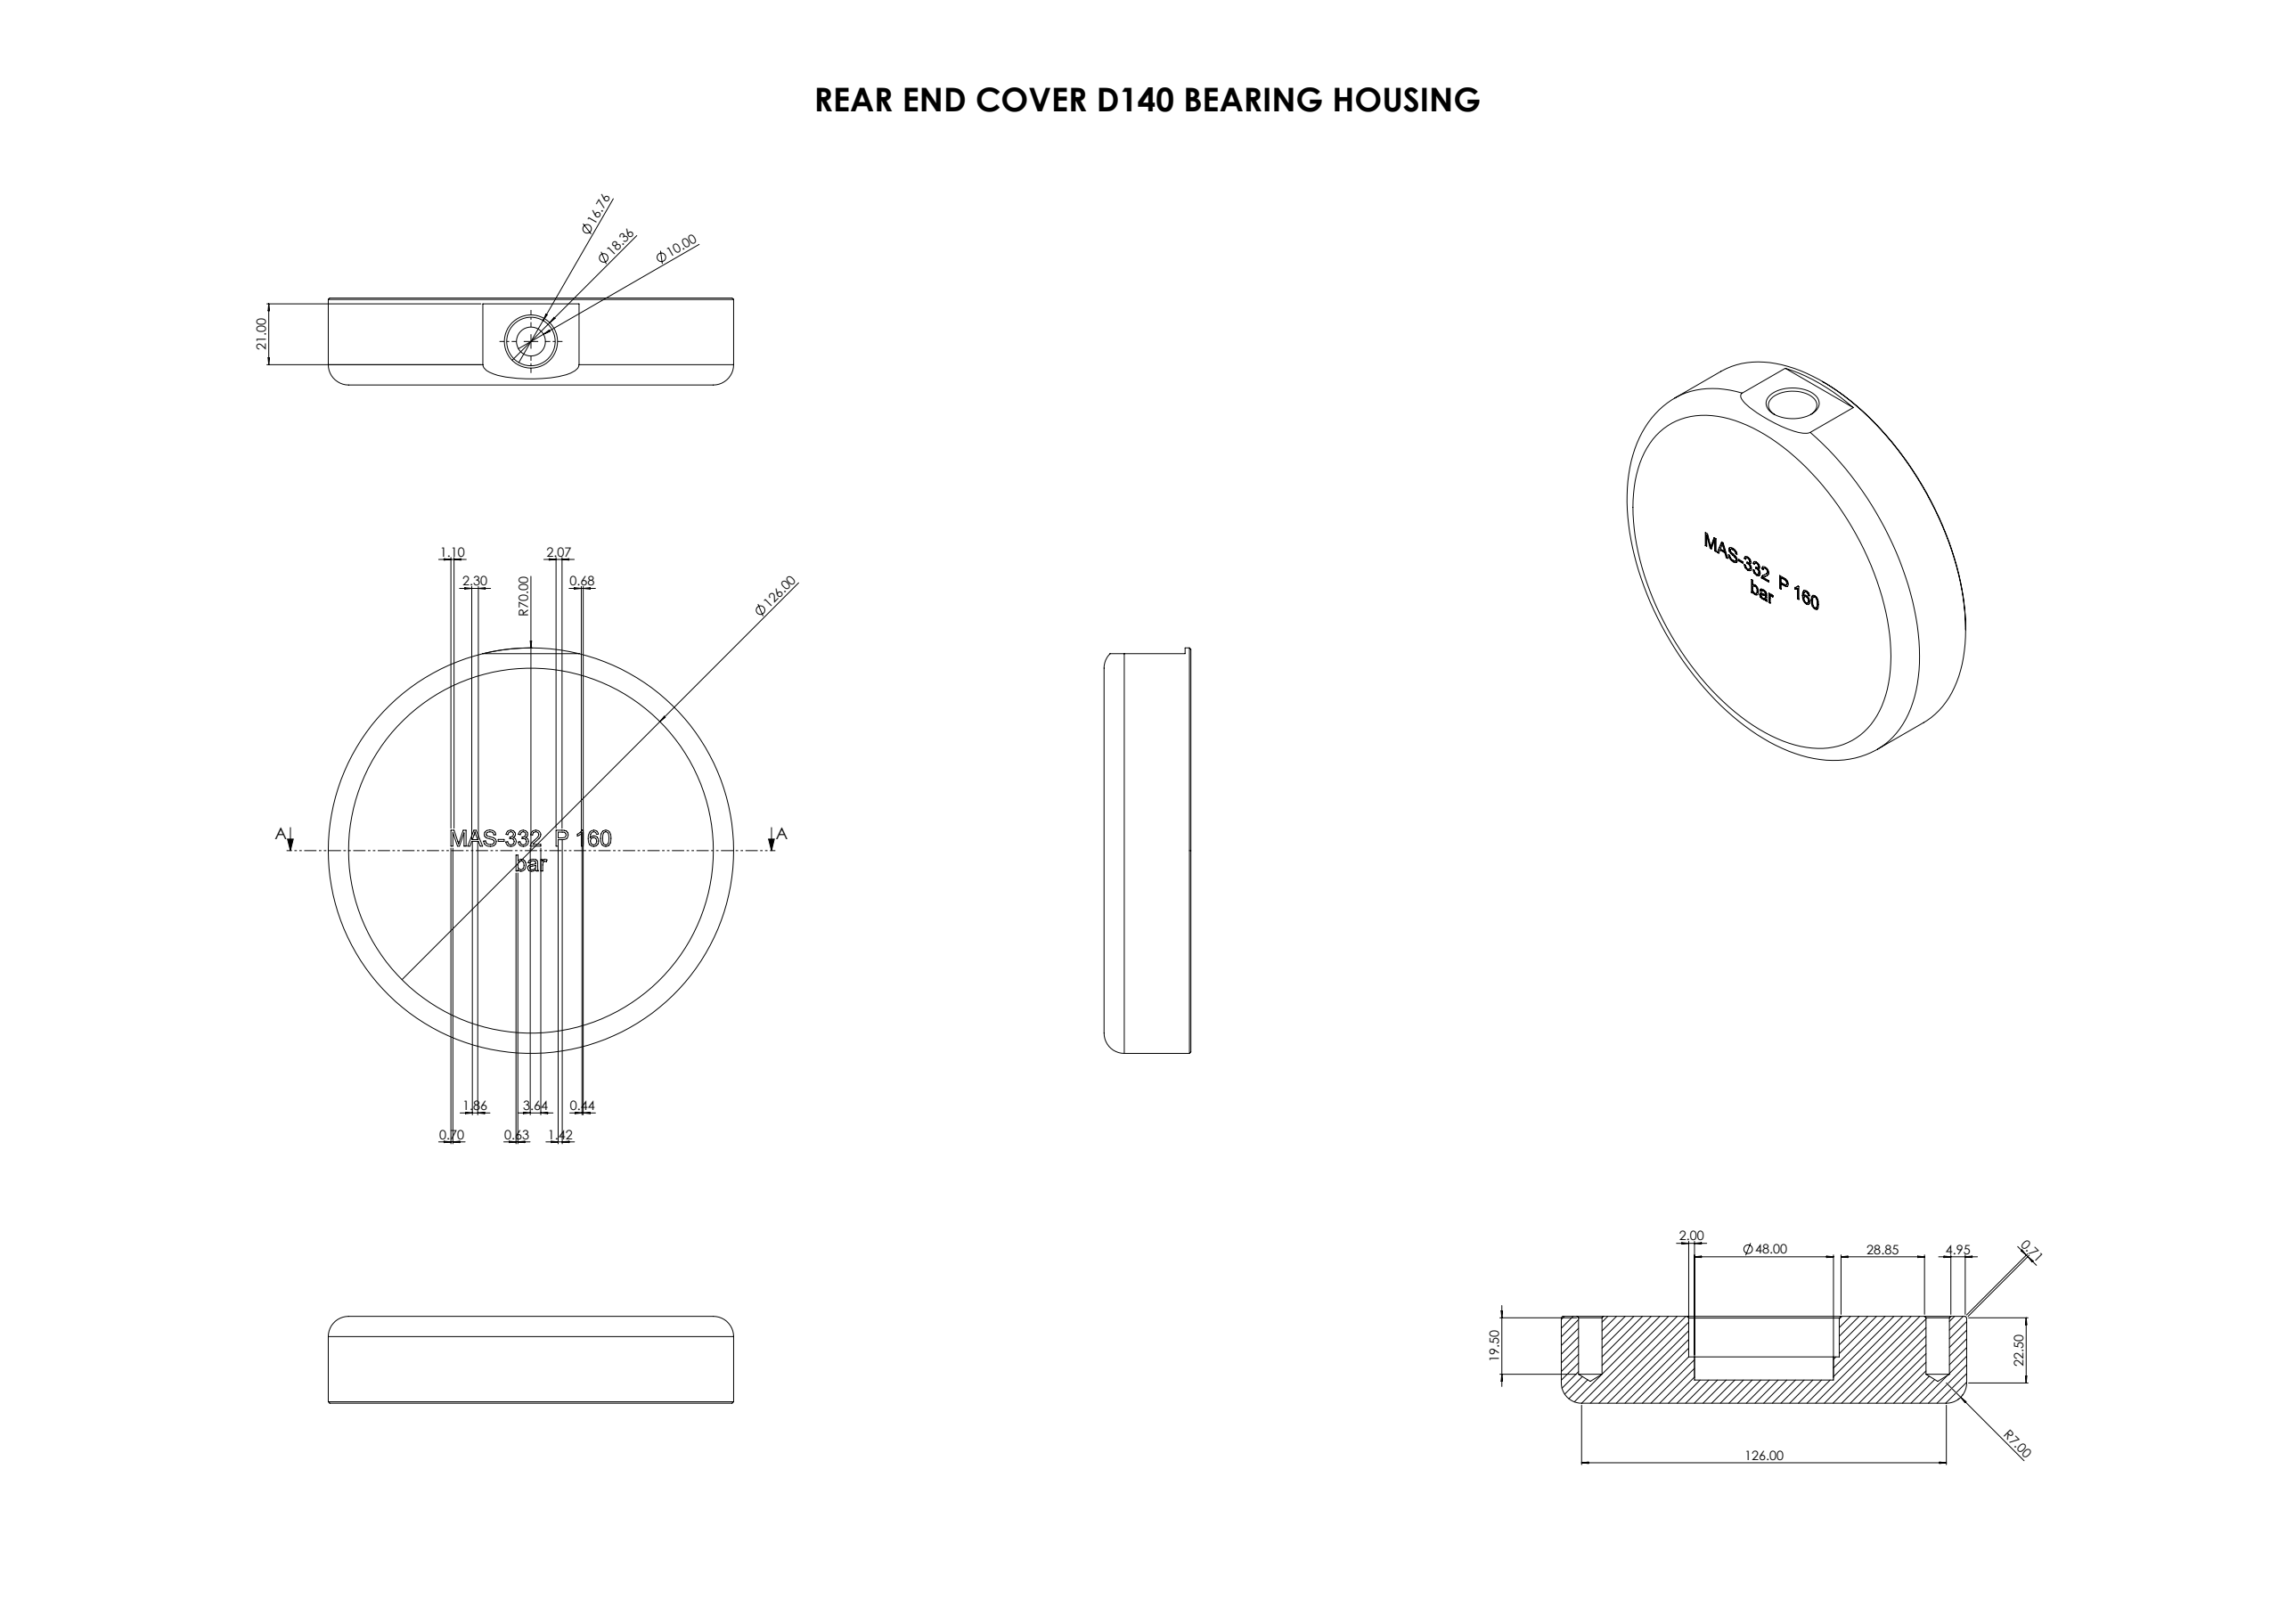
ISO-10303-21;
HEADER;
/* Generated by software containing ST-Developer
 * from STEP Tools, Inc. (www.steptools.com) 
 */

FILE_DESCRIPTION(
/* description */ (''),
/* implementation_level */ '2;1');

FILE_NAME(
/* name */ '03_Rear_End_Cover_D140_Bearing_Housing.step',
/* time_stamp */ '2026-10-23T00:52:27+05:00',
/* author */ (''),
/* organization */ (''),
/* preprocessor_version */ 'ST-DEVELOPER v20.2',
/* originating_system */ 'Autodesk Translation Framework v15.15.0.0',
/* authorisation */ '');

FILE_SCHEMA (('AUTOMOTIVE_DESIGN { 1 0 10303 214 3 1 1 }'));
ENDSEC;

DATA;
#10=MECHANICAL_DESIGN_GEOMETRIC_PRESENTATION_REPRESENTATION('',(#1566,#1567),#59204);
#312=TOROIDAL_SURFACE('',#24105,6.3,0.7);
#332=B_SPLINE_SURFACE_WITH_KNOTS('',2,1,((#43216,#43217),(#43218,#43219),
(#43220,#43221)),.UNSPECIFIED.,.F.,.F.,.F.,(3,3),(2,2),(0.,1.),(0.,0.0300000000000002),
 .UNSPECIFIED.);
#333=B_SPLINE_SURFACE_WITH_KNOTS('',2,1,((#43234,#43235),(#43236,#43237),
(#43238,#43239)),.UNSPECIFIED.,.F.,.F.,.F.,(3,3),(2,2),(0.,1.),(0.,0.0300000000000002),
 .UNSPECIFIED.);
#334=B_SPLINE_SURFACE_WITH_KNOTS('',2,1,((#43249,#43250),(#43251,#43252),
(#43253,#43254)),.UNSPECIFIED.,.F.,.F.,.F.,(3,3),(2,2),(0.,1.),(0.,0.0300000000000002),
 .UNSPECIFIED.);
#335=B_SPLINE_SURFACE_WITH_KNOTS('',2,1,((#43264,#43265),(#43266,#43267),
(#43268,#43269)),.UNSPECIFIED.,.F.,.F.,.F.,(3,3),(2,2),(0.,1.),(0.,0.0300000000000002),
 .UNSPECIFIED.);
#336=B_SPLINE_SURFACE_WITH_KNOTS('',2,1,((#43279,#43280),(#43281,#43282),
(#43283,#43284)),.UNSPECIFIED.,.F.,.F.,.F.,(3,3),(2,2),(0.,1.),(0.,0.0300000000000002),
 .UNSPECIFIED.);
#337=B_SPLINE_SURFACE_WITH_KNOTS('',2,1,((#43294,#43295),(#43296,#43297),
(#43298,#43299)),.UNSPECIFIED.,.F.,.F.,.F.,(3,3),(2,2),(0.,1.),(0.,0.0300000000000002),
 .UNSPECIFIED.);
#338=B_SPLINE_SURFACE_WITH_KNOTS('',2,1,((#43309,#43310),(#43311,#43312),
(#43313,#43314)),.UNSPECIFIED.,.F.,.F.,.F.,(3,3),(2,2),(0.,1.),(0.,0.0300000000000002),
 .UNSPECIFIED.);
#339=B_SPLINE_SURFACE_WITH_KNOTS('',2,1,((#43324,#43325),(#43326,#43327),
(#43328,#43329)),.UNSPECIFIED.,.F.,.F.,.F.,(3,3),(2,2),(0.,1.),(0.,0.0300000000000002),
 .UNSPECIFIED.);
#340=B_SPLINE_SURFACE_WITH_KNOTS('',2,1,((#43339,#43340),(#43341,#43342),
(#43343,#43344)),.UNSPECIFIED.,.F.,.F.,.F.,(3,3),(2,2),(0.,1.),(0.,0.0300000000000002),
 .UNSPECIFIED.);
#341=B_SPLINE_SURFACE_WITH_KNOTS('',2,1,((#43357,#43358),(#43359,#43360),
(#43361,#43362)),.UNSPECIFIED.,.F.,.F.,.F.,(3,3),(2,2),(0.,1.),(0.,0.0300000000000002),
 .UNSPECIFIED.);
#342=B_SPLINE_SURFACE_WITH_KNOTS('',2,1,((#43375,#43376),(#43377,#43378),
(#43379,#43380)),.UNSPECIFIED.,.F.,.F.,.F.,(3,3),(2,2),(0.,1.),(0.,0.0300000000000002),
 .UNSPECIFIED.);
#343=B_SPLINE_SURFACE_WITH_KNOTS('',2,1,((#43396,#43397),(#43398,#43399),
(#43400,#43401)),.UNSPECIFIED.,.F.,.F.,.F.,(3,3),(2,2),(0.,1.),(0.,0.0300000000000002),
 .UNSPECIFIED.);
#344=B_SPLINE_SURFACE_WITH_KNOTS('',2,1,((#43411,#43412),(#43413,#43414),
(#43415,#43416)),.UNSPECIFIED.,.F.,.F.,.F.,(3,3),(2,2),(0.,1.),(0.,0.0300000000000002),
 .UNSPECIFIED.);
#345=B_SPLINE_SURFACE_WITH_KNOTS('',2,1,((#43426,#43427),(#43428,#43429),
(#43430,#43431)),.UNSPECIFIED.,.F.,.F.,.F.,(3,3),(2,2),(0.,1.),(0.,0.0300000000000002),
 .UNSPECIFIED.);
#346=B_SPLINE_SURFACE_WITH_KNOTS('',2,1,((#43441,#43442),(#43443,#43444),
(#43445,#43446)),.UNSPECIFIED.,.F.,.F.,.F.,(3,3),(2,2),(0.,1.),(0.,0.0300000000000002),
 .UNSPECIFIED.);
#347=B_SPLINE_SURFACE_WITH_KNOTS('',2,1,((#43456,#43457),(#43458,#43459),
(#43460,#43461)),.UNSPECIFIED.,.F.,.F.,.F.,(3,3),(2,2),(0.,1.),(0.,0.0300000000000002),
 .UNSPECIFIED.);
#348=B_SPLINE_SURFACE_WITH_KNOTS('',2,1,((#43471,#43472),(#43473,#43474),
(#43475,#43476)),.UNSPECIFIED.,.F.,.F.,.F.,(3,3),(2,2),(0.,1.),(0.,0.0300000000000002),
 .UNSPECIFIED.);
#349=B_SPLINE_SURFACE_WITH_KNOTS('',2,1,((#43486,#43487),(#43488,#43489),
(#43490,#43491)),.UNSPECIFIED.,.F.,.F.,.F.,(3,3),(2,2),(0.,1.),(0.,0.0300000000000002),
 .UNSPECIFIED.);
#350=B_SPLINE_SURFACE_WITH_KNOTS('',2,1,((#43507,#43508),(#43509,#43510),
(#43511,#43512)),.UNSPECIFIED.,.F.,.F.,.F.,(3,3),(2,2),(0.,1.),(0.,0.0300000000000002),
 .UNSPECIFIED.);
#351=B_SPLINE_SURFACE_WITH_KNOTS('',2,1,((#43522,#43523),(#43524,#43525),
(#43526,#43527)),.UNSPECIFIED.,.F.,.F.,.F.,(3,3),(2,2),(0.,1.),(0.,0.0300000000000002),
 .UNSPECIFIED.);
#352=B_SPLINE_SURFACE_WITH_KNOTS('',2,1,((#43537,#43538),(#43539,#43540),
(#43541,#43542)),.UNSPECIFIED.,.F.,.F.,.F.,(3,3),(2,2),(0.,1.),(0.,0.0300000000000002),
 .UNSPECIFIED.);
#353=B_SPLINE_SURFACE_WITH_KNOTS('',2,1,((#43552,#43553),(#43554,#43555),
(#43556,#43557)),.UNSPECIFIED.,.F.,.F.,.F.,(3,3),(2,2),(0.,1.),(0.,0.0300000000000002),
 .UNSPECIFIED.);
#354=B_SPLINE_SURFACE_WITH_KNOTS('',2,1,((#43567,#43568),(#43569,#43570),
(#43571,#43572)),.UNSPECIFIED.,.F.,.F.,.F.,(3,3),(2,2),(0.,1.),(0.,0.0300000000000002),
 .UNSPECIFIED.);
#355=B_SPLINE_SURFACE_WITH_KNOTS('',2,1,((#43582,#43583),(#43584,#43585),
(#43586,#43587)),.UNSPECIFIED.,.F.,.F.,.F.,(3,3),(2,2),(0.,1.),(0.,0.0300000000000002),
 .UNSPECIFIED.);
#356=B_SPLINE_SURFACE_WITH_KNOTS('',2,1,((#43597,#43598),(#43599,#43600),
(#43601,#43602)),.UNSPECIFIED.,.F.,.F.,.F.,(3,3),(2,2),(0.,1.),(0.,0.0300000000000002),
 .UNSPECIFIED.);
#357=B_SPLINE_SURFACE_WITH_KNOTS('',2,1,((#43612,#43613),(#43614,#43615),
(#43616,#43617)),.UNSPECIFIED.,.F.,.F.,.F.,(3,3),(2,2),(0.,1.),(0.,0.0300000000000002),
 .UNSPECIFIED.);
#358=B_SPLINE_SURFACE_WITH_KNOTS('',2,1,((#43627,#43628),(#43629,#43630),
(#43631,#43632)),.UNSPECIFIED.,.F.,.F.,.F.,(3,3),(2,2),(0.,1.),(0.,0.0300000000000002),
 .UNSPECIFIED.);
#359=B_SPLINE_SURFACE_WITH_KNOTS('',2,1,((#43642,#43643),(#43644,#43645),
(#43646,#43647)),.UNSPECIFIED.,.F.,.F.,.F.,(3,3),(2,2),(0.,1.),(0.,0.0300000000000002),
 .UNSPECIFIED.);
#360=B_SPLINE_SURFACE_WITH_KNOTS('',2,1,((#43657,#43658),(#43659,#43660),
(#43661,#43662)),.UNSPECIFIED.,.F.,.F.,.F.,(3,3),(2,2),(0.,1.),(0.,0.0300000000000002),
 .UNSPECIFIED.);
#361=B_SPLINE_SURFACE_WITH_KNOTS('',2,1,((#43672,#43673),(#43674,#43675),
(#43676,#43677)),.UNSPECIFIED.,.F.,.F.,.F.,(3,3),(2,2),(0.,1.),(0.,0.0300000000000002),
 .UNSPECIFIED.);
#362=B_SPLINE_SURFACE_WITH_KNOTS('',2,1,((#43687,#43688),(#43689,#43690),
(#43691,#43692)),.UNSPECIFIED.,.F.,.F.,.F.,(3,3),(2,2),(0.,1.),(0.,0.0300000000000002),
 .UNSPECIFIED.);
#363=B_SPLINE_SURFACE_WITH_KNOTS('',2,1,((#43702,#43703),(#43704,#43705),
(#43706,#43707)),.UNSPECIFIED.,.F.,.F.,.F.,(3,3),(2,2),(0.,1.),(0.,0.0300000000000002),
 .UNSPECIFIED.);
#364=B_SPLINE_SURFACE_WITH_KNOTS('',2,1,((#43717,#43718),(#43719,#43720),
(#43721,#43722)),.UNSPECIFIED.,.F.,.F.,.F.,(3,3),(2,2),(0.,1.),(0.,0.0300000000000002),
 .UNSPECIFIED.);
#365=B_SPLINE_SURFACE_WITH_KNOTS('',2,1,((#43736,#43737),(#43738,#43739),
(#43740,#43741)),.UNSPECIFIED.,.F.,.F.,.F.,(3,3),(2,2),(0.,1.),(0.,0.0300000000000002),
 .UNSPECIFIED.);
#366=B_SPLINE_SURFACE_WITH_KNOTS('',2,1,((#43754,#43755),(#43756,#43757),
(#43758,#43759)),.UNSPECIFIED.,.F.,.F.,.F.,(3,3),(2,2),(0.,1.),(0.,0.0300000000000002),
 .UNSPECIFIED.);
#367=B_SPLINE_SURFACE_WITH_KNOTS('',2,1,((#43769,#43770),(#43771,#43772),
(#43773,#43774)),.UNSPECIFIED.,.F.,.F.,.F.,(3,3),(2,2),(0.,1.),(0.,0.0300000000000002),
 .UNSPECIFIED.);
#368=B_SPLINE_SURFACE_WITH_KNOTS('',2,1,((#43784,#43785),(#43786,#43787),
(#43788,#43789)),.UNSPECIFIED.,.F.,.F.,.F.,(3,3),(2,2),(0.,1.),(0.,0.0300000000000002),
 .UNSPECIFIED.);
#369=B_SPLINE_SURFACE_WITH_KNOTS('',2,1,((#43799,#43800),(#43801,#43802),
(#43803,#43804)),.UNSPECIFIED.,.F.,.F.,.F.,(3,3),(2,2),(0.,1.),(0.,0.0300000000000002),
 .UNSPECIFIED.);
#370=B_SPLINE_SURFACE_WITH_KNOTS('',2,1,((#43814,#43815),(#43816,#43817),
(#43818,#43819)),.UNSPECIFIED.,.F.,.F.,.F.,(3,3),(2,2),(0.,1.),(0.,0.0300000000000002),
 .UNSPECIFIED.);
#371=B_SPLINE_SURFACE_WITH_KNOTS('',2,1,((#43829,#43830),(#43831,#43832),
(#43833,#43834)),.UNSPECIFIED.,.F.,.F.,.F.,(3,3),(2,2),(0.,1.),(0.,0.0300000000000002),
 .UNSPECIFIED.);
#372=B_SPLINE_SURFACE_WITH_KNOTS('',2,1,((#43844,#43845),(#43846,#43847),
(#43848,#43849)),.UNSPECIFIED.,.F.,.F.,.F.,(3,3),(2,2),(0.,1.),(0.,0.0300000000000002),
 .UNSPECIFIED.);
#373=B_SPLINE_SURFACE_WITH_KNOTS('',2,1,((#43856,#43857),(#43858,#43859),
(#43860,#43861)),.UNSPECIFIED.,.F.,.F.,.F.,(3,3),(2,2),(0.,1.),(0.,0.0300000000000002),
 .UNSPECIFIED.);
#374=B_SPLINE_SURFACE_WITH_KNOTS('',2,1,((#43874,#43875),(#43876,#43877),
(#43878,#43879)),.UNSPECIFIED.,.F.,.F.,.F.,(3,3),(2,2),(0.,1.),(0.,0.0300000000000002),
 .UNSPECIFIED.);
#375=B_SPLINE_SURFACE_WITH_KNOTS('',2,1,((#43889,#43890),(#43891,#43892),
(#43893,#43894)),.UNSPECIFIED.,.F.,.F.,.F.,(3,3),(2,2),(0.,1.),(0.,0.0300000000000002),
 .UNSPECIFIED.);
#376=B_SPLINE_SURFACE_WITH_KNOTS('',2,1,((#43904,#43905),(#43906,#43907),
(#43908,#43909)),.UNSPECIFIED.,.F.,.F.,.F.,(3,3),(2,2),(0.,1.),(0.,0.0300000000000002),
 .UNSPECIFIED.);
#377=B_SPLINE_SURFACE_WITH_KNOTS('',2,1,((#43919,#43920),(#43921,#43922),
(#43923,#43924)),.UNSPECIFIED.,.F.,.F.,.F.,(3,3),(2,2),(0.,1.),(0.,0.0300000000000002),
 .UNSPECIFIED.);
#378=B_SPLINE_SURFACE_WITH_KNOTS('',2,1,((#43934,#43935),(#43936,#43937),
(#43938,#43939)),.UNSPECIFIED.,.F.,.F.,.F.,(3,3),(2,2),(0.,1.),(0.,0.0300000000000002),
 .UNSPECIFIED.);
#379=B_SPLINE_SURFACE_WITH_KNOTS('',2,1,((#43949,#43950),(#43951,#43952),
(#43953,#43954)),.UNSPECIFIED.,.F.,.F.,.F.,(3,3),(2,2),(0.,1.),(0.,0.0300000000000002),
 .UNSPECIFIED.);
#380=B_SPLINE_SURFACE_WITH_KNOTS('',2,1,((#43964,#43965),(#43966,#43967),
(#43968,#43969)),.UNSPECIFIED.,.F.,.F.,.F.,(3,3),(2,2),(0.,1.),(0.,0.0300000000000002),
 .UNSPECIFIED.);
#381=B_SPLINE_SURFACE_WITH_KNOTS('',2,1,((#43979,#43980),(#43981,#43982),
(#43983,#43984)),.UNSPECIFIED.,.F.,.F.,.F.,(3,3),(2,2),(0.,1.),(0.,0.0300000000000002),
 .UNSPECIFIED.);
#382=B_SPLINE_SURFACE_WITH_KNOTS('',2,1,((#43994,#43995),(#43996,#43997),
(#43998,#43999)),.UNSPECIFIED.,.F.,.F.,.F.,(3,3),(2,2),(0.,1.),(0.,0.0300000000000002),
 .UNSPECIFIED.);
#383=B_SPLINE_SURFACE_WITH_KNOTS('',2,1,((#44009,#44010),(#44011,#44012),
(#44013,#44014)),.UNSPECIFIED.,.F.,.F.,.F.,(3,3),(2,2),(0.,1.),(0.,0.0300000000000002),
 .UNSPECIFIED.);
#384=B_SPLINE_SURFACE_WITH_KNOTS('',2,1,((#44024,#44025),(#44026,#44027),
(#44028,#44029)),.UNSPECIFIED.,.F.,.F.,.F.,(3,3),(2,2),(0.,1.),(0.,0.0300000000000002),
 .UNSPECIFIED.);
#385=B_SPLINE_SURFACE_WITH_KNOTS('',2,1,((#44037,#44038),(#44039,#44040),
(#44041,#44042)),.UNSPECIFIED.,.F.,.F.,.F.,(3,3),(2,2),(0.,1.),(0.,0.0300000000000002),
 .UNSPECIFIED.);
#386=B_SPLINE_SURFACE_WITH_KNOTS('',2,1,((#44055,#44056),(#44057,#44058),
(#44059,#44060)),.UNSPECIFIED.,.F.,.F.,.F.,(3,3),(2,2),(0.,1.),(0.,0.0300000000000002),
 .UNSPECIFIED.);
#387=B_SPLINE_SURFACE_WITH_KNOTS('',2,1,((#44076,#44077),(#44078,#44079),
(#44080,#44081)),.UNSPECIFIED.,.F.,.F.,.F.,(3,3),(2,2),(0.,1.),(0.,0.0300000000000002),
 .UNSPECIFIED.);
#388=B_SPLINE_SURFACE_WITH_KNOTS('',2,1,((#44091,#44092),(#44093,#44094),
(#44095,#44096)),.UNSPECIFIED.,.F.,.F.,.F.,(3,3),(2,2),(0.,1.),(0.,0.0300000000000002),
 .UNSPECIFIED.);
#389=B_SPLINE_SURFACE_WITH_KNOTS('',2,1,((#44179,#44180),(#44181,#44182),
(#44183,#44184)),.UNSPECIFIED.,.F.,.F.,.F.,(3,3),(2,2),(0.,1.),(0.,0.0300000000000002),
 .UNSPECIFIED.);
#390=B_SPLINE_SURFACE_WITH_KNOTS('',2,1,((#44194,#44195),(#44196,#44197),
(#44198,#44199)),.UNSPECIFIED.,.F.,.F.,.F.,(3,3),(2,2),(0.,1.),(0.,0.0300000000000002),
 .UNSPECIFIED.);
#391=B_SPLINE_SURFACE_WITH_KNOTS('',2,1,((#44237,#44238),(#44239,#44240),
(#44241,#44242)),.UNSPECIFIED.,.F.,.F.,.F.,(3,3),(2,2),(0.,1.),(0.,0.0300000000000002),
 .UNSPECIFIED.);
#392=B_SPLINE_SURFACE_WITH_KNOTS('',2,1,((#44255,#44256),(#44257,#44258),
(#44259,#44260)),.UNSPECIFIED.,.F.,.F.,.F.,(3,3),(2,2),(0.,1.),(0.,0.0300000000000002),
 .UNSPECIFIED.);
#393=B_SPLINE_SURFACE_WITH_KNOTS('',2,1,((#44270,#44271),(#44272,#44273),
(#44274,#44275)),.UNSPECIFIED.,.F.,.F.,.F.,(3,3),(2,2),(0.,1.),(0.,0.0300000000000002),
 .UNSPECIFIED.);
#394=B_SPLINE_SURFACE_WITH_KNOTS('',2,1,((#44285,#44286),(#44287,#44288),
(#44289,#44290)),.UNSPECIFIED.,.F.,.F.,.F.,(3,3),(2,2),(0.,1.),(0.,0.0300000000000002),
 .UNSPECIFIED.);
#395=B_SPLINE_SURFACE_WITH_KNOTS('',2,1,((#44300,#44301),(#44302,#44303),
(#44304,#44305)),.UNSPECIFIED.,.F.,.F.,.F.,(3,3),(2,2),(0.,1.),(0.,0.0300000000000002),
 .UNSPECIFIED.);
#396=B_SPLINE_SURFACE_WITH_KNOTS('',2,1,((#44315,#44316),(#44317,#44318),
(#44319,#44320)),.UNSPECIFIED.,.F.,.F.,.F.,(3,3),(2,2),(0.,1.),(0.,0.0300000000000002),
 .UNSPECIFIED.);
#397=B_SPLINE_SURFACE_WITH_KNOTS('',2,1,((#44330,#44331),(#44332,#44333),
(#44334,#44335)),.UNSPECIFIED.,.F.,.F.,.F.,(3,3),(2,2),(0.,1.),(0.,0.0300000000000002),
 .UNSPECIFIED.);
#398=B_SPLINE_SURFACE_WITH_KNOTS('',2,1,((#44345,#44346),(#44347,#44348),
(#44349,#44350)),.UNSPECIFIED.,.F.,.F.,.F.,(3,3),(2,2),(0.,1.),(0.,0.0300000000000002),
 .UNSPECIFIED.);
#399=B_SPLINE_SURFACE_WITH_KNOTS('',2,1,((#44360,#44361),(#44362,#44363),
(#44364,#44365)),.UNSPECIFIED.,.F.,.F.,.F.,(3,3),(2,2),(0.,1.),(0.,0.0300000000000002),
 .UNSPECIFIED.);
#400=B_SPLINE_SURFACE_WITH_KNOTS('',2,1,((#44375,#44376),(#44377,#44378),
(#44379,#44380)),.UNSPECIFIED.,.F.,.F.,.F.,(3,3),(2,2),(0.,1.),(0.,0.0300000000000002),
 .UNSPECIFIED.);
#401=B_SPLINE_SURFACE_WITH_KNOTS('',2,1,((#44390,#44391),(#44392,#44393),
(#44394,#44395)),.UNSPECIFIED.,.F.,.F.,.F.,(3,3),(2,2),(0.,1.),(0.,0.0300000000000002),
 .UNSPECIFIED.);
#402=B_SPLINE_SURFACE_WITH_KNOTS('',2,1,((#44411,#44412),(#44413,#44414),
(#44415,#44416)),.UNSPECIFIED.,.F.,.F.,.F.,(3,3),(2,2),(0.,1.),(0.,0.0300000000000002),
 .UNSPECIFIED.);
#403=B_SPLINE_SURFACE_WITH_KNOTS('',2,1,((#44426,#44427),(#44428,#44429),
(#44430,#44431)),.UNSPECIFIED.,.F.,.F.,.F.,(3,3),(2,2),(0.,1.),(0.,0.0300000000000002),
 .UNSPECIFIED.);
#404=B_SPLINE_SURFACE_WITH_KNOTS('',2,1,((#44441,#44442),(#44443,#44444),
(#44445,#44446)),.UNSPECIFIED.,.F.,.F.,.F.,(3,3),(2,2),(0.,1.),(0.,0.0300000000000002),
 .UNSPECIFIED.);
#405=B_SPLINE_SURFACE_WITH_KNOTS('',2,1,((#44456,#44457),(#44458,#44459),
(#44460,#44461)),.UNSPECIFIED.,.F.,.F.,.F.,(3,3),(2,2),(0.,1.),(0.,0.0300000000000002),
 .UNSPECIFIED.);
#406=B_SPLINE_SURFACE_WITH_KNOTS('',2,1,((#44471,#44472),(#44473,#44474),
(#44475,#44476)),.UNSPECIFIED.,.F.,.F.,.F.,(3,3),(2,2),(0.,1.),(0.,0.0300000000000002),
 .UNSPECIFIED.);
#407=B_SPLINE_SURFACE_WITH_KNOTS('',2,1,((#44486,#44487),(#44488,#44489),
(#44490,#44491)),.UNSPECIFIED.,.F.,.F.,.F.,(3,3),(2,2),(0.,1.),(0.,0.0300000000000002),
 .UNSPECIFIED.);
#408=B_SPLINE_SURFACE_WITH_KNOTS('',2,1,((#44501,#44502),(#44503,#44504),
(#44505,#44506)),.UNSPECIFIED.,.F.,.F.,.F.,(3,3),(2,2),(0.,1.),(0.,0.0300000000000002),
 .UNSPECIFIED.);
#409=B_SPLINE_SURFACE_WITH_KNOTS('',2,1,((#44522,#44523),(#44524,#44525),
(#44526,#44527)),.UNSPECIFIED.,.F.,.F.,.F.,(3,3),(2,2),(0.,1.),(0.,0.0300000000000002),
 .UNSPECIFIED.);
#410=B_SPLINE_SURFACE_WITH_KNOTS('',2,1,((#44537,#44538),(#44539,#44540),
(#44541,#44542)),.UNSPECIFIED.,.F.,.F.,.F.,(3,3),(2,2),(0.,1.),(0.,0.0300000000000002),
 .UNSPECIFIED.);
#411=B_SPLINE_SURFACE_WITH_KNOTS('',2,1,((#44552,#44553),(#44554,#44555),
(#44556,#44557)),.UNSPECIFIED.,.F.,.F.,.F.,(3,3),(2,2),(0.,1.),(0.,0.0300000000000002),
 .UNSPECIFIED.);
#412=B_SPLINE_SURFACE_WITH_KNOTS('',2,1,((#44567,#44568),(#44569,#44570),
(#44571,#44572)),.UNSPECIFIED.,.F.,.F.,.F.,(3,3),(2,2),(0.,1.),(0.,0.0300000000000002),
 .UNSPECIFIED.);
#413=B_SPLINE_SURFACE_WITH_KNOTS('',2,1,((#44582,#44583),(#44584,#44585),
(#44586,#44587)),.UNSPECIFIED.,.F.,.F.,.F.,(3,3),(2,2),(0.,1.),(0.,0.0300000000000002),
 .UNSPECIFIED.);
#414=B_SPLINE_SURFACE_WITH_KNOTS('',2,1,((#44597,#44598),(#44599,#44600),
(#44601,#44602)),.UNSPECIFIED.,.F.,.F.,.F.,(3,3),(2,2),(0.,1.),(0.,0.0300000000000002),
 .UNSPECIFIED.);
#415=B_SPLINE_SURFACE_WITH_KNOTS('',2,1,((#44612,#44613),(#44614,#44615),
(#44616,#44617)),.UNSPECIFIED.,.F.,.F.,.F.,(3,3),(2,2),(0.,1.),(0.,0.0300000000000002),
 .UNSPECIFIED.);
#416=B_SPLINE_SURFACE_WITH_KNOTS('',2,1,((#44633,#44634),(#44635,#44636),
(#44637,#44638)),.UNSPECIFIED.,.F.,.F.,.F.,(3,3),(2,2),(0.,1.),(0.,0.0300000000000002),
 .UNSPECIFIED.);
#417=B_SPLINE_SURFACE_WITH_KNOTS('',2,1,((#44648,#44649),(#44650,#44651),
(#44652,#44653)),.UNSPECIFIED.,.F.,.F.,.F.,(3,3),(2,2),(0.,1.),(0.,0.0300000000000002),
 .UNSPECIFIED.);
#418=B_SPLINE_SURFACE_WITH_KNOTS('',2,1,((#44686,#44687),(#44688,#44689),
(#44690,#44691)),.UNSPECIFIED.,.F.,.F.,.F.,(3,3),(2,2),(0.,1.),(0.,0.0300000000000002),
 .UNSPECIFIED.);
#419=B_SPLINE_SURFACE_WITH_KNOTS('',2,1,((#44704,#44705),(#44706,#44707),
(#44708,#44709)),.UNSPECIFIED.,.F.,.F.,.F.,(3,3),(2,2),(0.,1.),(0.,0.0300000000000002),
 .UNSPECIFIED.);
#420=B_SPLINE_SURFACE_WITH_KNOTS('',2,1,((#44783,#44784),(#44785,#44786),
(#44787,#44788)),.UNSPECIFIED.,.F.,.F.,.F.,(3,3),(2,2),(0.,1.),(0.,0.0300000000000002),
 .UNSPECIFIED.);
#421=B_SPLINE_SURFACE_WITH_KNOTS('',2,1,((#44801,#44802),(#44803,#44804),
(#44805,#44806)),.UNSPECIFIED.,.F.,.F.,.F.,(3,3),(2,2),(0.,1.),(0.,0.0300000000000002),
 .UNSPECIFIED.);
#422=B_SPLINE_SURFACE_WITH_KNOTS('',2,1,((#44816,#44817),(#44818,#44819),
(#44820,#44821)),.UNSPECIFIED.,.F.,.F.,.F.,(3,3),(2,2),(0.,1.),(0.,0.0300000000000002),
 .UNSPECIFIED.);
#423=B_SPLINE_SURFACE_WITH_KNOTS('',2,1,((#44831,#44832),(#44833,#44834),
(#44835,#44836)),.UNSPECIFIED.,.F.,.F.,.F.,(3,3),(2,2),(0.,1.),(0.,0.0300000000000002),
 .UNSPECIFIED.);
#424=B_SPLINE_SURFACE_WITH_KNOTS('',2,1,((#44846,#44847),(#44848,#44849),
(#44850,#44851)),.UNSPECIFIED.,.F.,.F.,.F.,(3,3),(2,2),(0.,1.),(0.,0.0300000000000002),
 .UNSPECIFIED.);
#425=B_SPLINE_SURFACE_WITH_KNOTS('',2,1,((#44861,#44862),(#44863,#44864),
(#44865,#44866)),.UNSPECIFIED.,.F.,.F.,.F.,(3,3),(2,2),(0.,1.),(0.,0.0300000000000002),
 .UNSPECIFIED.);
#426=B_SPLINE_SURFACE_WITH_KNOTS('',2,1,((#44876,#44877),(#44878,#44879),
(#44880,#44881)),.UNSPECIFIED.,.F.,.F.,.F.,(3,3),(2,2),(0.,1.),(0.,0.0300000000000002),
 .UNSPECIFIED.);
#427=B_SPLINE_SURFACE_WITH_KNOTS('',2,1,((#44891,#44892),(#44893,#44894),
(#44895,#44896)),.UNSPECIFIED.,.F.,.F.,.F.,(3,3),(2,2),(0.,1.),(0.,0.0300000000000002),
 .UNSPECIFIED.);
#428=B_SPLINE_SURFACE_WITH_KNOTS('',2,1,((#44906,#44907),(#44908,#44909),
(#44910,#44911)),.UNSPECIFIED.,.F.,.F.,.F.,(3,3),(2,2),(0.,1.),(0.,0.0300000000000002),
 .UNSPECIFIED.);
#429=B_SPLINE_SURFACE_WITH_KNOTS('',2,1,((#44921,#44922),(#44923,#44924),
(#44925,#44926)),.UNSPECIFIED.,.F.,.F.,.F.,(3,3),(2,2),(0.,1.),(0.,0.0300000000000002),
 .UNSPECIFIED.);
#430=B_SPLINE_SURFACE_WITH_KNOTS('',2,1,((#44936,#44937),(#44938,#44939),
(#44940,#44941)),.UNSPECIFIED.,.F.,.F.,.F.,(3,3),(2,2),(0.,1.),(0.,0.0300000000000002),
 .UNSPECIFIED.);
#431=B_SPLINE_SURFACE_WITH_KNOTS('',2,1,((#44951,#44952),(#44953,#44954),
(#44955,#44956)),.UNSPECIFIED.,.F.,.F.,.F.,(3,3),(2,2),(0.,1.),(0.,0.0300000000000002),
 .UNSPECIFIED.);
#432=B_SPLINE_SURFACE_WITH_KNOTS('',2,1,((#44966,#44967),(#44968,#44969),
(#44970,#44971)),.UNSPECIFIED.,.F.,.F.,.F.,(3,3),(2,2),(0.,1.),(0.,0.0300000000000002),
 .UNSPECIFIED.);
#433=B_SPLINE_SURFACE_WITH_KNOTS('',2,1,((#44987,#44988),(#44989,#44990),
(#44991,#44992)),.UNSPECIFIED.,.F.,.F.,.F.,(3,3),(2,2),(0.,1.),(0.,0.0300000000000002),
 .UNSPECIFIED.);
#434=B_SPLINE_SURFACE_WITH_KNOTS('',2,1,((#45002,#45003),(#45004,#45005),
(#45006,#45007)),.UNSPECIFIED.,.F.,.F.,.F.,(3,3),(2,2),(0.,1.),(0.,0.0300000000000002),
 .UNSPECIFIED.);
#435=B_SPLINE_SURFACE_WITH_KNOTS('',2,1,((#45017,#45018),(#45019,#45020),
(#45021,#45022)),.UNSPECIFIED.,.F.,.F.,.F.,(3,3),(2,2),(0.,1.),(0.,0.0300000000000002),
 .UNSPECIFIED.);
#436=B_SPLINE_SURFACE_WITH_KNOTS('',2,1,((#45032,#45033),(#45034,#45035),
(#45036,#45037)),.UNSPECIFIED.,.F.,.F.,.F.,(3,3),(2,2),(0.,1.),(0.,0.0300000000000002),
 .UNSPECIFIED.);
#437=B_SPLINE_SURFACE_WITH_KNOTS('',2,1,((#45047,#45048),(#45049,#45050),
(#45051,#45052)),.UNSPECIFIED.,.F.,.F.,.F.,(3,3),(2,2),(0.,1.),(0.,0.0300000000000002),
 .UNSPECIFIED.);
#438=B_SPLINE_SURFACE_WITH_KNOTS('',2,1,((#45062,#45063),(#45064,#45065),
(#45066,#45067)),.UNSPECIFIED.,.F.,.F.,.F.,(3,3),(2,2),(0.,1.),(0.,0.0300000000000002),
 .UNSPECIFIED.);
#439=B_SPLINE_SURFACE_WITH_KNOTS('',2,1,((#45077,#45078),(#45079,#45080),
(#45081,#45082)),.UNSPECIFIED.,.F.,.F.,.F.,(3,3),(2,2),(0.,1.),(0.,0.0300000000000002),
 .UNSPECIFIED.);
#440=B_SPLINE_SURFACE_WITH_KNOTS('',2,1,((#45092,#45093),(#45094,#45095),
(#45096,#45097)),.UNSPECIFIED.,.F.,.F.,.F.,(3,3),(2,2),(0.,1.),(0.,0.0300000000000002),
 .UNSPECIFIED.);
#441=B_SPLINE_SURFACE_WITH_KNOTS('',2,1,((#45107,#45108),(#45109,#45110),
(#45111,#45112)),.UNSPECIFIED.,.F.,.F.,.F.,(3,3),(2,2),(0.,1.),(0.,0.0300000000000002),
 .UNSPECIFIED.);
#442=B_SPLINE_SURFACE_WITH_KNOTS('',2,1,((#45122,#45123),(#45124,#45125),
(#45126,#45127)),.UNSPECIFIED.,.F.,.F.,.F.,(3,3),(2,2),(0.,1.),(0.,0.0300000000000002),
 .UNSPECIFIED.);
#443=B_SPLINE_SURFACE_WITH_KNOTS('',2,1,((#45137,#45138),(#45139,#45140),
(#45141,#45142)),.UNSPECIFIED.,.F.,.F.,.F.,(3,3),(2,2),(0.,1.),(0.,0.0300000000000002),
 .UNSPECIFIED.);
#444=B_SPLINE_SURFACE_WITH_KNOTS('',2,1,((#45152,#45153),(#45154,#45155),
(#45156,#45157)),.UNSPECIFIED.,.F.,.F.,.F.,(3,3),(2,2),(0.,1.),(0.,0.0300000000000002),
 .UNSPECIFIED.);
#445=B_SPLINE_SURFACE_WITH_KNOTS('',2,1,((#45167,#45168),(#45169,#45170),
(#45171,#45172)),.UNSPECIFIED.,.F.,.F.,.F.,(3,3),(2,2),(0.,1.),(0.,0.0300000000000002),
 .UNSPECIFIED.);
#446=B_SPLINE_SURFACE_WITH_KNOTS('',2,1,((#45182,#45183),(#45184,#45185),
(#45186,#45187)),.UNSPECIFIED.,.F.,.F.,.F.,(3,3),(2,2),(0.,1.),(0.,0.0300000000000002),
 .UNSPECIFIED.);
#447=B_SPLINE_SURFACE_WITH_KNOTS('',2,1,((#45197,#45198),(#45199,#45200),
(#45201,#45202)),.UNSPECIFIED.,.F.,.F.,.F.,(3,3),(2,2),(0.,1.),(0.,0.0300000000000002),
 .UNSPECIFIED.);
#448=B_SPLINE_SURFACE_WITH_KNOTS('',2,1,((#45212,#45213),(#45214,#45215),
(#45216,#45217)),.UNSPECIFIED.,.F.,.F.,.F.,(3,3),(2,2),(0.,1.),(0.,0.0300000000000002),
 .UNSPECIFIED.);
#449=B_SPLINE_SURFACE_WITH_KNOTS('',2,1,((#45227,#45228),(#45229,#45230),
(#45231,#45232)),.UNSPECIFIED.,.F.,.F.,.F.,(3,3),(2,2),(0.,1.),(0.,0.0300000000000002),
 .UNSPECIFIED.);
#450=B_SPLINE_SURFACE_WITH_KNOTS('',2,1,((#45242,#45243),(#45244,#45245),
(#45246,#45247)),.UNSPECIFIED.,.F.,.F.,.F.,(3,3),(2,2),(0.,1.),(0.,0.0300000000000002),
 .UNSPECIFIED.);
#451=B_SPLINE_SURFACE_WITH_KNOTS('',2,1,((#45263,#45264),(#45265,#45266),
(#45267,#45268)),.UNSPECIFIED.,.F.,.F.,.F.,(3,3),(2,2),(0.,1.),(0.,0.0300000000000002),
 .UNSPECIFIED.);
#452=B_SPLINE_SURFACE_WITH_KNOTS('',2,1,((#45278,#45279),(#45280,#45281),
(#45282,#45283)),.UNSPECIFIED.,.F.,.F.,.F.,(3,3),(2,2),(0.,1.),(0.,0.0300000000000002),
 .UNSPECIFIED.);
#453=B_SPLINE_SURFACE_WITH_KNOTS('',2,1,((#45291,#45292),(#45293,#45294),
(#45295,#45296)),.UNSPECIFIED.,.F.,.F.,.F.,(3,3),(2,2),(0.,1.),(0.,0.0300000000000002),
 .UNSPECIFIED.);
#454=B_SPLINE_SURFACE_WITH_KNOTS('',2,1,((#45309,#45310),(#45311,#45312),
(#45313,#45314)),.UNSPECIFIED.,.F.,.F.,.F.,(3,3),(2,2),(0.,1.),(0.,0.0300000000000002),
 .UNSPECIFIED.);
#455=B_SPLINE_SURFACE_WITH_KNOTS('',2,1,((#45324,#45325),(#45326,#45327),
(#45328,#45329)),.UNSPECIFIED.,.F.,.F.,.F.,(3,3),(2,2),(0.,1.),(0.,0.0300000000000002),
 .UNSPECIFIED.);
#456=B_SPLINE_SURFACE_WITH_KNOTS('',2,1,((#45339,#45340),(#45341,#45342),
(#45343,#45344)),.UNSPECIFIED.,.F.,.F.,.F.,(3,3),(2,2),(0.,1.),(0.,0.0300000000000002),
 .UNSPECIFIED.);
#457=B_SPLINE_SURFACE_WITH_KNOTS('',2,1,((#45354,#45355),(#45356,#45357),
(#45358,#45359)),.UNSPECIFIED.,.F.,.F.,.F.,(3,3),(2,2),(0.,1.),(0.,0.0300000000000002),
 .UNSPECIFIED.);
#458=B_SPLINE_SURFACE_WITH_KNOTS('',2,1,((#45369,#45370),(#45371,#45372),
(#45373,#45374)),.UNSPECIFIED.,.F.,.F.,.F.,(3,3),(2,2),(0.,1.),(0.,0.0300000000000002),
 .UNSPECIFIED.);
#459=B_SPLINE_SURFACE_WITH_KNOTS('',2,1,((#45384,#45385),(#45386,#45387),
(#45388,#45389)),.UNSPECIFIED.,.F.,.F.,.F.,(3,3),(2,2),(0.,1.),(0.,0.0300000000000002),
 .UNSPECIFIED.);
#460=B_SPLINE_SURFACE_WITH_KNOTS('',2,1,((#45399,#45400),(#45401,#45402),
(#45403,#45404)),.UNSPECIFIED.,.F.,.F.,.F.,(3,3),(2,2),(0.,1.),(0.,0.0300000000000002),
 .UNSPECIFIED.);
#461=B_SPLINE_SURFACE_WITH_KNOTS('',2,1,((#45414,#45415),(#45416,#45417),
(#45418,#45419)),.UNSPECIFIED.,.F.,.F.,.F.,(3,3),(2,2),(0.,1.),(0.,0.0300000000000002),
 .UNSPECIFIED.);
#462=B_SPLINE_SURFACE_WITH_KNOTS('',2,1,((#45429,#45430),(#45431,#45432),
(#45433,#45434)),.UNSPECIFIED.,.F.,.F.,.F.,(3,3),(2,2),(0.,1.),(0.,0.0300000000000002),
 .UNSPECIFIED.);
#463=B_SPLINE_SURFACE_WITH_KNOTS('',2,1,((#45444,#45445),(#45446,#45447),
(#45448,#45449)),.UNSPECIFIED.,.F.,.F.,.F.,(3,3),(2,2),(0.,1.),(0.,0.0300000000000002),
 .UNSPECIFIED.);
#464=B_SPLINE_SURFACE_WITH_KNOTS('',2,1,((#45465,#45466),(#45467,#45468),
(#45469,#45470)),.UNSPECIFIED.,.F.,.F.,.F.,(3,3),(2,2),(0.,1.),(0.,0.0300000000000002),
 .UNSPECIFIED.);
#465=B_SPLINE_SURFACE_WITH_KNOTS('',2,1,((#45480,#45481),(#45482,#45483),
(#45484,#45485)),.UNSPECIFIED.,.F.,.F.,.F.,(3,3),(2,2),(0.,1.),(0.,0.0300000000000002),
 .UNSPECIFIED.);
#466=B_SPLINE_SURFACE_WITH_KNOTS('',2,1,((#45495,#45496),(#45497,#45498),
(#45499,#45500)),.UNSPECIFIED.,.F.,.F.,.F.,(3,3),(2,2),(0.,1.),(0.,0.0300000000000002),
 .UNSPECIFIED.);
#467=B_SPLINE_SURFACE_WITH_KNOTS('',2,1,((#45510,#45511),(#45512,#45513),
(#45514,#45515)),.UNSPECIFIED.,.F.,.F.,.F.,(3,3),(2,2),(0.,1.),(0.,0.0300000000000002),
 .UNSPECIFIED.);
#468=B_SPLINE_SURFACE_WITH_KNOTS('',2,1,((#45525,#45526),(#45527,#45528),
(#45529,#45530)),.UNSPECIFIED.,.F.,.F.,.F.,(3,3),(2,2),(0.,1.),(0.,0.0300000000000002),
 .UNSPECIFIED.);
#469=B_SPLINE_SURFACE_WITH_KNOTS('',2,1,((#45540,#45541),(#45542,#45543),
(#45544,#45545)),.UNSPECIFIED.,.F.,.F.,.F.,(3,3),(2,2),(0.,1.),(0.,0.0300000000000002),
 .UNSPECIFIED.);
#470=B_SPLINE_SURFACE_WITH_KNOTS('',2,1,((#45555,#45556),(#45557,#45558),
(#45559,#45560)),.UNSPECIFIED.,.F.,.F.,.F.,(3,3),(2,2),(0.,1.),(0.,0.0300000000000002),
 .UNSPECIFIED.);
#471=B_SPLINE_SURFACE_WITH_KNOTS('',2,1,((#45576,#45577),(#45578,#45579),
(#45580,#45581)),.UNSPECIFIED.,.F.,.F.,.F.,(3,3),(2,2),(0.,1.),(0.,0.0300000000000002),
 .UNSPECIFIED.);
#472=B_SPLINE_SURFACE_WITH_KNOTS('',2,1,((#45591,#45592),(#45593,#45594),
(#45595,#45596)),.UNSPECIFIED.,.F.,.F.,.F.,(3,3),(2,2),(0.,1.),(0.,0.0300000000000002),
 .UNSPECIFIED.);
#473=B_SPLINE_SURFACE_WITH_KNOTS('',2,1,((#45606,#45607),(#45608,#45609),
(#45610,#45611)),.UNSPECIFIED.,.F.,.F.,.F.,(3,3),(2,2),(0.,1.),(0.,0.0300000000000002),
 .UNSPECIFIED.);
#474=B_SPLINE_SURFACE_WITH_KNOTS('',2,1,((#45621,#45622),(#45623,#45624),
(#45625,#45626)),.UNSPECIFIED.,.F.,.F.,.F.,(3,3),(2,2),(0.,1.),(0.,0.0300000000000002),
 .UNSPECIFIED.);
#475=B_SPLINE_SURFACE_WITH_KNOTS('',2,1,((#45636,#45637),(#45638,#45639),
(#45640,#45641)),.UNSPECIFIED.,.F.,.F.,.F.,(3,3),(2,2),(0.,1.),(0.,0.0300000000000002),
 .UNSPECIFIED.);
#476=B_SPLINE_SURFACE_WITH_KNOTS('',2,1,((#45651,#45652),(#45653,#45654),
(#45655,#45656)),.UNSPECIFIED.,.F.,.F.,.F.,(3,3),(2,2),(0.,1.),(0.,0.0300000000000002),
 .UNSPECIFIED.);
#477=B_SPLINE_SURFACE_WITH_KNOTS('',2,1,((#45666,#45667),(#45668,#45669),
(#45670,#45671)),.UNSPECIFIED.,.F.,.F.,.F.,(3,3),(2,2),(0.,1.),(0.,0.0300000000000002),
 .UNSPECIFIED.);
#478=B_SPLINE_SURFACE_WITH_KNOTS('',2,1,((#45687,#45688),(#45689,#45690),
(#45691,#45692)),.UNSPECIFIED.,.F.,.F.,.F.,(3,3),(2,2),(0.,1.),(0.,0.0300000000000002),
 .UNSPECIFIED.);
#479=B_SPLINE_SURFACE_WITH_KNOTS('',2,1,((#45702,#45703),(#45704,#45705),
(#45706,#45707)),.UNSPECIFIED.,.F.,.F.,.F.,(3,3),(2,2),(0.,1.),(0.,0.0300000000000002),
 .UNSPECIFIED.);
#480=B_SPLINE_SURFACE_WITH_KNOTS('',2,1,((#45715,#45716),(#45717,#45718),
(#45719,#45720)),.UNSPECIFIED.,.F.,.F.,.F.,(3,3),(2,2),(0.,1.),(0.,0.0300000000000002),
 .UNSPECIFIED.);
#481=B_SPLINE_SURFACE_WITH_KNOTS('',2,1,((#45733,#45734),(#45735,#45736),
(#45737,#45738)),.UNSPECIFIED.,.F.,.F.,.F.,(3,3),(2,2),(0.,1.),(0.,0.0300000000000002),
 .UNSPECIFIED.);
#482=B_SPLINE_SURFACE_WITH_KNOTS('',2,1,((#45748,#45749),(#45750,#45751),
(#45752,#45753)),.UNSPECIFIED.,.F.,.F.,.F.,(3,3),(2,2),(0.,1.),(0.,0.0300000000000002),
 .UNSPECIFIED.);
#483=B_SPLINE_SURFACE_WITH_KNOTS('',2,1,((#45763,#45764),(#45765,#45766),
(#45767,#45768)),.UNSPECIFIED.,.F.,.F.,.F.,(3,3),(2,2),(0.,1.),(0.,0.0300000000000002),
 .UNSPECIFIED.);
#484=B_SPLINE_SURFACE_WITH_KNOTS('',2,1,((#45778,#45779),(#45780,#45781),
(#45782,#45783)),.UNSPECIFIED.,.F.,.F.,.F.,(3,3),(2,2),(0.,1.),(0.,0.0300000000000002),
 .UNSPECIFIED.);
#485=B_SPLINE_SURFACE_WITH_KNOTS('',2,1,((#45793,#45794),(#45795,#45796),
(#45797,#45798)),.UNSPECIFIED.,.F.,.F.,.F.,(3,3),(2,2),(0.,1.),(0.,0.0300000000000002),
 .UNSPECIFIED.);
#486=B_SPLINE_SURFACE_WITH_KNOTS('',2,1,((#45808,#45809),(#45810,#45811),
(#45812,#45813)),.UNSPECIFIED.,.F.,.F.,.F.,(3,3),(2,2),(0.,1.),(0.,0.0300000000000002),
 .UNSPECIFIED.);
#487=B_SPLINE_SURFACE_WITH_KNOTS('',2,1,((#45823,#45824),(#45825,#45826),
(#45827,#45828)),.UNSPECIFIED.,.F.,.F.,.F.,(3,3),(2,2),(0.,1.),(0.,0.0300000000000002),
 .UNSPECIFIED.);
#488=B_SPLINE_SURFACE_WITH_KNOTS('',2,1,((#45844,#45845),(#45846,#45847),
(#45848,#45849)),.UNSPECIFIED.,.F.,.F.,.F.,(3,3),(2,2),(0.,1.),(0.,0.0300000000000002),
 .UNSPECIFIED.);
#489=B_SPLINE_SURFACE_WITH_KNOTS('',2,1,((#45859,#45860),(#45861,#45862),
(#45863,#45864)),.UNSPECIFIED.,.F.,.F.,.F.,(3,3),(2,2),(0.,1.),(0.,0.0300000000000002),
 .UNSPECIFIED.);
#490=B_SPLINE_SURFACE_WITH_KNOTS('',2,1,((#45874,#45875),(#45876,#45877),
(#45878,#45879)),.UNSPECIFIED.,.F.,.F.,.F.,(3,3),(2,2),(0.,1.),(0.,0.0300000000000002),
 .UNSPECIFIED.);
#491=B_SPLINE_SURFACE_WITH_KNOTS('',2,1,((#45889,#45890),(#45891,#45892),
(#45893,#45894)),.UNSPECIFIED.,.F.,.F.,.F.,(3,3),(2,2),(0.,1.),(0.,0.0300000000000002),
 .UNSPECIFIED.);
#492=B_SPLINE_SURFACE_WITH_KNOTS('',2,1,((#45904,#45905),(#45906,#45907),
(#45908,#45909)),.UNSPECIFIED.,.F.,.F.,.F.,(3,3),(2,2),(0.,1.),(0.,0.0300000000000002),
 .UNSPECIFIED.);
#493=B_SPLINE_SURFACE_WITH_KNOTS('',2,1,((#45919,#45920),(#45921,#45922),
(#45923,#45924)),.UNSPECIFIED.,.F.,.F.,.F.,(3,3),(2,2),(0.,1.),(0.,0.0300000000000002),
 .UNSPECIFIED.);
#494=B_SPLINE_SURFACE_WITH_KNOTS('',2,1,((#45934,#45935),(#45936,#45937),
(#45938,#45939)),.UNSPECIFIED.,.F.,.F.,.F.,(3,3),(2,2),(0.,1.),(0.,0.0300000000000002),
 .UNSPECIFIED.);
#495=B_SPLINE_SURFACE_WITH_KNOTS('',2,1,((#45949,#45950),(#45951,#45952),
(#45953,#45954)),.UNSPECIFIED.,.F.,.F.,.F.,(3,3),(2,2),(0.,1.),(0.,0.0300000000000002),
 .UNSPECIFIED.);
#496=B_SPLINE_SURFACE_WITH_KNOTS('',2,1,((#45964,#45965),(#45966,#45967),
(#45968,#45969)),.UNSPECIFIED.,.F.,.F.,.F.,(3,3),(2,2),(0.,1.),(0.,0.0300000000000002),
 .UNSPECIFIED.);
#497=B_SPLINE_SURFACE_WITH_KNOTS('',2,1,((#45997,#45998),(#45999,#46000),
(#46001,#46002)),.UNSPECIFIED.,.F.,.F.,.F.,(3,3),(2,2),(0.,1.),(0.,0.0300000000000002),
 .UNSPECIFIED.);
#498=B_SPLINE_SURFACE_WITH_KNOTS('',2,1,((#46019,#46020),(#46021,#46022),
(#46023,#46024)),.UNSPECIFIED.,.F.,.F.,.F.,(3,3),(2,2),(0.,1.),(0.,0.0300000000000002),
 .UNSPECIFIED.);
#499=B_SPLINE_SURFACE_WITH_KNOTS('',2,1,((#46034,#46035),(#46036,#46037),
(#46038,#46039)),.UNSPECIFIED.,.F.,.F.,.F.,(3,3),(2,2),(0.,1.),(0.,0.0300000000000002),
 .UNSPECIFIED.);
#500=B_SPLINE_SURFACE_WITH_KNOTS('',2,1,((#46049,#46050),(#46051,#46052),
(#46053,#46054)),.UNSPECIFIED.,.F.,.F.,.F.,(3,3),(2,2),(0.,1.),(0.,0.0300000000000002),
 .UNSPECIFIED.);
#501=B_SPLINE_SURFACE_WITH_KNOTS('',2,1,((#46064,#46065),(#46066,#46067),
(#46068,#46069)),.UNSPECIFIED.,.F.,.F.,.F.,(3,3),(2,2),(0.,1.),(0.,0.0300000000000002),
 .UNSPECIFIED.);
#502=B_SPLINE_SURFACE_WITH_KNOTS('',2,1,((#46079,#46080),(#46081,#46082),
(#46083,#46084)),.UNSPECIFIED.,.F.,.F.,.F.,(3,3),(2,2),(0.,1.),(0.,0.0300000000000002),
 .UNSPECIFIED.);
#503=B_SPLINE_SURFACE_WITH_KNOTS('',2,1,((#46112,#46113),(#46114,#46115),
(#46116,#46117)),.UNSPECIFIED.,.F.,.F.,.F.,(3,3),(2,2),(0.,1.),(0.,0.0300000000000002),
 .UNSPECIFIED.);
#504=B_SPLINE_SURFACE_WITH_KNOTS('',2,1,((#46127,#46128),(#46129,#46130),
(#46131,#46132)),.UNSPECIFIED.,.F.,.F.,.F.,(3,3),(2,2),(0.,1.),(0.,0.0300000000000002),
 .UNSPECIFIED.);
#505=B_SPLINE_SURFACE_WITH_KNOTS('',2,1,((#46142,#46143),(#46144,#46145),
(#46146,#46147)),.UNSPECIFIED.,.F.,.F.,.F.,(3,3),(2,2),(0.,1.),(0.,0.0300000000000002),
 .UNSPECIFIED.);
#506=B_SPLINE_SURFACE_WITH_KNOTS('',2,1,((#46157,#46158),(#46159,#46160),
(#46161,#46162)),.UNSPECIFIED.,.F.,.F.,.F.,(3,3),(2,2),(0.,1.),(0.,0.0300000000000002),
 .UNSPECIFIED.);
#507=B_SPLINE_SURFACE_WITH_KNOTS('',2,1,((#46172,#46173),(#46174,#46175),
(#46176,#46177)),.UNSPECIFIED.,.F.,.F.,.F.,(3,3),(2,2),(0.,1.),(0.,0.0300000000000002),
 .UNSPECIFIED.);
#508=B_SPLINE_SURFACE_WITH_KNOTS('',2,1,((#46187,#46188),(#46189,#46190),
(#46191,#46192)),.UNSPECIFIED.,.F.,.F.,.F.,(3,3),(2,2),(0.,1.),(0.,0.0300000000000002),
 .UNSPECIFIED.);
#509=B_SPLINE_SURFACE_WITH_KNOTS('',2,1,((#46224,#46225),(#46226,#46227),
(#46228,#46229)),.UNSPECIFIED.,.F.,.F.,.F.,(3,3),(2,2),(0.,1.),(0.,0.0300000000000002),
 .UNSPECIFIED.);
#510=B_SPLINE_SURFACE_WITH_KNOTS('',2,1,((#46242,#46243),(#46244,#46245),
(#46246,#46247)),.UNSPECIFIED.,.F.,.F.,.F.,(3,3),(2,2),(0.,1.),(0.,0.0300000000000002),
 .UNSPECIFIED.);
#511=B_SPLINE_SURFACE_WITH_KNOTS('',2,1,((#46257,#46258),(#46259,#46260),
(#46261,#46262)),.UNSPECIFIED.,.F.,.F.,.F.,(3,3),(2,2),(0.,1.),(0.,0.0300000000000002),
 .UNSPECIFIED.);
#512=B_SPLINE_SURFACE_WITH_KNOTS('',2,1,((#46272,#46273),(#46274,#46275),
(#46276,#46277)),.UNSPECIFIED.,.F.,.F.,.F.,(3,3),(2,2),(0.,1.),(0.,0.0300000000000002),
 .UNSPECIFIED.);
#513=B_SPLINE_SURFACE_WITH_KNOTS('',2,1,((#46287,#46288),(#46289,#46290),
(#46291,#46292)),.UNSPECIFIED.,.F.,.F.,.F.,(3,3),(2,2),(0.,1.),(0.,0.0300000000000002),
 .UNSPECIFIED.);
#514=B_SPLINE_SURFACE_WITH_KNOTS('',2,1,((#46302,#46303),(#46304,#46305),
(#46306,#46307)),.UNSPECIFIED.,.F.,.F.,.F.,(3,3),(2,2),(0.,1.),(0.,0.0300000000000002),
 .UNSPECIFIED.);
#515=B_SPLINE_SURFACE_WITH_KNOTS('',2,1,((#46317,#46318),(#46319,#46320),
(#46321,#46322)),.UNSPECIFIED.,.F.,.F.,.F.,(3,3),(2,2),(0.,1.),(0.,0.0300000000000002),
 .UNSPECIFIED.);
#516=B_SPLINE_SURFACE_WITH_KNOTS('',2,1,((#46332,#46333),(#46334,#46335),
(#46336,#46337)),.UNSPECIFIED.,.F.,.F.,.F.,(3,3),(2,2),(0.,1.),(0.,0.0300000000000002),
 .UNSPECIFIED.);
#517=B_SPLINE_SURFACE_WITH_KNOTS('',2,1,((#46347,#46348),(#46349,#46350),
(#46351,#46352)),.UNSPECIFIED.,.F.,.F.,.F.,(3,3),(2,2),(0.,1.),(0.,0.0300000000000002),
 .UNSPECIFIED.);
#518=B_SPLINE_SURFACE_WITH_KNOTS('',2,1,((#46359,#46360),(#46361,#46362),
(#46363,#46364)),.UNSPECIFIED.,.F.,.F.,.F.,(3,3),(2,2),(0.,1.),(0.,0.0300000000000002),
 .UNSPECIFIED.);
#519=B_SPLINE_SURFACE_WITH_KNOTS('',2,1,((#46377,#46378),(#46379,#46380),
(#46381,#46382)),.UNSPECIFIED.,.F.,.F.,.F.,(3,3),(2,2),(0.,1.),(0.,0.0300000000000002),
 .UNSPECIFIED.);
#520=B_SPLINE_SURFACE_WITH_KNOTS('',2,1,((#46392,#46393),(#46394,#46395),
(#46396,#46397)),.UNSPECIFIED.,.F.,.F.,.F.,(3,3),(2,2),(0.,1.),(0.,0.0300000000000002),
 .UNSPECIFIED.);
#521=B_SPLINE_SURFACE_WITH_KNOTS('',2,1,((#46407,#46408),(#46409,#46410),
(#46411,#46412)),.UNSPECIFIED.,.F.,.F.,.F.,(3,3),(2,2),(0.,1.),(0.,0.0300000000000002),
 .UNSPECIFIED.);
#522=B_SPLINE_SURFACE_WITH_KNOTS('',2,1,((#46422,#46423),(#46424,#46425),
(#46426,#46427)),.UNSPECIFIED.,.F.,.F.,.F.,(3,3),(2,2),(0.,1.),(0.,0.0300000000000002),
 .UNSPECIFIED.);
#523=B_SPLINE_SURFACE_WITH_KNOTS('',2,1,((#46437,#46438),(#46439,#46440),
(#46441,#46442)),.UNSPECIFIED.,.F.,.F.,.F.,(3,3),(2,2),(0.,1.),(0.,0.0300000000000002),
 .UNSPECIFIED.);
#524=B_SPLINE_SURFACE_WITH_KNOTS('',2,1,((#46452,#46453),(#46454,#46455),
(#46456,#46457)),.UNSPECIFIED.,.F.,.F.,.F.,(3,3),(2,2),(0.,1.),(0.,0.0300000000000002),
 .UNSPECIFIED.);
#525=B_SPLINE_SURFACE_WITH_KNOTS('',2,1,((#46467,#46468),(#46469,#46470),
(#46471,#46472)),.UNSPECIFIED.,.F.,.F.,.F.,(3,3),(2,2),(0.,1.),(0.,0.0300000000000002),
 .UNSPECIFIED.);
#526=B_SPLINE_SURFACE_WITH_KNOTS('',2,1,((#46482,#46483),(#46484,#46485),
(#46486,#46487)),.UNSPECIFIED.,.F.,.F.,.F.,(3,3),(2,2),(0.,1.),(0.,0.0300000000000002),
 .UNSPECIFIED.);
#527=B_SPLINE_SURFACE_WITH_KNOTS('',2,1,((#46497,#46498),(#46499,#46500),
(#46501,#46502)),.UNSPECIFIED.,.F.,.F.,.F.,(3,3),(2,2),(0.,1.),(0.,0.0300000000000002),
 .UNSPECIFIED.);
#528=B_SPLINE_SURFACE_WITH_KNOTS('',2,1,((#46512,#46513),(#46514,#46515),
(#46516,#46517)),.UNSPECIFIED.,.F.,.F.,.F.,(3,3),(2,2),(0.,1.),(0.,0.0300000000000002),
 .UNSPECIFIED.);
#529=B_SPLINE_SURFACE_WITH_KNOTS('',2,1,((#46527,#46528),(#46529,#46530),
(#46531,#46532)),.UNSPECIFIED.,.F.,.F.,.F.,(3,3),(2,2),(0.,1.),(0.,0.0300000000000002),
 .UNSPECIFIED.);
#530=B_SPLINE_SURFACE_WITH_KNOTS('',2,1,((#46542,#46543),(#46544,#46545),
(#46546,#46547)),.UNSPECIFIED.,.F.,.F.,.F.,(3,3),(2,2),(0.,1.),(0.,0.0300000000000002),
 .UNSPECIFIED.);
#531=B_SPLINE_SURFACE_WITH_KNOTS('',2,1,((#46557,#46558),(#46559,#46560),
(#46561,#46562)),.UNSPECIFIED.,.F.,.F.,.F.,(3,3),(2,2),(0.,1.),(0.,0.0300000000000002),
 .UNSPECIFIED.);
#532=B_SPLINE_SURFACE_WITH_KNOTS('',2,1,((#46572,#46573),(#46574,#46575),
(#46576,#46577)),.UNSPECIFIED.,.F.,.F.,.F.,(3,3),(2,2),(0.,1.),(0.,0.0300000000000002),
 .UNSPECIFIED.);
#533=B_SPLINE_SURFACE_WITH_KNOTS('',2,1,((#46587,#46588),(#46589,#46590),
(#46591,#46592)),.UNSPECIFIED.,.F.,.F.,.F.,(3,3),(2,2),(0.,1.),(0.,0.0300000000000002),
 .UNSPECIFIED.);
#534=B_SPLINE_SURFACE_WITH_KNOTS('',2,1,((#46608,#46609),(#46610,#46611),
(#46612,#46613)),.UNSPECIFIED.,.F.,.F.,.F.,(3,3),(2,2),(0.,1.),(0.,0.0300000000000002),
 .UNSPECIFIED.);
#535=B_SPLINE_SURFACE_WITH_KNOTS('',2,1,((#46623,#46624),(#46625,#46626),
(#46627,#46628)),.UNSPECIFIED.,.F.,.F.,.F.,(3,3),(2,2),(0.,1.),(0.,0.0300000000000002),
 .UNSPECIFIED.);
#536=B_SPLINE_SURFACE_WITH_KNOTS('',2,1,((#46636,#46637),(#46638,#46639),
(#46640,#46641)),.UNSPECIFIED.,.F.,.F.,.F.,(3,3),(2,2),(0.,1.),(0.,0.0300000000000002),
 .UNSPECIFIED.);
#537=B_SPLINE_SURFACE_WITH_KNOTS('',2,1,((#46654,#46655),(#46656,#46657),
(#46658,#46659)),.UNSPECIFIED.,.F.,.F.,.F.,(3,3),(2,2),(0.,1.),(0.,0.0300000000000002),
 .UNSPECIFIED.);
#538=B_SPLINE_SURFACE_WITH_KNOTS('',2,1,((#46669,#46670),(#46671,#46672),
(#46673,#46674)),.UNSPECIFIED.,.F.,.F.,.F.,(3,3),(2,2),(0.,1.),(0.,0.0300000000000002),
 .UNSPECIFIED.);
#539=B_SPLINE_SURFACE_WITH_KNOTS('',2,1,((#46684,#46685),(#46686,#46687),
(#46688,#46689)),.UNSPECIFIED.,.F.,.F.,.F.,(3,3),(2,2),(0.,1.),(0.,0.0300000000000002),
 .UNSPECIFIED.);
#540=B_SPLINE_SURFACE_WITH_KNOTS('',2,1,((#46699,#46700),(#46701,#46702),
(#46703,#46704)),.UNSPECIFIED.,.F.,.F.,.F.,(3,3),(2,2),(0.,1.),(0.,0.0300000000000002),
 .UNSPECIFIED.);
#541=B_SPLINE_SURFACE_WITH_KNOTS('',2,1,((#46714,#46715),(#46716,#46717),
(#46718,#46719)),.UNSPECIFIED.,.F.,.F.,.F.,(3,3),(2,2),(0.,1.),(0.,0.0300000000000002),
 .UNSPECIFIED.);
#542=B_SPLINE_SURFACE_WITH_KNOTS('',2,1,((#46729,#46730),(#46731,#46732),
(#46733,#46734)),.UNSPECIFIED.,.F.,.F.,.F.,(3,3),(2,2),(0.,1.),(0.,0.0300000000000002),
 .UNSPECIFIED.);
#543=B_SPLINE_SURFACE_WITH_KNOTS('',2,1,((#46744,#46745),(#46746,#46747),
(#46748,#46749)),.UNSPECIFIED.,.F.,.F.,.F.,(3,3),(2,2),(0.,1.),(0.,0.0300000000000002),
 .UNSPECIFIED.);
#544=B_SPLINE_SURFACE_WITH_KNOTS('',2,1,((#46756,#46757),(#46758,#46759),
(#46760,#46761)),.UNSPECIFIED.,.F.,.F.,.F.,(3,3),(2,2),(0.,1.),(0.,0.0300000000000002),
 .UNSPECIFIED.);
#545=B_SPLINE_SURFACE_WITH_KNOTS('',2,1,((#46774,#46775),(#46776,#46777),
(#46778,#46779)),.UNSPECIFIED.,.F.,.F.,.F.,(3,3),(2,2),(0.,1.),(0.,0.0300000000000002),
 .UNSPECIFIED.);
#546=B_SPLINE_SURFACE_WITH_KNOTS('',2,1,((#46789,#46790),(#46791,#46792),
(#46793,#46794)),.UNSPECIFIED.,.F.,.F.,.F.,(3,3),(2,2),(0.,1.),(0.,0.0300000000000002),
 .UNSPECIFIED.);
#547=B_SPLINE_SURFACE_WITH_KNOTS('',2,1,((#46804,#46805),(#46806,#46807),
(#46808,#46809)),.UNSPECIFIED.,.F.,.F.,.F.,(3,3),(2,2),(0.,1.),(0.,0.0300000000000002),
 .UNSPECIFIED.);
#548=B_SPLINE_SURFACE_WITH_KNOTS('',2,1,((#46819,#46820),(#46821,#46822),
(#46823,#46824)),.UNSPECIFIED.,.F.,.F.,.F.,(3,3),(2,2),(0.,1.),(0.,0.0300000000000002),
 .UNSPECIFIED.);
#549=B_SPLINE_SURFACE_WITH_KNOTS('',2,1,((#46834,#46835),(#46836,#46837),
(#46838,#46839)),.UNSPECIFIED.,.F.,.F.,.F.,(3,3),(2,2),(0.,1.),(0.,0.0300000000000002),
 .UNSPECIFIED.);
#550=B_SPLINE_SURFACE_WITH_KNOTS('',2,1,((#46849,#46850),(#46851,#46852),
(#46853,#46854)),.UNSPECIFIED.,.F.,.F.,.F.,(3,3),(2,2),(0.,1.),(0.,0.0300000000000002),
 .UNSPECIFIED.);
#551=B_SPLINE_SURFACE_WITH_KNOTS('',2,1,((#46894,#46895),(#46896,#46897),
(#46898,#46899)),.UNSPECIFIED.,.F.,.F.,.F.,(3,3),(2,2),(0.,1.),(0.,0.0300000000000002),
 .UNSPECIFIED.);
#552=B_SPLINE_SURFACE_WITH_KNOTS('',2,1,((#46907,#46908),(#46909,#46910),
(#46911,#46912)),.UNSPECIFIED.,.F.,.F.,.F.,(3,3),(2,2),(0.,1.),(0.,0.0300000000000002),
 .UNSPECIFIED.);
#553=B_SPLINE_SURFACE_WITH_KNOTS('',2,1,((#46925,#46926),(#46927,#46928),
(#46929,#46930)),.UNSPECIFIED.,.F.,.F.,.F.,(3,3),(2,2),(0.,1.),(0.,0.0300000000000002),
 .UNSPECIFIED.);
#554=B_SPLINE_SURFACE_WITH_KNOTS('',2,1,((#46940,#46941),(#46942,#46943),
(#46944,#46945)),.UNSPECIFIED.,.F.,.F.,.F.,(3,3),(2,2),(0.,1.),(0.,0.0300000000000002),
 .UNSPECIFIED.);
#555=B_SPLINE_SURFACE_WITH_KNOTS('',2,1,((#46955,#46956),(#46957,#46958),
(#46959,#46960)),.UNSPECIFIED.,.F.,.F.,.F.,(3,3),(2,2),(0.,1.),(0.,0.0300000000000002),
 .UNSPECIFIED.);
#556=B_SPLINE_SURFACE_WITH_KNOTS('',2,1,((#46976,#46977),(#46978,#46979),
(#46980,#46981)),.UNSPECIFIED.,.F.,.F.,.F.,(3,3),(2,2),(0.,1.),(0.,0.0300000000000002),
 .UNSPECIFIED.);
#557=B_SPLINE_SURFACE_WITH_KNOTS('',2,1,((#46991,#46992),(#46993,#46994),
(#46995,#46996)),.UNSPECIFIED.,.F.,.F.,.F.,(3,3),(2,2),(0.,1.),(0.,0.0300000000000002),
 .UNSPECIFIED.);
#558=B_SPLINE_SURFACE_WITH_KNOTS('',2,1,((#47006,#47007),(#47008,#47009),
(#47010,#47011)),.UNSPECIFIED.,.F.,.F.,.F.,(3,3),(2,2),(0.,1.),(0.,0.0300000000000002),
 .UNSPECIFIED.);
#716=B_SPLINE_CURVE_WITH_KNOTS('',2,(#43224,#43225,#43226),
 .UNSPECIFIED.,.F.,.F.,(3,3),(0.,1.),.UNSPECIFIED.);
#717=B_SPLINE_CURVE_WITH_KNOTS('',2,(#43230,#43231,#43232),
 .UNSPECIFIED.,.F.,.F.,(3,3),(0.,1.),.UNSPECIFIED.);
#718=B_SPLINE_CURVE_WITH_KNOTS('',2,(#43241,#43242,#43243),
 .UNSPECIFIED.,.F.,.F.,(3,3),(0.,1.),.UNSPECIFIED.);
#719=B_SPLINE_CURVE_WITH_KNOTS('',2,(#43246,#43247,#43248),
 .UNSPECIFIED.,.F.,.F.,(3,3),(0.,1.),.UNSPECIFIED.);
#720=B_SPLINE_CURVE_WITH_KNOTS('',2,(#43256,#43257,#43258),
 .UNSPECIFIED.,.F.,.F.,(3,3),(0.,1.),.UNSPECIFIED.);
#721=B_SPLINE_CURVE_WITH_KNOTS('',2,(#43261,#43262,#43263),
 .UNSPECIFIED.,.F.,.F.,(3,3),(0.,1.),.UNSPECIFIED.);
#722=B_SPLINE_CURVE_WITH_KNOTS('',2,(#43271,#43272,#43273),
 .UNSPECIFIED.,.F.,.F.,(3,3),(0.,1.),.UNSPECIFIED.);
#723=B_SPLINE_CURVE_WITH_KNOTS('',2,(#43276,#43277,#43278),
 .UNSPECIFIED.,.F.,.F.,(3,3),(0.,1.),.UNSPECIFIED.);
#724=B_SPLINE_CURVE_WITH_KNOTS('',2,(#43286,#43287,#43288),
 .UNSPECIFIED.,.F.,.F.,(3,3),(0.,1.),.UNSPECIFIED.);
#725=B_SPLINE_CURVE_WITH_KNOTS('',2,(#43291,#43292,#43293),
 .UNSPECIFIED.,.F.,.F.,(3,3),(0.,1.),.UNSPECIFIED.);
#726=B_SPLINE_CURVE_WITH_KNOTS('',2,(#43301,#43302,#43303),
 .UNSPECIFIED.,.F.,.F.,(3,3),(0.,1.),.UNSPECIFIED.);
#727=B_SPLINE_CURVE_WITH_KNOTS('',2,(#43306,#43307,#43308),
 .UNSPECIFIED.,.F.,.F.,(3,3),(0.,1.),.UNSPECIFIED.);
#728=B_SPLINE_CURVE_WITH_KNOTS('',2,(#43316,#43317,#43318),
 .UNSPECIFIED.,.F.,.F.,(3,3),(0.,1.),.UNSPECIFIED.);
#729=B_SPLINE_CURVE_WITH_KNOTS('',2,(#43321,#43322,#43323),
 .UNSPECIFIED.,.F.,.F.,(3,3),(0.,1.),.UNSPECIFIED.);
#730=B_SPLINE_CURVE_WITH_KNOTS('',2,(#43331,#43332,#43333),
 .UNSPECIFIED.,.F.,.F.,(3,3),(0.,1.),.UNSPECIFIED.);
#731=B_SPLINE_CURVE_WITH_KNOTS('',2,(#43336,#43337,#43338),
 .UNSPECIFIED.,.F.,.F.,(3,3),(0.,1.),.UNSPECIFIED.);
#732=B_SPLINE_CURVE_WITH_KNOTS('',2,(#43346,#43347,#43348),
 .UNSPECIFIED.,.F.,.F.,(3,3),(0.,1.),.UNSPECIFIED.);
#733=B_SPLINE_CURVE_WITH_KNOTS('',2,(#43351,#43352,#43353),
 .UNSPECIFIED.,.F.,.F.,(3,3),(0.,1.),.UNSPECIFIED.);
#734=B_SPLINE_CURVE_WITH_KNOTS('',2,(#43365,#43366,#43367),
 .UNSPECIFIED.,.F.,.F.,(3,3),(0.,1.),.UNSPECIFIED.);
#735=B_SPLINE_CURVE_WITH_KNOTS('',2,(#43371,#43372,#43373),
 .UNSPECIFIED.,.F.,.F.,(3,3),(0.,1.),.UNSPECIFIED.);
#736=B_SPLINE_CURVE_WITH_KNOTS('',2,(#43382,#43383,#43384),
 .UNSPECIFIED.,.F.,.F.,(3,3),(0.,1.),.UNSPECIFIED.);
#737=B_SPLINE_CURVE_WITH_KNOTS('',2,(#43387,#43388,#43389),
 .UNSPECIFIED.,.F.,.F.,(3,3),(0.,1.),.UNSPECIFIED.);
#738=B_SPLINE_CURVE_WITH_KNOTS('',2,(#43403,#43404,#43405),
 .UNSPECIFIED.,.F.,.F.,(3,3),(0.,1.),.UNSPECIFIED.);
#739=B_SPLINE_CURVE_WITH_KNOTS('',2,(#43408,#43409,#43410),
 .UNSPECIFIED.,.F.,.F.,(3,3),(0.,1.),.UNSPECIFIED.);
#740=B_SPLINE_CURVE_WITH_KNOTS('',2,(#43418,#43419,#43420),
 .UNSPECIFIED.,.F.,.F.,(3,3),(0.,1.),.UNSPECIFIED.);
#741=B_SPLINE_CURVE_WITH_KNOTS('',2,(#43423,#43424,#43425),
 .UNSPECIFIED.,.F.,.F.,(3,3),(0.,1.),.UNSPECIFIED.);
#742=B_SPLINE_CURVE_WITH_KNOTS('',2,(#43433,#43434,#43435),
 .UNSPECIFIED.,.F.,.F.,(3,3),(0.,1.),.UNSPECIFIED.);
#743=B_SPLINE_CURVE_WITH_KNOTS('',2,(#43438,#43439,#43440),
 .UNSPECIFIED.,.F.,.F.,(3,3),(0.,1.),.UNSPECIFIED.);
#744=B_SPLINE_CURVE_WITH_KNOTS('',2,(#43448,#43449,#43450),
 .UNSPECIFIED.,.F.,.F.,(3,3),(0.,1.),.UNSPECIFIED.);
#745=B_SPLINE_CURVE_WITH_KNOTS('',2,(#43453,#43454,#43455),
 .UNSPECIFIED.,.F.,.F.,(3,3),(0.,1.),.UNSPECIFIED.);
#746=B_SPLINE_CURVE_WITH_KNOTS('',2,(#43463,#43464,#43465),
 .UNSPECIFIED.,.F.,.F.,(3,3),(0.,1.),.UNSPECIFIED.);
#747=B_SPLINE_CURVE_WITH_KNOTS('',2,(#43468,#43469,#43470),
 .UNSPECIFIED.,.F.,.F.,(3,3),(0.,1.),.UNSPECIFIED.);
#748=B_SPLINE_CURVE_WITH_KNOTS('',2,(#43478,#43479,#43480),
 .UNSPECIFIED.,.F.,.F.,(3,3),(0.,1.),.UNSPECIFIED.);
#749=B_SPLINE_CURVE_WITH_KNOTS('',2,(#43483,#43484,#43485),
 .UNSPECIFIED.,.F.,.F.,(3,3),(0.,1.),.UNSPECIFIED.);
#750=B_SPLINE_CURVE_WITH_KNOTS('',2,(#43493,#43494,#43495),
 .UNSPECIFIED.,.F.,.F.,(3,3),(0.,1.),.UNSPECIFIED.);
#751=B_SPLINE_CURVE_WITH_KNOTS('',2,(#43498,#43499,#43500),
 .UNSPECIFIED.,.F.,.F.,(3,3),(0.,1.),.UNSPECIFIED.);
#752=B_SPLINE_CURVE_WITH_KNOTS('',2,(#43514,#43515,#43516),
 .UNSPECIFIED.,.F.,.F.,(3,3),(0.,1.),.UNSPECIFIED.);
#753=B_SPLINE_CURVE_WITH_KNOTS('',2,(#43519,#43520,#43521),
 .UNSPECIFIED.,.F.,.F.,(3,3),(0.,1.),.UNSPECIFIED.);
#754=B_SPLINE_CURVE_WITH_KNOTS('',2,(#43529,#43530,#43531),
 .UNSPECIFIED.,.F.,.F.,(3,3),(0.,1.),.UNSPECIFIED.);
#755=B_SPLINE_CURVE_WITH_KNOTS('',2,(#43534,#43535,#43536),
 .UNSPECIFIED.,.F.,.F.,(3,3),(0.,1.),.UNSPECIFIED.);
#756=B_SPLINE_CURVE_WITH_KNOTS('',2,(#43544,#43545,#43546),
 .UNSPECIFIED.,.F.,.F.,(3,3),(0.,1.),.UNSPECIFIED.);
#757=B_SPLINE_CURVE_WITH_KNOTS('',2,(#43549,#43550,#43551),
 .UNSPECIFIED.,.F.,.F.,(3,3),(0.,1.),.UNSPECIFIED.);
#758=B_SPLINE_CURVE_WITH_KNOTS('',2,(#43559,#43560,#43561),
 .UNSPECIFIED.,.F.,.F.,(3,3),(0.,1.),.UNSPECIFIED.);
#759=B_SPLINE_CURVE_WITH_KNOTS('',2,(#43564,#43565,#43566),
 .UNSPECIFIED.,.F.,.F.,(3,3),(0.,1.),.UNSPECIFIED.);
#760=B_SPLINE_CURVE_WITH_KNOTS('',2,(#43574,#43575,#43576),
 .UNSPECIFIED.,.F.,.F.,(3,3),(0.,1.),.UNSPECIFIED.);
#761=B_SPLINE_CURVE_WITH_KNOTS('',2,(#43579,#43580,#43581),
 .UNSPECIFIED.,.F.,.F.,(3,3),(0.,1.),.UNSPECIFIED.);
#762=B_SPLINE_CURVE_WITH_KNOTS('',2,(#43589,#43590,#43591),
 .UNSPECIFIED.,.F.,.F.,(3,3),(0.,1.),.UNSPECIFIED.);
#763=B_SPLINE_CURVE_WITH_KNOTS('',2,(#43594,#43595,#43596),
 .UNSPECIFIED.,.F.,.F.,(3,3),(0.,1.),.UNSPECIFIED.);
#764=B_SPLINE_CURVE_WITH_KNOTS('',2,(#43604,#43605,#43606),
 .UNSPECIFIED.,.F.,.F.,(3,3),(0.,1.),.UNSPECIFIED.);
#765=B_SPLINE_CURVE_WITH_KNOTS('',2,(#43609,#43610,#43611),
 .UNSPECIFIED.,.F.,.F.,(3,3),(0.,1.),.UNSPECIFIED.);
#766=B_SPLINE_CURVE_WITH_KNOTS('',2,(#43619,#43620,#43621),
 .UNSPECIFIED.,.F.,.F.,(3,3),(0.,1.),.UNSPECIFIED.);
#767=B_SPLINE_CURVE_WITH_KNOTS('',2,(#43624,#43625,#43626),
 .UNSPECIFIED.,.F.,.F.,(3,3),(0.,1.),.UNSPECIFIED.);
#768=B_SPLINE_CURVE_WITH_KNOTS('',2,(#43634,#43635,#43636),
 .UNSPECIFIED.,.F.,.F.,(3,3),(0.,1.),.UNSPECIFIED.);
#769=B_SPLINE_CURVE_WITH_KNOTS('',2,(#43639,#43640,#43641),
 .UNSPECIFIED.,.F.,.F.,(3,3),(0.,1.),.UNSPECIFIED.);
#770=B_SPLINE_CURVE_WITH_KNOTS('',2,(#43649,#43650,#43651),
 .UNSPECIFIED.,.F.,.F.,(3,3),(0.,1.),.UNSPECIFIED.);
#771=B_SPLINE_CURVE_WITH_KNOTS('',2,(#43654,#43655,#43656),
 .UNSPECIFIED.,.F.,.F.,(3,3),(0.,1.),.UNSPECIFIED.);
#772=B_SPLINE_CURVE_WITH_KNOTS('',2,(#43664,#43665,#43666),
 .UNSPECIFIED.,.F.,.F.,(3,3),(0.,1.),.UNSPECIFIED.);
#773=B_SPLINE_CURVE_WITH_KNOTS('',2,(#43669,#43670,#43671),
 .UNSPECIFIED.,.F.,.F.,(3,3),(0.,1.),.UNSPECIFIED.);
#774=B_SPLINE_CURVE_WITH_KNOTS('',2,(#43679,#43680,#43681),
 .UNSPECIFIED.,.F.,.F.,(3,3),(0.,1.),.UNSPECIFIED.);
#775=B_SPLINE_CURVE_WITH_KNOTS('',2,(#43684,#43685,#43686),
 .UNSPECIFIED.,.F.,.F.,(3,3),(0.,1.),.UNSPECIFIED.);
#776=B_SPLINE_CURVE_WITH_KNOTS('',2,(#43694,#43695,#43696),
 .UNSPECIFIED.,.F.,.F.,(3,3),(0.,1.),.UNSPECIFIED.);
#777=B_SPLINE_CURVE_WITH_KNOTS('',2,(#43699,#43700,#43701),
 .UNSPECIFIED.,.F.,.F.,(3,3),(0.,1.),.UNSPECIFIED.);
#778=B_SPLINE_CURVE_WITH_KNOTS('',2,(#43709,#43710,#43711),
 .UNSPECIFIED.,.F.,.F.,(3,3),(0.,1.),.UNSPECIFIED.);
#779=B_SPLINE_CURVE_WITH_KNOTS('',2,(#43714,#43715,#43716),
 .UNSPECIFIED.,.F.,.F.,(3,3),(0.,1.),.UNSPECIFIED.);
#780=B_SPLINE_CURVE_WITH_KNOTS('',2,(#43724,#43725,#43726),
 .UNSPECIFIED.,.F.,.F.,(3,3),(0.,1.),.UNSPECIFIED.);
#781=B_SPLINE_CURVE_WITH_KNOTS('',2,(#43729,#43730,#43731),
 .UNSPECIFIED.,.F.,.F.,(3,3),(0.,1.),.UNSPECIFIED.);
#782=B_SPLINE_CURVE_WITH_KNOTS('',2,(#43744,#43745,#43746),
 .UNSPECIFIED.,.F.,.F.,(3,3),(0.,1.),.UNSPECIFIED.);
#783=B_SPLINE_CURVE_WITH_KNOTS('',2,(#43750,#43751,#43752),
 .UNSPECIFIED.,.F.,.F.,(3,3),(0.,1.),.UNSPECIFIED.);
#784=B_SPLINE_CURVE_WITH_KNOTS('',2,(#43761,#43762,#43763),
 .UNSPECIFIED.,.F.,.F.,(3,3),(0.,1.),.UNSPECIFIED.);
#785=B_SPLINE_CURVE_WITH_KNOTS('',2,(#43766,#43767,#43768),
 .UNSPECIFIED.,.F.,.F.,(3,3),(0.,1.),.UNSPECIFIED.);
#786=B_SPLINE_CURVE_WITH_KNOTS('',2,(#43776,#43777,#43778),
 .UNSPECIFIED.,.F.,.F.,(3,3),(0.,1.),.UNSPECIFIED.);
#787=B_SPLINE_CURVE_WITH_KNOTS('',2,(#43781,#43782,#43783),
 .UNSPECIFIED.,.F.,.F.,(3,3),(0.,1.),.UNSPECIFIED.);
#788=B_SPLINE_CURVE_WITH_KNOTS('',2,(#43791,#43792,#43793),
 .UNSPECIFIED.,.F.,.F.,(3,3),(0.,1.),.UNSPECIFIED.);
#789=B_SPLINE_CURVE_WITH_KNOTS('',2,(#43796,#43797,#43798),
 .UNSPECIFIED.,.F.,.F.,(3,3),(0.,1.),.UNSPECIFIED.);
#790=B_SPLINE_CURVE_WITH_KNOTS('',2,(#43806,#43807,#43808),
 .UNSPECIFIED.,.F.,.F.,(3,3),(0.,1.),.UNSPECIFIED.);
#791=B_SPLINE_CURVE_WITH_KNOTS('',2,(#43811,#43812,#43813),
 .UNSPECIFIED.,.F.,.F.,(3,3),(0.,1.),.UNSPECIFIED.);
#792=B_SPLINE_CURVE_WITH_KNOTS('',2,(#43821,#43822,#43823),
 .UNSPECIFIED.,.F.,.F.,(3,3),(0.,1.),.UNSPECIFIED.);
#793=B_SPLINE_CURVE_WITH_KNOTS('',2,(#43826,#43827,#43828),
 .UNSPECIFIED.,.F.,.F.,(3,3),(0.,1.),.UNSPECIFIED.);
#794=B_SPLINE_CURVE_WITH_KNOTS('',2,(#43836,#43837,#43838),
 .UNSPECIFIED.,.F.,.F.,(3,3),(0.,1.),.UNSPECIFIED.);
#795=B_SPLINE_CURVE_WITH_KNOTS('',2,(#43841,#43842,#43843),
 .UNSPECIFIED.,.F.,.F.,(3,3),(0.,1.),.UNSPECIFIED.);
#796=B_SPLINE_CURVE_WITH_KNOTS('',2,(#43850,#43851,#43852),
 .UNSPECIFIED.,.F.,.F.,(3,3),(0.,1.),.UNSPECIFIED.);
#797=B_SPLINE_CURVE_WITH_KNOTS('',2,(#43853,#43854,#43855),
 .UNSPECIFIED.,.F.,.F.,(3,3),(0.,1.),.UNSPECIFIED.);
#798=B_SPLINE_CURVE_WITH_KNOTS('',2,(#43864,#43865,#43866),
 .UNSPECIFIED.,.F.,.F.,(3,3),(0.,1.),.UNSPECIFIED.);
#799=B_SPLINE_CURVE_WITH_KNOTS('',2,(#43870,#43871,#43872),
 .UNSPECIFIED.,.F.,.F.,(3,3),(0.,1.),.UNSPECIFIED.);
#800=B_SPLINE_CURVE_WITH_KNOTS('',2,(#43881,#43882,#43883),
 .UNSPECIFIED.,.F.,.F.,(3,3),(0.,1.),.UNSPECIFIED.);
#801=B_SPLINE_CURVE_WITH_KNOTS('',2,(#43886,#43887,#43888),
 .UNSPECIFIED.,.F.,.F.,(3,3),(0.,1.),.UNSPECIFIED.);
#802=B_SPLINE_CURVE_WITH_KNOTS('',2,(#43896,#43897,#43898),
 .UNSPECIFIED.,.F.,.F.,(3,3),(0.,1.),.UNSPECIFIED.);
#803=B_SPLINE_CURVE_WITH_KNOTS('',2,(#43901,#43902,#43903),
 .UNSPECIFIED.,.F.,.F.,(3,3),(0.,1.),.UNSPECIFIED.);
#804=B_SPLINE_CURVE_WITH_KNOTS('',2,(#43911,#43912,#43913),
 .UNSPECIFIED.,.F.,.F.,(3,3),(0.,1.),.UNSPECIFIED.);
#805=B_SPLINE_CURVE_WITH_KNOTS('',2,(#43916,#43917,#43918),
 .UNSPECIFIED.,.F.,.F.,(3,3),(0.,1.),.UNSPECIFIED.);
#806=B_SPLINE_CURVE_WITH_KNOTS('',2,(#43926,#43927,#43928),
 .UNSPECIFIED.,.F.,.F.,(3,3),(0.,1.),.UNSPECIFIED.);
#807=B_SPLINE_CURVE_WITH_KNOTS('',2,(#43931,#43932,#43933),
 .UNSPECIFIED.,.F.,.F.,(3,3),(0.,1.),.UNSPECIFIED.);
#808=B_SPLINE_CURVE_WITH_KNOTS('',2,(#43941,#43942,#43943),
 .UNSPECIFIED.,.F.,.F.,(3,3),(0.,1.),.UNSPECIFIED.);
#809=B_SPLINE_CURVE_WITH_KNOTS('',2,(#43946,#43947,#43948),
 .UNSPECIFIED.,.F.,.F.,(3,3),(0.,1.),.UNSPECIFIED.);
#810=B_SPLINE_CURVE_WITH_KNOTS('',2,(#43956,#43957,#43958),
 .UNSPECIFIED.,.F.,.F.,(3,3),(0.,1.),.UNSPECIFIED.);
#811=B_SPLINE_CURVE_WITH_KNOTS('',2,(#43961,#43962,#43963),
 .UNSPECIFIED.,.F.,.F.,(3,3),(0.,1.),.UNSPECIFIED.);
#812=B_SPLINE_CURVE_WITH_KNOTS('',2,(#43971,#43972,#43973),
 .UNSPECIFIED.,.F.,.F.,(3,3),(0.,1.),.UNSPECIFIED.);
#813=B_SPLINE_CURVE_WITH_KNOTS('',2,(#43976,#43977,#43978),
 .UNSPECIFIED.,.F.,.F.,(3,3),(0.,1.),.UNSPECIFIED.);
#814=B_SPLINE_CURVE_WITH_KNOTS('',2,(#43986,#43987,#43988),
 .UNSPECIFIED.,.F.,.F.,(3,3),(0.,1.),.UNSPECIFIED.);
#815=B_SPLINE_CURVE_WITH_KNOTS('',2,(#43991,#43992,#43993),
 .UNSPECIFIED.,.F.,.F.,(3,3),(0.,1.),.UNSPECIFIED.);
#816=B_SPLINE_CURVE_WITH_KNOTS('',2,(#44001,#44002,#44003),
 .UNSPECIFIED.,.F.,.F.,(3,3),(0.,1.),.UNSPECIFIED.);
#817=B_SPLINE_CURVE_WITH_KNOTS('',2,(#44006,#44007,#44008),
 .UNSPECIFIED.,.F.,.F.,(3,3),(0.,1.),.UNSPECIFIED.);
#818=B_SPLINE_CURVE_WITH_KNOTS('',2,(#44016,#44017,#44018),
 .UNSPECIFIED.,.F.,.F.,(3,3),(0.,1.),.UNSPECIFIED.);
#819=B_SPLINE_CURVE_WITH_KNOTS('',2,(#44021,#44022,#44023),
 .UNSPECIFIED.,.F.,.F.,(3,3),(0.,1.),.UNSPECIFIED.);
#820=B_SPLINE_CURVE_WITH_KNOTS('',2,(#44030,#44031,#44032),
 .UNSPECIFIED.,.F.,.F.,(3,3),(0.,1.),.UNSPECIFIED.);
#821=B_SPLINE_CURVE_WITH_KNOTS('',2,(#44033,#44034,#44035),
 .UNSPECIFIED.,.F.,.F.,(3,3),(0.,1.),.UNSPECIFIED.);
#822=B_SPLINE_CURVE_WITH_KNOTS('',2,(#44045,#44046,#44047),
 .UNSPECIFIED.,.F.,.F.,(3,3),(0.,1.),.UNSPECIFIED.);
#823=B_SPLINE_CURVE_WITH_KNOTS('',2,(#44051,#44052,#44053),
 .UNSPECIFIED.,.F.,.F.,(3,3),(0.,1.),.UNSPECIFIED.);
#824=B_SPLINE_CURVE_WITH_KNOTS('',2,(#44062,#44063,#44064),
 .UNSPECIFIED.,.F.,.F.,(3,3),(0.,1.),.UNSPECIFIED.);
#825=B_SPLINE_CURVE_WITH_KNOTS('',2,(#44067,#44068,#44069),
 .UNSPECIFIED.,.F.,.F.,(3,3),(0.,1.),.UNSPECIFIED.);
#826=B_SPLINE_CURVE_WITH_KNOTS('',2,(#44083,#44084,#44085),
 .UNSPECIFIED.,.F.,.F.,(3,3),(0.,1.),.UNSPECIFIED.);
#827=B_SPLINE_CURVE_WITH_KNOTS('',2,(#44088,#44089,#44090),
 .UNSPECIFIED.,.F.,.F.,(3,3),(0.,1.),.UNSPECIFIED.);
#828=B_SPLINE_CURVE_WITH_KNOTS('',2,(#44098,#44099,#44100),
 .UNSPECIFIED.,.F.,.F.,(3,3),(0.,1.),.UNSPECIFIED.);
#829=B_SPLINE_CURVE_WITH_KNOTS('',2,(#44103,#44104,#44105),
 .UNSPECIFIED.,.F.,.F.,(3,3),(0.,1.),.UNSPECIFIED.);
#830=B_SPLINE_CURVE_WITH_KNOTS('',2,(#44186,#44187,#44188),
 .UNSPECIFIED.,.F.,.F.,(3,3),(0.,1.),.UNSPECIFIED.);
#831=B_SPLINE_CURVE_WITH_KNOTS('',2,(#44191,#44192,#44193),
 .UNSPECIFIED.,.F.,.F.,(3,3),(0.,1.),.UNSPECIFIED.);
#832=B_SPLINE_CURVE_WITH_KNOTS('',2,(#44201,#44202,#44203),
 .UNSPECIFIED.,.F.,.F.,(3,3),(0.,1.),.UNSPECIFIED.);
#833=B_SPLINE_CURVE_WITH_KNOTS('',2,(#44206,#44207,#44208),
 .UNSPECIFIED.,.F.,.F.,(3,3),(0.,1.),.UNSPECIFIED.);
#834=B_SPLINE_CURVE_WITH_KNOTS('',2,(#44245,#44246,#44247),
 .UNSPECIFIED.,.F.,.F.,(3,3),(0.,1.),.UNSPECIFIED.);
#835=B_SPLINE_CURVE_WITH_KNOTS('',2,(#44251,#44252,#44253),
 .UNSPECIFIED.,.F.,.F.,(3,3),(0.,1.),.UNSPECIFIED.);
#836=B_SPLINE_CURVE_WITH_KNOTS('',2,(#44262,#44263,#44264),
 .UNSPECIFIED.,.F.,.F.,(3,3),(0.,1.),.UNSPECIFIED.);
#837=B_SPLINE_CURVE_WITH_KNOTS('',2,(#44267,#44268,#44269),
 .UNSPECIFIED.,.F.,.F.,(3,3),(0.,1.),.UNSPECIFIED.);
#838=B_SPLINE_CURVE_WITH_KNOTS('',2,(#44277,#44278,#44279),
 .UNSPECIFIED.,.F.,.F.,(3,3),(0.,1.),.UNSPECIFIED.);
#839=B_SPLINE_CURVE_WITH_KNOTS('',2,(#44282,#44283,#44284),
 .UNSPECIFIED.,.F.,.F.,(3,3),(0.,1.),.UNSPECIFIED.);
#840=B_SPLINE_CURVE_WITH_KNOTS('',2,(#44292,#44293,#44294),
 .UNSPECIFIED.,.F.,.F.,(3,3),(0.,1.),.UNSPECIFIED.);
#841=B_SPLINE_CURVE_WITH_KNOTS('',2,(#44297,#44298,#44299),
 .UNSPECIFIED.,.F.,.F.,(3,3),(0.,1.),.UNSPECIFIED.);
#842=B_SPLINE_CURVE_WITH_KNOTS('',2,(#44307,#44308,#44309),
 .UNSPECIFIED.,.F.,.F.,(3,3),(0.,1.),.UNSPECIFIED.);
#843=B_SPLINE_CURVE_WITH_KNOTS('',2,(#44312,#44313,#44314),
 .UNSPECIFIED.,.F.,.F.,(3,3),(0.,1.),.UNSPECIFIED.);
#844=B_SPLINE_CURVE_WITH_KNOTS('',2,(#44322,#44323,#44324),
 .UNSPECIFIED.,.F.,.F.,(3,3),(0.,1.),.UNSPECIFIED.);
#845=B_SPLINE_CURVE_WITH_KNOTS('',2,(#44327,#44328,#44329),
 .UNSPECIFIED.,.F.,.F.,(3,3),(0.,1.),.UNSPECIFIED.);
#846=B_SPLINE_CURVE_WITH_KNOTS('',2,(#44337,#44338,#44339),
 .UNSPECIFIED.,.F.,.F.,(3,3),(0.,1.),.UNSPECIFIED.);
#847=B_SPLINE_CURVE_WITH_KNOTS('',2,(#44342,#44343,#44344),
 .UNSPECIFIED.,.F.,.F.,(3,3),(0.,1.),.UNSPECIFIED.);
#848=B_SPLINE_CURVE_WITH_KNOTS('',2,(#44352,#44353,#44354),
 .UNSPECIFIED.,.F.,.F.,(3,3),(0.,1.),.UNSPECIFIED.);
#849=B_SPLINE_CURVE_WITH_KNOTS('',2,(#44357,#44358,#44359),
 .UNSPECIFIED.,.F.,.F.,(3,3),(0.,1.),.UNSPECIFIED.);
#850=B_SPLINE_CURVE_WITH_KNOTS('',2,(#44367,#44368,#44369),
 .UNSPECIFIED.,.F.,.F.,(3,3),(0.,1.),.UNSPECIFIED.);
#851=B_SPLINE_CURVE_WITH_KNOTS('',2,(#44372,#44373,#44374),
 .UNSPECIFIED.,.F.,.F.,(3,3),(0.,1.),.UNSPECIFIED.);
#852=B_SPLINE_CURVE_WITH_KNOTS('',2,(#44382,#44383,#44384),
 .UNSPECIFIED.,.F.,.F.,(3,3),(0.,1.),.UNSPECIFIED.);
#853=B_SPLINE_CURVE_WITH_KNOTS('',2,(#44387,#44388,#44389),
 .UNSPECIFIED.,.F.,.F.,(3,3),(0.,1.),.UNSPECIFIED.);
#854=B_SPLINE_CURVE_WITH_KNOTS('',2,(#44397,#44398,#44399),
 .UNSPECIFIED.,.F.,.F.,(3,3),(0.,1.),.UNSPECIFIED.);
#855=B_SPLINE_CURVE_WITH_KNOTS('',2,(#44402,#44403,#44404),
 .UNSPECIFIED.,.F.,.F.,(3,3),(0.,1.),.UNSPECIFIED.);
#856=B_SPLINE_CURVE_WITH_KNOTS('',2,(#44418,#44419,#44420),
 .UNSPECIFIED.,.F.,.F.,(3,3),(0.,1.),.UNSPECIFIED.);
#857=B_SPLINE_CURVE_WITH_KNOTS('',2,(#44423,#44424,#44425),
 .UNSPECIFIED.,.F.,.F.,(3,3),(0.,1.),.UNSPECIFIED.);
#858=B_SPLINE_CURVE_WITH_KNOTS('',2,(#44433,#44434,#44435),
 .UNSPECIFIED.,.F.,.F.,(3,3),(0.,1.),.UNSPECIFIED.);
#859=B_SPLINE_CURVE_WITH_KNOTS('',2,(#44438,#44439,#44440),
 .UNSPECIFIED.,.F.,.F.,(3,3),(0.,1.),.UNSPECIFIED.);
#860=B_SPLINE_CURVE_WITH_KNOTS('',2,(#44448,#44449,#44450),
 .UNSPECIFIED.,.F.,.F.,(3,3),(0.,1.),.UNSPECIFIED.);
#861=B_SPLINE_CURVE_WITH_KNOTS('',2,(#44453,#44454,#44455),
 .UNSPECIFIED.,.F.,.F.,(3,3),(0.,1.),.UNSPECIFIED.);
#862=B_SPLINE_CURVE_WITH_KNOTS('',2,(#44463,#44464,#44465),
 .UNSPECIFIED.,.F.,.F.,(3,3),(0.,1.),.UNSPECIFIED.);
#863=B_SPLINE_CURVE_WITH_KNOTS('',2,(#44468,#44469,#44470),
 .UNSPECIFIED.,.F.,.F.,(3,3),(0.,1.),.UNSPECIFIED.);
#864=B_SPLINE_CURVE_WITH_KNOTS('',2,(#44478,#44479,#44480),
 .UNSPECIFIED.,.F.,.F.,(3,3),(0.,1.),.UNSPECIFIED.);
#865=B_SPLINE_CURVE_WITH_KNOTS('',2,(#44483,#44484,#44485),
 .UNSPECIFIED.,.F.,.F.,(3,3),(0.,1.),.UNSPECIFIED.);
#866=B_SPLINE_CURVE_WITH_KNOTS('',2,(#44493,#44494,#44495),
 .UNSPECIFIED.,.F.,.F.,(3,3),(0.,1.),.UNSPECIFIED.);
#867=B_SPLINE_CURVE_WITH_KNOTS('',2,(#44498,#44499,#44500),
 .UNSPECIFIED.,.F.,.F.,(3,3),(0.,1.),.UNSPECIFIED.);
#868=B_SPLINE_CURVE_WITH_KNOTS('',2,(#44508,#44509,#44510),
 .UNSPECIFIED.,.F.,.F.,(3,3),(0.,1.),.UNSPECIFIED.);
#869=B_SPLINE_CURVE_WITH_KNOTS('',2,(#44513,#44514,#44515),
 .UNSPECIFIED.,.F.,.F.,(3,3),(0.,1.),.UNSPECIFIED.);
#870=B_SPLINE_CURVE_WITH_KNOTS('',2,(#44529,#44530,#44531),
 .UNSPECIFIED.,.F.,.F.,(3,3),(0.,1.),.UNSPECIFIED.);
#871=B_SPLINE_CURVE_WITH_KNOTS('',2,(#44534,#44535,#44536),
 .UNSPECIFIED.,.F.,.F.,(3,3),(0.,1.),.UNSPECIFIED.);
#872=B_SPLINE_CURVE_WITH_KNOTS('',2,(#44544,#44545,#44546),
 .UNSPECIFIED.,.F.,.F.,(3,3),(0.,1.),.UNSPECIFIED.);
#873=B_SPLINE_CURVE_WITH_KNOTS('',2,(#44549,#44550,#44551),
 .UNSPECIFIED.,.F.,.F.,(3,3),(0.,1.),.UNSPECIFIED.);
#874=B_SPLINE_CURVE_WITH_KNOTS('',2,(#44559,#44560,#44561),
 .UNSPECIFIED.,.F.,.F.,(3,3),(0.,1.),.UNSPECIFIED.);
#875=B_SPLINE_CURVE_WITH_KNOTS('',2,(#44564,#44565,#44566),
 .UNSPECIFIED.,.F.,.F.,(3,3),(0.,1.),.UNSPECIFIED.);
#876=B_SPLINE_CURVE_WITH_KNOTS('',2,(#44574,#44575,#44576),
 .UNSPECIFIED.,.F.,.F.,(3,3),(0.,1.),.UNSPECIFIED.);
#877=B_SPLINE_CURVE_WITH_KNOTS('',2,(#44579,#44580,#44581),
 .UNSPECIFIED.,.F.,.F.,(3,3),(0.,1.),.UNSPECIFIED.);
#878=B_SPLINE_CURVE_WITH_KNOTS('',2,(#44589,#44590,#44591),
 .UNSPECIFIED.,.F.,.F.,(3,3),(0.,1.),.UNSPECIFIED.);
#879=B_SPLINE_CURVE_WITH_KNOTS('',2,(#44594,#44595,#44596),
 .UNSPECIFIED.,.F.,.F.,(3,3),(0.,1.),.UNSPECIFIED.);
#880=B_SPLINE_CURVE_WITH_KNOTS('',2,(#44604,#44605,#44606),
 .UNSPECIFIED.,.F.,.F.,(3,3),(0.,1.),.UNSPECIFIED.);
#881=B_SPLINE_CURVE_WITH_KNOTS('',2,(#44609,#44610,#44611),
 .UNSPECIFIED.,.F.,.F.,(3,3),(0.,1.),.UNSPECIFIED.);
#882=B_SPLINE_CURVE_WITH_KNOTS('',2,(#44619,#44620,#44621),
 .UNSPECIFIED.,.F.,.F.,(3,3),(0.,1.),.UNSPECIFIED.);
#883=B_SPLINE_CURVE_WITH_KNOTS('',2,(#44624,#44625,#44626),
 .UNSPECIFIED.,.F.,.F.,(3,3),(0.,1.),.UNSPECIFIED.);
#884=B_SPLINE_CURVE_WITH_KNOTS('',2,(#44640,#44641,#44642),
 .UNSPECIFIED.,.F.,.F.,(3,3),(0.,1.),.UNSPECIFIED.);
#885=B_SPLINE_CURVE_WITH_KNOTS('',2,(#44645,#44646,#44647),
 .UNSPECIFIED.,.F.,.F.,(3,3),(0.,1.),.UNSPECIFIED.);
#886=B_SPLINE_CURVE_WITH_KNOTS('',2,(#44654,#44655,#44656),
 .UNSPECIFIED.,.F.,.F.,(3,3),(0.,1.),.UNSPECIFIED.);
#887=B_SPLINE_CURVE_WITH_KNOTS('',2,(#44657,#44658,#44659),
 .UNSPECIFIED.,.F.,.F.,(3,3),(0.,1.),.UNSPECIFIED.);
#888=B_SPLINE_CURVE_WITH_KNOTS('',2,(#44694,#44695,#44696),
 .UNSPECIFIED.,.F.,.F.,(3,3),(0.,1.),.UNSPECIFIED.);
#889=B_SPLINE_CURVE_WITH_KNOTS('',2,(#44700,#44701,#44702),
 .UNSPECIFIED.,.F.,.F.,(3,3),(0.,1.),.UNSPECIFIED.);
#890=B_SPLINE_CURVE_WITH_KNOTS('',2,(#44711,#44712,#44713),
 .UNSPECIFIED.,.F.,.F.,(3,3),(0.,1.),.UNSPECIFIED.);
#891=B_SPLINE_CURVE_WITH_KNOTS('',2,(#44716,#44717,#44718),
 .UNSPECIFIED.,.F.,.F.,(3,3),(0.,1.),.UNSPECIFIED.);
#892=B_SPLINE_CURVE_WITH_KNOTS('',2,(#44791,#44792,#44793),
 .UNSPECIFIED.,.F.,.F.,(3,3),(0.,1.),.UNSPECIFIED.);
#893=B_SPLINE_CURVE_WITH_KNOTS('',2,(#44797,#44798,#44799),
 .UNSPECIFIED.,.F.,.F.,(3,3),(0.,1.),.UNSPECIFIED.);
#894=B_SPLINE_CURVE_WITH_KNOTS('',2,(#44808,#44809,#44810),
 .UNSPECIFIED.,.F.,.F.,(3,3),(0.,1.),.UNSPECIFIED.);
#895=B_SPLINE_CURVE_WITH_KNOTS('',2,(#44813,#44814,#44815),
 .UNSPECIFIED.,.F.,.F.,(3,3),(0.,1.),.UNSPECIFIED.);
#896=B_SPLINE_CURVE_WITH_KNOTS('',2,(#44823,#44824,#44825),
 .UNSPECIFIED.,.F.,.F.,(3,3),(0.,1.),.UNSPECIFIED.);
#897=B_SPLINE_CURVE_WITH_KNOTS('',2,(#44828,#44829,#44830),
 .UNSPECIFIED.,.F.,.F.,(3,3),(0.,1.),.UNSPECIFIED.);
#898=B_SPLINE_CURVE_WITH_KNOTS('',2,(#44838,#44839,#44840),
 .UNSPECIFIED.,.F.,.F.,(3,3),(0.,1.),.UNSPECIFIED.);
#899=B_SPLINE_CURVE_WITH_KNOTS('',2,(#44843,#44844,#44845),
 .UNSPECIFIED.,.F.,.F.,(3,3),(0.,1.),.UNSPECIFIED.);
#900=B_SPLINE_CURVE_WITH_KNOTS('',2,(#44853,#44854,#44855),
 .UNSPECIFIED.,.F.,.F.,(3,3),(0.,1.),.UNSPECIFIED.);
#901=B_SPLINE_CURVE_WITH_KNOTS('',2,(#44858,#44859,#44860),
 .UNSPECIFIED.,.F.,.F.,(3,3),(0.,1.),.UNSPECIFIED.);
#902=B_SPLINE_CURVE_WITH_KNOTS('',2,(#44868,#44869,#44870),
 .UNSPECIFIED.,.F.,.F.,(3,3),(0.,1.),.UNSPECIFIED.);
#903=B_SPLINE_CURVE_WITH_KNOTS('',2,(#44873,#44874,#44875),
 .UNSPECIFIED.,.F.,.F.,(3,3),(0.,1.),.UNSPECIFIED.);
#904=B_SPLINE_CURVE_WITH_KNOTS('',2,(#44883,#44884,#44885),
 .UNSPECIFIED.,.F.,.F.,(3,3),(0.,1.),.UNSPECIFIED.);
#905=B_SPLINE_CURVE_WITH_KNOTS('',2,(#44888,#44889,#44890),
 .UNSPECIFIED.,.F.,.F.,(3,3),(0.,1.),.UNSPECIFIED.);
#906=B_SPLINE_CURVE_WITH_KNOTS('',2,(#44898,#44899,#44900),
 .UNSPECIFIED.,.F.,.F.,(3,3),(0.,1.),.UNSPECIFIED.);
#907=B_SPLINE_CURVE_WITH_KNOTS('',2,(#44903,#44904,#44905),
 .UNSPECIFIED.,.F.,.F.,(3,3),(0.,1.),.UNSPECIFIED.);
#908=B_SPLINE_CURVE_WITH_KNOTS('',2,(#44913,#44914,#44915),
 .UNSPECIFIED.,.F.,.F.,(3,3),(0.,1.),.UNSPECIFIED.);
#909=B_SPLINE_CURVE_WITH_KNOTS('',2,(#44918,#44919,#44920),
 .UNSPECIFIED.,.F.,.F.,(3,3),(0.,1.),.UNSPECIFIED.);
#910=B_SPLINE_CURVE_WITH_KNOTS('',2,(#44928,#44929,#44930),
 .UNSPECIFIED.,.F.,.F.,(3,3),(0.,1.),.UNSPECIFIED.);
#911=B_SPLINE_CURVE_WITH_KNOTS('',2,(#44933,#44934,#44935),
 .UNSPECIFIED.,.F.,.F.,(3,3),(0.,1.),.UNSPECIFIED.);
#912=B_SPLINE_CURVE_WITH_KNOTS('',2,(#44943,#44944,#44945),
 .UNSPECIFIED.,.F.,.F.,(3,3),(0.,1.),.UNSPECIFIED.);
#913=B_SPLINE_CURVE_WITH_KNOTS('',2,(#44948,#44949,#44950),
 .UNSPECIFIED.,.F.,.F.,(3,3),(0.,1.),.UNSPECIFIED.);
#914=B_SPLINE_CURVE_WITH_KNOTS('',2,(#44958,#44959,#44960),
 .UNSPECIFIED.,.F.,.F.,(3,3),(0.,1.),.UNSPECIFIED.);
#915=B_SPLINE_CURVE_WITH_KNOTS('',2,(#44963,#44964,#44965),
 .UNSPECIFIED.,.F.,.F.,(3,3),(0.,1.),.UNSPECIFIED.);
#916=B_SPLINE_CURVE_WITH_KNOTS('',2,(#44973,#44974,#44975),
 .UNSPECIFIED.,.F.,.F.,(3,3),(0.,1.),.UNSPECIFIED.);
#917=B_SPLINE_CURVE_WITH_KNOTS('',2,(#44978,#44979,#44980),
 .UNSPECIFIED.,.F.,.F.,(3,3),(0.,1.),.UNSPECIFIED.);
#918=B_SPLINE_CURVE_WITH_KNOTS('',2,(#44994,#44995,#44996),
 .UNSPECIFIED.,.F.,.F.,(3,3),(0.,1.),.UNSPECIFIED.);
#919=B_SPLINE_CURVE_WITH_KNOTS('',2,(#44999,#45000,#45001),
 .UNSPECIFIED.,.F.,.F.,(3,3),(0.,1.),.UNSPECIFIED.);
#920=B_SPLINE_CURVE_WITH_KNOTS('',2,(#45009,#45010,#45011),
 .UNSPECIFIED.,.F.,.F.,(3,3),(0.,1.),.UNSPECIFIED.);
#921=B_SPLINE_CURVE_WITH_KNOTS('',2,(#45014,#45015,#45016),
 .UNSPECIFIED.,.F.,.F.,(3,3),(0.,1.),.UNSPECIFIED.);
#922=B_SPLINE_CURVE_WITH_KNOTS('',2,(#45024,#45025,#45026),
 .UNSPECIFIED.,.F.,.F.,(3,3),(0.,1.),.UNSPECIFIED.);
#923=B_SPLINE_CURVE_WITH_KNOTS('',2,(#45029,#45030,#45031),
 .UNSPECIFIED.,.F.,.F.,(3,3),(0.,1.),.UNSPECIFIED.);
#924=B_SPLINE_CURVE_WITH_KNOTS('',2,(#45039,#45040,#45041),
 .UNSPECIFIED.,.F.,.F.,(3,3),(0.,1.),.UNSPECIFIED.);
#925=B_SPLINE_CURVE_WITH_KNOTS('',2,(#45044,#45045,#45046),
 .UNSPECIFIED.,.F.,.F.,(3,3),(0.,1.),.UNSPECIFIED.);
#926=B_SPLINE_CURVE_WITH_KNOTS('',2,(#45054,#45055,#45056),
 .UNSPECIFIED.,.F.,.F.,(3,3),(0.,1.),.UNSPECIFIED.);
#927=B_SPLINE_CURVE_WITH_KNOTS('',2,(#45059,#45060,#45061),
 .UNSPECIFIED.,.F.,.F.,(3,3),(0.,1.),.UNSPECIFIED.);
#928=B_SPLINE_CURVE_WITH_KNOTS('',2,(#45069,#45070,#45071),
 .UNSPECIFIED.,.F.,.F.,(3,3),(0.,1.),.UNSPECIFIED.);
#929=B_SPLINE_CURVE_WITH_KNOTS('',2,(#45074,#45075,#45076),
 .UNSPECIFIED.,.F.,.F.,(3,3),(0.,1.),.UNSPECIFIED.);
#930=B_SPLINE_CURVE_WITH_KNOTS('',2,(#45084,#45085,#45086),
 .UNSPECIFIED.,.F.,.F.,(3,3),(0.,1.),.UNSPECIFIED.);
#931=B_SPLINE_CURVE_WITH_KNOTS('',2,(#45089,#45090,#45091),
 .UNSPECIFIED.,.F.,.F.,(3,3),(0.,1.),.UNSPECIFIED.);
#932=B_SPLINE_CURVE_WITH_KNOTS('',2,(#45099,#45100,#45101),
 .UNSPECIFIED.,.F.,.F.,(3,3),(0.,1.),.UNSPECIFIED.);
#933=B_SPLINE_CURVE_WITH_KNOTS('',2,(#45104,#45105,#45106),
 .UNSPECIFIED.,.F.,.F.,(3,3),(0.,1.),.UNSPECIFIED.);
#934=B_SPLINE_CURVE_WITH_KNOTS('',2,(#45114,#45115,#45116),
 .UNSPECIFIED.,.F.,.F.,(3,3),(0.,1.),.UNSPECIFIED.);
#935=B_SPLINE_CURVE_WITH_KNOTS('',2,(#45119,#45120,#45121),
 .UNSPECIFIED.,.F.,.F.,(3,3),(0.,1.),.UNSPECIFIED.);
#936=B_SPLINE_CURVE_WITH_KNOTS('',2,(#45129,#45130,#45131),
 .UNSPECIFIED.,.F.,.F.,(3,3),(0.,1.),.UNSPECIFIED.);
#937=B_SPLINE_CURVE_WITH_KNOTS('',2,(#45134,#45135,#45136),
 .UNSPECIFIED.,.F.,.F.,(3,3),(0.,1.),.UNSPECIFIED.);
#938=B_SPLINE_CURVE_WITH_KNOTS('',2,(#45144,#45145,#45146),
 .UNSPECIFIED.,.F.,.F.,(3,3),(0.,1.),.UNSPECIFIED.);
#939=B_SPLINE_CURVE_WITH_KNOTS('',2,(#45149,#45150,#45151),
 .UNSPECIFIED.,.F.,.F.,(3,3),(0.,1.),.UNSPECIFIED.);
#940=B_SPLINE_CURVE_WITH_KNOTS('',2,(#45159,#45160,#45161),
 .UNSPECIFIED.,.F.,.F.,(3,3),(0.,1.),.UNSPECIFIED.);
#941=B_SPLINE_CURVE_WITH_KNOTS('',2,(#45164,#45165,#45166),
 .UNSPECIFIED.,.F.,.F.,(3,3),(0.,1.),.UNSPECIFIED.);
#942=B_SPLINE_CURVE_WITH_KNOTS('',2,(#45174,#45175,#45176),
 .UNSPECIFIED.,.F.,.F.,(3,3),(0.,1.),.UNSPECIFIED.);
#943=B_SPLINE_CURVE_WITH_KNOTS('',2,(#45179,#45180,#45181),
 .UNSPECIFIED.,.F.,.F.,(3,3),(0.,1.),.UNSPECIFIED.);
#944=B_SPLINE_CURVE_WITH_KNOTS('',2,(#45189,#45190,#45191),
 .UNSPECIFIED.,.F.,.F.,(3,3),(0.,1.),.UNSPECIFIED.);
#945=B_SPLINE_CURVE_WITH_KNOTS('',2,(#45194,#45195,#45196),
 .UNSPECIFIED.,.F.,.F.,(3,3),(0.,1.),.UNSPECIFIED.);
#946=B_SPLINE_CURVE_WITH_KNOTS('',2,(#45204,#45205,#45206),
 .UNSPECIFIED.,.F.,.F.,(3,3),(0.,1.),.UNSPECIFIED.);
#947=B_SPLINE_CURVE_WITH_KNOTS('',2,(#45209,#45210,#45211),
 .UNSPECIFIED.,.F.,.F.,(3,3),(0.,1.),.UNSPECIFIED.);
#948=B_SPLINE_CURVE_WITH_KNOTS('',2,(#45219,#45220,#45221),
 .UNSPECIFIED.,.F.,.F.,(3,3),(0.,1.),.UNSPECIFIED.);
#949=B_SPLINE_CURVE_WITH_KNOTS('',2,(#45224,#45225,#45226),
 .UNSPECIFIED.,.F.,.F.,(3,3),(0.,1.),.UNSPECIFIED.);
#950=B_SPLINE_CURVE_WITH_KNOTS('',2,(#45234,#45235,#45236),
 .UNSPECIFIED.,.F.,.F.,(3,3),(0.,1.),.UNSPECIFIED.);
#951=B_SPLINE_CURVE_WITH_KNOTS('',2,(#45239,#45240,#45241),
 .UNSPECIFIED.,.F.,.F.,(3,3),(0.,1.),.UNSPECIFIED.);
#952=B_SPLINE_CURVE_WITH_KNOTS('',2,(#45249,#45250,#45251),
 .UNSPECIFIED.,.F.,.F.,(3,3),(0.,1.),.UNSPECIFIED.);
#953=B_SPLINE_CURVE_WITH_KNOTS('',2,(#45254,#45255,#45256),
 .UNSPECIFIED.,.F.,.F.,(3,3),(0.,1.),.UNSPECIFIED.);
#954=B_SPLINE_CURVE_WITH_KNOTS('',2,(#45270,#45271,#45272),
 .UNSPECIFIED.,.F.,.F.,(3,3),(0.,1.),.UNSPECIFIED.);
#955=B_SPLINE_CURVE_WITH_KNOTS('',2,(#45275,#45276,#45277),
 .UNSPECIFIED.,.F.,.F.,(3,3),(0.,1.),.UNSPECIFIED.);
#956=B_SPLINE_CURVE_WITH_KNOTS('',2,(#45284,#45285,#45286),
 .UNSPECIFIED.,.F.,.F.,(3,3),(0.,1.),.UNSPECIFIED.);
#957=B_SPLINE_CURVE_WITH_KNOTS('',2,(#45287,#45288,#45289),
 .UNSPECIFIED.,.F.,.F.,(3,3),(0.,1.),.UNSPECIFIED.);
#958=B_SPLINE_CURVE_WITH_KNOTS('',2,(#45299,#45300,#45301),
 .UNSPECIFIED.,.F.,.F.,(3,3),(0.,1.),.UNSPECIFIED.);
#959=B_SPLINE_CURVE_WITH_KNOTS('',2,(#45305,#45306,#45307),
 .UNSPECIFIED.,.F.,.F.,(3,3),(0.,1.),.UNSPECIFIED.);
#960=B_SPLINE_CURVE_WITH_KNOTS('',2,(#45316,#45317,#45318),
 .UNSPECIFIED.,.F.,.F.,(3,3),(0.,1.),.UNSPECIFIED.);
#961=B_SPLINE_CURVE_WITH_KNOTS('',2,(#45321,#45322,#45323),
 .UNSPECIFIED.,.F.,.F.,(3,3),(0.,1.),.UNSPECIFIED.);
#962=B_SPLINE_CURVE_WITH_KNOTS('',2,(#45331,#45332,#45333),
 .UNSPECIFIED.,.F.,.F.,(3,3),(0.,1.),.UNSPECIFIED.);
#963=B_SPLINE_CURVE_WITH_KNOTS('',2,(#45336,#45337,#45338),
 .UNSPECIFIED.,.F.,.F.,(3,3),(0.,1.),.UNSPECIFIED.);
#964=B_SPLINE_CURVE_WITH_KNOTS('',2,(#45346,#45347,#45348),
 .UNSPECIFIED.,.F.,.F.,(3,3),(0.,1.),.UNSPECIFIED.);
#965=B_SPLINE_CURVE_WITH_KNOTS('',2,(#45351,#45352,#45353),
 .UNSPECIFIED.,.F.,.F.,(3,3),(0.,1.),.UNSPECIFIED.);
#966=B_SPLINE_CURVE_WITH_KNOTS('',2,(#45361,#45362,#45363),
 .UNSPECIFIED.,.F.,.F.,(3,3),(0.,1.),.UNSPECIFIED.);
#967=B_SPLINE_CURVE_WITH_KNOTS('',2,(#45366,#45367,#45368),
 .UNSPECIFIED.,.F.,.F.,(3,3),(0.,1.),.UNSPECIFIED.);
#968=B_SPLINE_CURVE_WITH_KNOTS('',2,(#45376,#45377,#45378),
 .UNSPECIFIED.,.F.,.F.,(3,3),(0.,1.),.UNSPECIFIED.);
#969=B_SPLINE_CURVE_WITH_KNOTS('',2,(#45381,#45382,#45383),
 .UNSPECIFIED.,.F.,.F.,(3,3),(0.,1.),.UNSPECIFIED.);
#970=B_SPLINE_CURVE_WITH_KNOTS('',2,(#45391,#45392,#45393),
 .UNSPECIFIED.,.F.,.F.,(3,3),(0.,1.),.UNSPECIFIED.);
#971=B_SPLINE_CURVE_WITH_KNOTS('',2,(#45396,#45397,#45398),
 .UNSPECIFIED.,.F.,.F.,(3,3),(0.,1.),.UNSPECIFIED.);
#972=B_SPLINE_CURVE_WITH_KNOTS('',2,(#45406,#45407,#45408),
 .UNSPECIFIED.,.F.,.F.,(3,3),(0.,1.),.UNSPECIFIED.);
#973=B_SPLINE_CURVE_WITH_KNOTS('',2,(#45411,#45412,#45413),
 .UNSPECIFIED.,.F.,.F.,(3,3),(0.,1.),.UNSPECIFIED.);
#974=B_SPLINE_CURVE_WITH_KNOTS('',2,(#45421,#45422,#45423),
 .UNSPECIFIED.,.F.,.F.,(3,3),(0.,1.),.UNSPECIFIED.);
#975=B_SPLINE_CURVE_WITH_KNOTS('',2,(#45426,#45427,#45428),
 .UNSPECIFIED.,.F.,.F.,(3,3),(0.,1.),.UNSPECIFIED.);
#976=B_SPLINE_CURVE_WITH_KNOTS('',2,(#45436,#45437,#45438),
 .UNSPECIFIED.,.F.,.F.,(3,3),(0.,1.),.UNSPECIFIED.);
#977=B_SPLINE_CURVE_WITH_KNOTS('',2,(#45441,#45442,#45443),
 .UNSPECIFIED.,.F.,.F.,(3,3),(0.,1.),.UNSPECIFIED.);
#978=B_SPLINE_CURVE_WITH_KNOTS('',2,(#45451,#45452,#45453),
 .UNSPECIFIED.,.F.,.F.,(3,3),(0.,1.),.UNSPECIFIED.);
#979=B_SPLINE_CURVE_WITH_KNOTS('',2,(#45456,#45457,#45458),
 .UNSPECIFIED.,.F.,.F.,(3,3),(0.,1.),.UNSPECIFIED.);
#980=B_SPLINE_CURVE_WITH_KNOTS('',2,(#45472,#45473,#45474),
 .UNSPECIFIED.,.F.,.F.,(3,3),(0.,1.),.UNSPECIFIED.);
#981=B_SPLINE_CURVE_WITH_KNOTS('',2,(#45477,#45478,#45479),
 .UNSPECIFIED.,.F.,.F.,(3,3),(0.,1.),.UNSPECIFIED.);
#982=B_SPLINE_CURVE_WITH_KNOTS('',2,(#45487,#45488,#45489),
 .UNSPECIFIED.,.F.,.F.,(3,3),(0.,1.),.UNSPECIFIED.);
#983=B_SPLINE_CURVE_WITH_KNOTS('',2,(#45492,#45493,#45494),
 .UNSPECIFIED.,.F.,.F.,(3,3),(0.,1.),.UNSPECIFIED.);
#984=B_SPLINE_CURVE_WITH_KNOTS('',2,(#45502,#45503,#45504),
 .UNSPECIFIED.,.F.,.F.,(3,3),(0.,1.),.UNSPECIFIED.);
#985=B_SPLINE_CURVE_WITH_KNOTS('',2,(#45507,#45508,#45509),
 .UNSPECIFIED.,.F.,.F.,(3,3),(0.,1.),.UNSPECIFIED.);
#986=B_SPLINE_CURVE_WITH_KNOTS('',2,(#45517,#45518,#45519),
 .UNSPECIFIED.,.F.,.F.,(3,3),(0.,1.),.UNSPECIFIED.);
#987=B_SPLINE_CURVE_WITH_KNOTS('',2,(#45522,#45523,#45524),
 .UNSPECIFIED.,.F.,.F.,(3,3),(0.,1.),.UNSPECIFIED.);
#988=B_SPLINE_CURVE_WITH_KNOTS('',2,(#45532,#45533,#45534),
 .UNSPECIFIED.,.F.,.F.,(3,3),(0.,1.),.UNSPECIFIED.);
#989=B_SPLINE_CURVE_WITH_KNOTS('',2,(#45537,#45538,#45539),
 .UNSPECIFIED.,.F.,.F.,(3,3),(0.,1.),.UNSPECIFIED.);
#990=B_SPLINE_CURVE_WITH_KNOTS('',2,(#45547,#45548,#45549),
 .UNSPECIFIED.,.F.,.F.,(3,3),(0.,1.),.UNSPECIFIED.);
#991=B_SPLINE_CURVE_WITH_KNOTS('',2,(#45552,#45553,#45554),
 .UNSPECIFIED.,.F.,.F.,(3,3),(0.,1.),.UNSPECIFIED.);
#992=B_SPLINE_CURVE_WITH_KNOTS('',2,(#45562,#45563,#45564),
 .UNSPECIFIED.,.F.,.F.,(3,3),(0.,1.),.UNSPECIFIED.);
#993=B_SPLINE_CURVE_WITH_KNOTS('',2,(#45567,#45568,#45569),
 .UNSPECIFIED.,.F.,.F.,(3,3),(0.,1.),.UNSPECIFIED.);
#994=B_SPLINE_CURVE_WITH_KNOTS('',2,(#45583,#45584,#45585),
 .UNSPECIFIED.,.F.,.F.,(3,3),(0.,1.),.UNSPECIFIED.);
#995=B_SPLINE_CURVE_WITH_KNOTS('',2,(#45588,#45589,#45590),
 .UNSPECIFIED.,.F.,.F.,(3,3),(0.,1.),.UNSPECIFIED.);
#996=B_SPLINE_CURVE_WITH_KNOTS('',2,(#45598,#45599,#45600),
 .UNSPECIFIED.,.F.,.F.,(3,3),(0.,1.),.UNSPECIFIED.);
#997=B_SPLINE_CURVE_WITH_KNOTS('',2,(#45603,#45604,#45605),
 .UNSPECIFIED.,.F.,.F.,(3,3),(0.,1.),.UNSPECIFIED.);
#998=B_SPLINE_CURVE_WITH_KNOTS('',2,(#45613,#45614,#45615),
 .UNSPECIFIED.,.F.,.F.,(3,3),(0.,1.),.UNSPECIFIED.);
#999=B_SPLINE_CURVE_WITH_KNOTS('',2,(#45618,#45619,#45620),
 .UNSPECIFIED.,.F.,.F.,(3,3),(0.,1.),.UNSPECIFIED.);
#1000=B_SPLINE_CURVE_WITH_KNOTS('',2,(#45628,#45629,#45630),
 .UNSPECIFIED.,.F.,.F.,(3,3),(0.,1.),.UNSPECIFIED.);
#1001=B_SPLINE_CURVE_WITH_KNOTS('',2,(#45633,#45634,#45635),
 .UNSPECIFIED.,.F.,.F.,(3,3),(0.,1.),.UNSPECIFIED.);
#1002=B_SPLINE_CURVE_WITH_KNOTS('',2,(#45643,#45644,#45645),
 .UNSPECIFIED.,.F.,.F.,(3,3),(0.,1.),.UNSPECIFIED.);
#1003=B_SPLINE_CURVE_WITH_KNOTS('',2,(#45648,#45649,#45650),
 .UNSPECIFIED.,.F.,.F.,(3,3),(0.,1.),.UNSPECIFIED.);
#1004=B_SPLINE_CURVE_WITH_KNOTS('',2,(#45658,#45659,#45660),
 .UNSPECIFIED.,.F.,.F.,(3,3),(0.,1.),.UNSPECIFIED.);
#1005=B_SPLINE_CURVE_WITH_KNOTS('',2,(#45663,#45664,#45665),
 .UNSPECIFIED.,.F.,.F.,(3,3),(0.,1.),.UNSPECIFIED.);
#1006=B_SPLINE_CURVE_WITH_KNOTS('',2,(#45673,#45674,#45675),
 .UNSPECIFIED.,.F.,.F.,(3,3),(0.,1.),.UNSPECIFIED.);
#1007=B_SPLINE_CURVE_WITH_KNOTS('',2,(#45678,#45679,#45680),
 .UNSPECIFIED.,.F.,.F.,(3,3),(0.,1.),.UNSPECIFIED.);
#1008=B_SPLINE_CURVE_WITH_KNOTS('',2,(#45694,#45695,#45696),
 .UNSPECIFIED.,.F.,.F.,(3,3),(0.,1.),.UNSPECIFIED.);
#1009=B_SPLINE_CURVE_WITH_KNOTS('',2,(#45699,#45700,#45701),
 .UNSPECIFIED.,.F.,.F.,(3,3),(0.,1.),.UNSPECIFIED.);
#1010=B_SPLINE_CURVE_WITH_KNOTS('',2,(#45708,#45709,#45710),
 .UNSPECIFIED.,.F.,.F.,(3,3),(0.,1.),.UNSPECIFIED.);
#1011=B_SPLINE_CURVE_WITH_KNOTS('',2,(#45711,#45712,#45713),
 .UNSPECIFIED.,.F.,.F.,(3,3),(0.,1.),.UNSPECIFIED.);
#1012=B_SPLINE_CURVE_WITH_KNOTS('',2,(#45723,#45724,#45725),
 .UNSPECIFIED.,.F.,.F.,(3,3),(0.,1.),.UNSPECIFIED.);
#1013=B_SPLINE_CURVE_WITH_KNOTS('',2,(#45729,#45730,#45731),
 .UNSPECIFIED.,.F.,.F.,(3,3),(0.,1.),.UNSPECIFIED.);
#1014=B_SPLINE_CURVE_WITH_KNOTS('',2,(#45740,#45741,#45742),
 .UNSPECIFIED.,.F.,.F.,(3,3),(0.,1.),.UNSPECIFIED.);
#1015=B_SPLINE_CURVE_WITH_KNOTS('',2,(#45745,#45746,#45747),
 .UNSPECIFIED.,.F.,.F.,(3,3),(0.,1.),.UNSPECIFIED.);
#1016=B_SPLINE_CURVE_WITH_KNOTS('',2,(#45755,#45756,#45757),
 .UNSPECIFIED.,.F.,.F.,(3,3),(0.,1.),.UNSPECIFIED.);
#1017=B_SPLINE_CURVE_WITH_KNOTS('',2,(#45760,#45761,#45762),
 .UNSPECIFIED.,.F.,.F.,(3,3),(0.,1.),.UNSPECIFIED.);
#1018=B_SPLINE_CURVE_WITH_KNOTS('',2,(#45770,#45771,#45772),
 .UNSPECIFIED.,.F.,.F.,(3,3),(0.,1.),.UNSPECIFIED.);
#1019=B_SPLINE_CURVE_WITH_KNOTS('',2,(#45775,#45776,#45777),
 .UNSPECIFIED.,.F.,.F.,(3,3),(0.,1.),.UNSPECIFIED.);
#1020=B_SPLINE_CURVE_WITH_KNOTS('',2,(#45785,#45786,#45787),
 .UNSPECIFIED.,.F.,.F.,(3,3),(0.,1.),.UNSPECIFIED.);
#1021=B_SPLINE_CURVE_WITH_KNOTS('',2,(#45790,#45791,#45792),
 .UNSPECIFIED.,.F.,.F.,(3,3),(0.,1.),.UNSPECIFIED.);
#1022=B_SPLINE_CURVE_WITH_KNOTS('',2,(#45800,#45801,#45802),
 .UNSPECIFIED.,.F.,.F.,(3,3),(0.,1.),.UNSPECIFIED.);
#1023=B_SPLINE_CURVE_WITH_KNOTS('',2,(#45805,#45806,#45807),
 .UNSPECIFIED.,.F.,.F.,(3,3),(0.,1.),.UNSPECIFIED.);
#1024=B_SPLINE_CURVE_WITH_KNOTS('',2,(#45815,#45816,#45817),
 .UNSPECIFIED.,.F.,.F.,(3,3),(0.,1.),.UNSPECIFIED.);
#1025=B_SPLINE_CURVE_WITH_KNOTS('',2,(#45820,#45821,#45822),
 .UNSPECIFIED.,.F.,.F.,(3,3),(0.,1.),.UNSPECIFIED.);
#1026=B_SPLINE_CURVE_WITH_KNOTS('',2,(#45830,#45831,#45832),
 .UNSPECIFIED.,.F.,.F.,(3,3),(0.,1.),.UNSPECIFIED.);
#1027=B_SPLINE_CURVE_WITH_KNOTS('',2,(#45835,#45836,#45837),
 .UNSPECIFIED.,.F.,.F.,(3,3),(0.,1.),.UNSPECIFIED.);
#1028=B_SPLINE_CURVE_WITH_KNOTS('',2,(#45851,#45852,#45853),
 .UNSPECIFIED.,.F.,.F.,(3,3),(0.,1.),.UNSPECIFIED.);
#1029=B_SPLINE_CURVE_WITH_KNOTS('',2,(#45856,#45857,#45858),
 .UNSPECIFIED.,.F.,.F.,(3,3),(0.,1.),.UNSPECIFIED.);
#1030=B_SPLINE_CURVE_WITH_KNOTS('',2,(#45866,#45867,#45868),
 .UNSPECIFIED.,.F.,.F.,(3,3),(0.,1.),.UNSPECIFIED.);
#1031=B_SPLINE_CURVE_WITH_KNOTS('',2,(#45871,#45872,#45873),
 .UNSPECIFIED.,.F.,.F.,(3,3),(0.,1.),.UNSPECIFIED.);
#1032=B_SPLINE_CURVE_WITH_KNOTS('',2,(#45881,#45882,#45883),
 .UNSPECIFIED.,.F.,.F.,(3,3),(0.,1.),.UNSPECIFIED.);
#1033=B_SPLINE_CURVE_WITH_KNOTS('',2,(#45886,#45887,#45888),
 .UNSPECIFIED.,.F.,.F.,(3,3),(0.,1.),.UNSPECIFIED.);
#1034=B_SPLINE_CURVE_WITH_KNOTS('',2,(#45896,#45897,#45898),
 .UNSPECIFIED.,.F.,.F.,(3,3),(0.,1.),.UNSPECIFIED.);
#1035=B_SPLINE_CURVE_WITH_KNOTS('',2,(#45901,#45902,#45903),
 .UNSPECIFIED.,.F.,.F.,(3,3),(0.,1.),.UNSPECIFIED.);
#1036=B_SPLINE_CURVE_WITH_KNOTS('',2,(#45911,#45912,#45913),
 .UNSPECIFIED.,.F.,.F.,(3,3),(0.,1.),.UNSPECIFIED.);
#1037=B_SPLINE_CURVE_WITH_KNOTS('',2,(#45916,#45917,#45918),
 .UNSPECIFIED.,.F.,.F.,(3,3),(0.,1.),.UNSPECIFIED.);
#1038=B_SPLINE_CURVE_WITH_KNOTS('',2,(#45926,#45927,#45928),
 .UNSPECIFIED.,.F.,.F.,(3,3),(0.,1.),.UNSPECIFIED.);
#1039=B_SPLINE_CURVE_WITH_KNOTS('',2,(#45931,#45932,#45933),
 .UNSPECIFIED.,.F.,.F.,(3,3),(0.,1.),.UNSPECIFIED.);
#1040=B_SPLINE_CURVE_WITH_KNOTS('',2,(#45941,#45942,#45943),
 .UNSPECIFIED.,.F.,.F.,(3,3),(0.,1.),.UNSPECIFIED.);
#1041=B_SPLINE_CURVE_WITH_KNOTS('',2,(#45946,#45947,#45948),
 .UNSPECIFIED.,.F.,.F.,(3,3),(0.,1.),.UNSPECIFIED.);
#1042=B_SPLINE_CURVE_WITH_KNOTS('',2,(#45956,#45957,#45958),
 .UNSPECIFIED.,.F.,.F.,(3,3),(0.,1.),.UNSPECIFIED.);
#1043=B_SPLINE_CURVE_WITH_KNOTS('',2,(#45961,#45962,#45963),
 .UNSPECIFIED.,.F.,.F.,(3,3),(0.,1.),.UNSPECIFIED.);
#1044=B_SPLINE_CURVE_WITH_KNOTS('',2,(#45971,#45972,#45973),
 .UNSPECIFIED.,.F.,.F.,(3,3),(0.,1.),.UNSPECIFIED.);
#1045=B_SPLINE_CURVE_WITH_KNOTS('',2,(#45976,#45977,#45978),
 .UNSPECIFIED.,.F.,.F.,(3,3),(0.,1.),.UNSPECIFIED.);
#1046=B_SPLINE_CURVE_WITH_KNOTS('',2,(#46003,#46004,#46005),
 .UNSPECIFIED.,.F.,.F.,(3,3),(0.,1.),.UNSPECIFIED.);
#1047=B_SPLINE_CURVE_WITH_KNOTS('',2,(#46006,#46007,#46008),
 .UNSPECIFIED.,.F.,.F.,(3,3),(0.,1.),.UNSPECIFIED.);
#1048=B_SPLINE_CURVE_WITH_KNOTS('',2,(#46026,#46027,#46028),
 .UNSPECIFIED.,.F.,.F.,(3,3),(0.,1.),.UNSPECIFIED.);
#1049=B_SPLINE_CURVE_WITH_KNOTS('',2,(#46031,#46032,#46033),
 .UNSPECIFIED.,.F.,.F.,(3,3),(0.,1.),.UNSPECIFIED.);
#1050=B_SPLINE_CURVE_WITH_KNOTS('',2,(#46041,#46042,#46043),
 .UNSPECIFIED.,.F.,.F.,(3,3),(0.,1.),.UNSPECIFIED.);
#1051=B_SPLINE_CURVE_WITH_KNOTS('',2,(#46046,#46047,#46048),
 .UNSPECIFIED.,.F.,.F.,(3,3),(0.,1.),.UNSPECIFIED.);
#1052=B_SPLINE_CURVE_WITH_KNOTS('',2,(#46056,#46057,#46058),
 .UNSPECIFIED.,.F.,.F.,(3,3),(0.,1.),.UNSPECIFIED.);
#1053=B_SPLINE_CURVE_WITH_KNOTS('',2,(#46061,#46062,#46063),
 .UNSPECIFIED.,.F.,.F.,(3,3),(0.,1.),.UNSPECIFIED.);
#1054=B_SPLINE_CURVE_WITH_KNOTS('',2,(#46071,#46072,#46073),
 .UNSPECIFIED.,.F.,.F.,(3,3),(0.,1.),.UNSPECIFIED.);
#1055=B_SPLINE_CURVE_WITH_KNOTS('',2,(#46076,#46077,#46078),
 .UNSPECIFIED.,.F.,.F.,(3,3),(0.,1.),.UNSPECIFIED.);
#1056=B_SPLINE_CURVE_WITH_KNOTS('',2,(#46086,#46087,#46088),
 .UNSPECIFIED.,.F.,.F.,(3,3),(0.,1.),.UNSPECIFIED.);
#1057=B_SPLINE_CURVE_WITH_KNOTS('',2,(#46091,#46092,#46093),
 .UNSPECIFIED.,.F.,.F.,(3,3),(0.,1.),.UNSPECIFIED.);
#1058=B_SPLINE_CURVE_WITH_KNOTS('',2,(#46119,#46120,#46121),
 .UNSPECIFIED.,.F.,.F.,(3,3),(0.,1.),.UNSPECIFIED.);
#1059=B_SPLINE_CURVE_WITH_KNOTS('',2,(#46124,#46125,#46126),
 .UNSPECIFIED.,.F.,.F.,(3,3),(0.,1.),.UNSPECIFIED.);
#1060=B_SPLINE_CURVE_WITH_KNOTS('',2,(#46134,#46135,#46136),
 .UNSPECIFIED.,.F.,.F.,(3,3),(0.,1.),.UNSPECIFIED.);
#1061=B_SPLINE_CURVE_WITH_KNOTS('',2,(#46139,#46140,#46141),
 .UNSPECIFIED.,.F.,.F.,(3,3),(0.,1.),.UNSPECIFIED.);
#1062=B_SPLINE_CURVE_WITH_KNOTS('',2,(#46149,#46150,#46151),
 .UNSPECIFIED.,.F.,.F.,(3,3),(0.,1.),.UNSPECIFIED.);
#1063=B_SPLINE_CURVE_WITH_KNOTS('',2,(#46154,#46155,#46156),
 .UNSPECIFIED.,.F.,.F.,(3,3),(0.,1.),.UNSPECIFIED.);
#1064=B_SPLINE_CURVE_WITH_KNOTS('',2,(#46164,#46165,#46166),
 .UNSPECIFIED.,.F.,.F.,(3,3),(0.,1.),.UNSPECIFIED.);
#1065=B_SPLINE_CURVE_WITH_KNOTS('',2,(#46169,#46170,#46171),
 .UNSPECIFIED.,.F.,.F.,(3,3),(0.,1.),.UNSPECIFIED.);
#1066=B_SPLINE_CURVE_WITH_KNOTS('',2,(#46179,#46180,#46181),
 .UNSPECIFIED.,.F.,.F.,(3,3),(0.,1.),.UNSPECIFIED.);
#1067=B_SPLINE_CURVE_WITH_KNOTS('',2,(#46184,#46185,#46186),
 .UNSPECIFIED.,.F.,.F.,(3,3),(0.,1.),.UNSPECIFIED.);
#1068=B_SPLINE_CURVE_WITH_KNOTS('',2,(#46194,#46195,#46196),
 .UNSPECIFIED.,.F.,.F.,(3,3),(0.,1.),.UNSPECIFIED.);
#1069=B_SPLINE_CURVE_WITH_KNOTS('',2,(#46199,#46200,#46201),
 .UNSPECIFIED.,.F.,.F.,(3,3),(0.,1.),.UNSPECIFIED.);
#1070=B_SPLINE_CURVE_WITH_KNOTS('',2,(#46232,#46233,#46234),
 .UNSPECIFIED.,.F.,.F.,(3,3),(0.,1.),.UNSPECIFIED.);
#1071=B_SPLINE_CURVE_WITH_KNOTS('',2,(#46238,#46239,#46240),
 .UNSPECIFIED.,.F.,.F.,(3,3),(0.,1.),.UNSPECIFIED.);
#1072=B_SPLINE_CURVE_WITH_KNOTS('',2,(#46249,#46250,#46251),
 .UNSPECIFIED.,.F.,.F.,(3,3),(0.,1.),.UNSPECIFIED.);
#1073=B_SPLINE_CURVE_WITH_KNOTS('',2,(#46254,#46255,#46256),
 .UNSPECIFIED.,.F.,.F.,(3,3),(0.,1.),.UNSPECIFIED.);
#1074=B_SPLINE_CURVE_WITH_KNOTS('',2,(#46264,#46265,#46266),
 .UNSPECIFIED.,.F.,.F.,(3,3),(0.,1.),.UNSPECIFIED.);
#1075=B_SPLINE_CURVE_WITH_KNOTS('',2,(#46269,#46270,#46271),
 .UNSPECIFIED.,.F.,.F.,(3,3),(0.,1.),.UNSPECIFIED.);
#1076=B_SPLINE_CURVE_WITH_KNOTS('',2,(#46279,#46280,#46281),
 .UNSPECIFIED.,.F.,.F.,(3,3),(0.,1.),.UNSPECIFIED.);
#1077=B_SPLINE_CURVE_WITH_KNOTS('',2,(#46284,#46285,#46286),
 .UNSPECIFIED.,.F.,.F.,(3,3),(0.,1.),.UNSPECIFIED.);
#1078=B_SPLINE_CURVE_WITH_KNOTS('',2,(#46294,#46295,#46296),
 .UNSPECIFIED.,.F.,.F.,(3,3),(0.,1.),.UNSPECIFIED.);
#1079=B_SPLINE_CURVE_WITH_KNOTS('',2,(#46299,#46300,#46301),
 .UNSPECIFIED.,.F.,.F.,(3,3),(0.,1.),.UNSPECIFIED.);
#1080=B_SPLINE_CURVE_WITH_KNOTS('',2,(#46309,#46310,#46311),
 .UNSPECIFIED.,.F.,.F.,(3,3),(0.,1.),.UNSPECIFIED.);
#1081=B_SPLINE_CURVE_WITH_KNOTS('',2,(#46314,#46315,#46316),
 .UNSPECIFIED.,.F.,.F.,(3,3),(0.,1.),.UNSPECIFIED.);
#1082=B_SPLINE_CURVE_WITH_KNOTS('',2,(#46324,#46325,#46326),
 .UNSPECIFIED.,.F.,.F.,(3,3),(0.,1.),.UNSPECIFIED.);
#1083=B_SPLINE_CURVE_WITH_KNOTS('',2,(#46329,#46330,#46331),
 .UNSPECIFIED.,.F.,.F.,(3,3),(0.,1.),.UNSPECIFIED.);
#1084=B_SPLINE_CURVE_WITH_KNOTS('',2,(#46339,#46340,#46341),
 .UNSPECIFIED.,.F.,.F.,(3,3),(0.,1.),.UNSPECIFIED.);
#1085=B_SPLINE_CURVE_WITH_KNOTS('',2,(#46344,#46345,#46346),
 .UNSPECIFIED.,.F.,.F.,(3,3),(0.,1.),.UNSPECIFIED.);
#1086=B_SPLINE_CURVE_WITH_KNOTS('',2,(#46353,#46354,#46355),
 .UNSPECIFIED.,.F.,.F.,(3,3),(0.,1.),.UNSPECIFIED.);
#1087=B_SPLINE_CURVE_WITH_KNOTS('',2,(#46356,#46357,#46358),
 .UNSPECIFIED.,.F.,.F.,(3,3),(0.,1.),.UNSPECIFIED.);
#1088=B_SPLINE_CURVE_WITH_KNOTS('',2,(#46367,#46368,#46369),
 .UNSPECIFIED.,.F.,.F.,(3,3),(0.,1.),.UNSPECIFIED.);
#1089=B_SPLINE_CURVE_WITH_KNOTS('',2,(#46373,#46374,#46375),
 .UNSPECIFIED.,.F.,.F.,(3,3),(0.,1.),.UNSPECIFIED.);
#1090=B_SPLINE_CURVE_WITH_KNOTS('',2,(#46384,#46385,#46386),
 .UNSPECIFIED.,.F.,.F.,(3,3),(0.,1.),.UNSPECIFIED.);
#1091=B_SPLINE_CURVE_WITH_KNOTS('',2,(#46389,#46390,#46391),
 .UNSPECIFIED.,.F.,.F.,(3,3),(0.,1.),.UNSPECIFIED.);
#1092=B_SPLINE_CURVE_WITH_KNOTS('',2,(#46399,#46400,#46401),
 .UNSPECIFIED.,.F.,.F.,(3,3),(0.,1.),.UNSPECIFIED.);
#1093=B_SPLINE_CURVE_WITH_KNOTS('',2,(#46404,#46405,#46406),
 .UNSPECIFIED.,.F.,.F.,(3,3),(0.,1.),.UNSPECIFIED.);
#1094=B_SPLINE_CURVE_WITH_KNOTS('',2,(#46414,#46415,#46416),
 .UNSPECIFIED.,.F.,.F.,(3,3),(0.,1.),.UNSPECIFIED.);
#1095=B_SPLINE_CURVE_WITH_KNOTS('',2,(#46419,#46420,#46421),
 .UNSPECIFIED.,.F.,.F.,(3,3),(0.,1.),.UNSPECIFIED.);
#1096=B_SPLINE_CURVE_WITH_KNOTS('',2,(#46429,#46430,#46431),
 .UNSPECIFIED.,.F.,.F.,(3,3),(0.,1.),.UNSPECIFIED.);
#1097=B_SPLINE_CURVE_WITH_KNOTS('',2,(#46434,#46435,#46436),
 .UNSPECIFIED.,.F.,.F.,(3,3),(0.,1.),.UNSPECIFIED.);
#1098=B_SPLINE_CURVE_WITH_KNOTS('',2,(#46444,#46445,#46446),
 .UNSPECIFIED.,.F.,.F.,(3,3),(0.,1.),.UNSPECIFIED.);
#1099=B_SPLINE_CURVE_WITH_KNOTS('',2,(#46449,#46450,#46451),
 .UNSPECIFIED.,.F.,.F.,(3,3),(0.,1.),.UNSPECIFIED.);
#1100=B_SPLINE_CURVE_WITH_KNOTS('',2,(#46459,#46460,#46461),
 .UNSPECIFIED.,.F.,.F.,(3,3),(0.,1.),.UNSPECIFIED.);
#1101=B_SPLINE_CURVE_WITH_KNOTS('',2,(#46464,#46465,#46466),
 .UNSPECIFIED.,.F.,.F.,(3,3),(0.,1.),.UNSPECIFIED.);
#1102=B_SPLINE_CURVE_WITH_KNOTS('',2,(#46474,#46475,#46476),
 .UNSPECIFIED.,.F.,.F.,(3,3),(0.,1.),.UNSPECIFIED.);
#1103=B_SPLINE_CURVE_WITH_KNOTS('',2,(#46479,#46480,#46481),
 .UNSPECIFIED.,.F.,.F.,(3,3),(0.,1.),.UNSPECIFIED.);
#1104=B_SPLINE_CURVE_WITH_KNOTS('',2,(#46489,#46490,#46491),
 .UNSPECIFIED.,.F.,.F.,(3,3),(0.,1.),.UNSPECIFIED.);
#1105=B_SPLINE_CURVE_WITH_KNOTS('',2,(#46494,#46495,#46496),
 .UNSPECIFIED.,.F.,.F.,(3,3),(0.,1.),.UNSPECIFIED.);
#1106=B_SPLINE_CURVE_WITH_KNOTS('',2,(#46504,#46505,#46506),
 .UNSPECIFIED.,.F.,.F.,(3,3),(0.,1.),.UNSPECIFIED.);
#1107=B_SPLINE_CURVE_WITH_KNOTS('',2,(#46509,#46510,#46511),
 .UNSPECIFIED.,.F.,.F.,(3,3),(0.,1.),.UNSPECIFIED.);
#1108=B_SPLINE_CURVE_WITH_KNOTS('',2,(#46519,#46520,#46521),
 .UNSPECIFIED.,.F.,.F.,(3,3),(0.,1.),.UNSPECIFIED.);
#1109=B_SPLINE_CURVE_WITH_KNOTS('',2,(#46524,#46525,#46526),
 .UNSPECIFIED.,.F.,.F.,(3,3),(0.,1.),.UNSPECIFIED.);
#1110=B_SPLINE_CURVE_WITH_KNOTS('',2,(#46534,#46535,#46536),
 .UNSPECIFIED.,.F.,.F.,(3,3),(0.,1.),.UNSPECIFIED.);
#1111=B_SPLINE_CURVE_WITH_KNOTS('',2,(#46539,#46540,#46541),
 .UNSPECIFIED.,.F.,.F.,(3,3),(0.,1.),.UNSPECIFIED.);
#1112=B_SPLINE_CURVE_WITH_KNOTS('',2,(#46549,#46550,#46551),
 .UNSPECIFIED.,.F.,.F.,(3,3),(0.,1.),.UNSPECIFIED.);
#1113=B_SPLINE_CURVE_WITH_KNOTS('',2,(#46554,#46555,#46556),
 .UNSPECIFIED.,.F.,.F.,(3,3),(0.,1.),.UNSPECIFIED.);
#1114=B_SPLINE_CURVE_WITH_KNOTS('',2,(#46564,#46565,#46566),
 .UNSPECIFIED.,.F.,.F.,(3,3),(0.,1.),.UNSPECIFIED.);
#1115=B_SPLINE_CURVE_WITH_KNOTS('',2,(#46569,#46570,#46571),
 .UNSPECIFIED.,.F.,.F.,(3,3),(0.,1.),.UNSPECIFIED.);
#1116=B_SPLINE_CURVE_WITH_KNOTS('',2,(#46579,#46580,#46581),
 .UNSPECIFIED.,.F.,.F.,(3,3),(0.,1.),.UNSPECIFIED.);
#1117=B_SPLINE_CURVE_WITH_KNOTS('',2,(#46584,#46585,#46586),
 .UNSPECIFIED.,.F.,.F.,(3,3),(0.,1.),.UNSPECIFIED.);
#1118=B_SPLINE_CURVE_WITH_KNOTS('',2,(#46594,#46595,#46596),
 .UNSPECIFIED.,.F.,.F.,(3,3),(0.,1.),.UNSPECIFIED.);
#1119=B_SPLINE_CURVE_WITH_KNOTS('',2,(#46599,#46600,#46601),
 .UNSPECIFIED.,.F.,.F.,(3,3),(0.,1.),.UNSPECIFIED.);
#1120=B_SPLINE_CURVE_WITH_KNOTS('',2,(#46615,#46616,#46617),
 .UNSPECIFIED.,.F.,.F.,(3,3),(0.,1.),.UNSPECIFIED.);
#1121=B_SPLINE_CURVE_WITH_KNOTS('',2,(#46620,#46621,#46622),
 .UNSPECIFIED.,.F.,.F.,(3,3),(0.,1.),.UNSPECIFIED.);
#1122=B_SPLINE_CURVE_WITH_KNOTS('',2,(#46629,#46630,#46631),
 .UNSPECIFIED.,.F.,.F.,(3,3),(0.,1.),.UNSPECIFIED.);
#1123=B_SPLINE_CURVE_WITH_KNOTS('',2,(#46632,#46633,#46634),
 .UNSPECIFIED.,.F.,.F.,(3,3),(0.,1.),.UNSPECIFIED.);
#1124=B_SPLINE_CURVE_WITH_KNOTS('',2,(#46644,#46645,#46646),
 .UNSPECIFIED.,.F.,.F.,(3,3),(0.,1.),.UNSPECIFIED.);
#1125=B_SPLINE_CURVE_WITH_KNOTS('',2,(#46650,#46651,#46652),
 .UNSPECIFIED.,.F.,.F.,(3,3),(0.,1.),.UNSPECIFIED.);
#1126=B_SPLINE_CURVE_WITH_KNOTS('',2,(#46661,#46662,#46663),
 .UNSPECIFIED.,.F.,.F.,(3,3),(0.,1.),.UNSPECIFIED.);
#1127=B_SPLINE_CURVE_WITH_KNOTS('',2,(#46666,#46667,#46668),
 .UNSPECIFIED.,.F.,.F.,(3,3),(0.,1.),.UNSPECIFIED.);
#1128=B_SPLINE_CURVE_WITH_KNOTS('',2,(#46676,#46677,#46678),
 .UNSPECIFIED.,.F.,.F.,(3,3),(0.,1.),.UNSPECIFIED.);
#1129=B_SPLINE_CURVE_WITH_KNOTS('',2,(#46681,#46682,#46683),
 .UNSPECIFIED.,.F.,.F.,(3,3),(0.,1.),.UNSPECIFIED.);
#1130=B_SPLINE_CURVE_WITH_KNOTS('',2,(#46691,#46692,#46693),
 .UNSPECIFIED.,.F.,.F.,(3,3),(0.,1.),.UNSPECIFIED.);
#1131=B_SPLINE_CURVE_WITH_KNOTS('',2,(#46696,#46697,#46698),
 .UNSPECIFIED.,.F.,.F.,(3,3),(0.,1.),.UNSPECIFIED.);
#1132=B_SPLINE_CURVE_WITH_KNOTS('',2,(#46706,#46707,#46708),
 .UNSPECIFIED.,.F.,.F.,(3,3),(0.,1.),.UNSPECIFIED.);
#1133=B_SPLINE_CURVE_WITH_KNOTS('',2,(#46711,#46712,#46713),
 .UNSPECIFIED.,.F.,.F.,(3,3),(0.,1.),.UNSPECIFIED.);
#1134=B_SPLINE_CURVE_WITH_KNOTS('',2,(#46721,#46722,#46723),
 .UNSPECIFIED.,.F.,.F.,(3,3),(0.,1.),.UNSPECIFIED.);
#1135=B_SPLINE_CURVE_WITH_KNOTS('',2,(#46726,#46727,#46728),
 .UNSPECIFIED.,.F.,.F.,(3,3),(0.,1.),.UNSPECIFIED.);
#1136=B_SPLINE_CURVE_WITH_KNOTS('',2,(#46736,#46737,#46738),
 .UNSPECIFIED.,.F.,.F.,(3,3),(0.,1.),.UNSPECIFIED.);
#1137=B_SPLINE_CURVE_WITH_KNOTS('',2,(#46741,#46742,#46743),
 .UNSPECIFIED.,.F.,.F.,(3,3),(0.,1.),.UNSPECIFIED.);
#1138=B_SPLINE_CURVE_WITH_KNOTS('',2,(#46750,#46751,#46752),
 .UNSPECIFIED.,.F.,.F.,(3,3),(0.,1.),.UNSPECIFIED.);
#1139=B_SPLINE_CURVE_WITH_KNOTS('',2,(#46753,#46754,#46755),
 .UNSPECIFIED.,.F.,.F.,(3,3),(0.,1.),.UNSPECIFIED.);
#1140=B_SPLINE_CURVE_WITH_KNOTS('',2,(#46764,#46765,#46766),
 .UNSPECIFIED.,.F.,.F.,(3,3),(0.,1.),.UNSPECIFIED.);
#1141=B_SPLINE_CURVE_WITH_KNOTS('',2,(#46770,#46771,#46772),
 .UNSPECIFIED.,.F.,.F.,(3,3),(0.,1.),.UNSPECIFIED.);
#1142=B_SPLINE_CURVE_WITH_KNOTS('',2,(#46781,#46782,#46783),
 .UNSPECIFIED.,.F.,.F.,(3,3),(0.,1.),.UNSPECIFIED.);
#1143=B_SPLINE_CURVE_WITH_KNOTS('',2,(#46786,#46787,#46788),
 .UNSPECIFIED.,.F.,.F.,(3,3),(0.,1.),.UNSPECIFIED.);
#1144=B_SPLINE_CURVE_WITH_KNOTS('',2,(#46796,#46797,#46798),
 .UNSPECIFIED.,.F.,.F.,(3,3),(0.,1.),.UNSPECIFIED.);
#1145=B_SPLINE_CURVE_WITH_KNOTS('',2,(#46801,#46802,#46803),
 .UNSPECIFIED.,.F.,.F.,(3,3),(0.,1.),.UNSPECIFIED.);
#1146=B_SPLINE_CURVE_WITH_KNOTS('',2,(#46811,#46812,#46813),
 .UNSPECIFIED.,.F.,.F.,(3,3),(0.,1.),.UNSPECIFIED.);
#1147=B_SPLINE_CURVE_WITH_KNOTS('',2,(#46816,#46817,#46818),
 .UNSPECIFIED.,.F.,.F.,(3,3),(0.,1.),.UNSPECIFIED.);
#1148=B_SPLINE_CURVE_WITH_KNOTS('',2,(#46826,#46827,#46828),
 .UNSPECIFIED.,.F.,.F.,(3,3),(0.,1.),.UNSPECIFIED.);
#1149=B_SPLINE_CURVE_WITH_KNOTS('',2,(#46831,#46832,#46833),
 .UNSPECIFIED.,.F.,.F.,(3,3),(0.,1.),.UNSPECIFIED.);
#1150=B_SPLINE_CURVE_WITH_KNOTS('',2,(#46841,#46842,#46843),
 .UNSPECIFIED.,.F.,.F.,(3,3),(0.,1.),.UNSPECIFIED.);
#1151=B_SPLINE_CURVE_WITH_KNOTS('',2,(#46846,#46847,#46848),
 .UNSPECIFIED.,.F.,.F.,(3,3),(0.,1.),.UNSPECIFIED.);
#1152=B_SPLINE_CURVE_WITH_KNOTS('',2,(#46856,#46857,#46858),
 .UNSPECIFIED.,.F.,.F.,(3,3),(0.,1.),.UNSPECIFIED.);
#1153=B_SPLINE_CURVE_WITH_KNOTS('',2,(#46861,#46862,#46863),
 .UNSPECIFIED.,.F.,.F.,(3,3),(0.,1.),.UNSPECIFIED.);
#1154=B_SPLINE_CURVE_WITH_KNOTS('',2,(#46900,#46901,#46902),
 .UNSPECIFIED.,.F.,.F.,(3,3),(0.,1.),.UNSPECIFIED.);
#1155=B_SPLINE_CURVE_WITH_KNOTS('',2,(#46903,#46904,#46905),
 .UNSPECIFIED.,.F.,.F.,(3,3),(0.,1.),.UNSPECIFIED.);
#1156=B_SPLINE_CURVE_WITH_KNOTS('',2,(#46915,#46916,#46917),
 .UNSPECIFIED.,.F.,.F.,(3,3),(0.,1.),.UNSPECIFIED.);
#1157=B_SPLINE_CURVE_WITH_KNOTS('',2,(#46921,#46922,#46923),
 .UNSPECIFIED.,.F.,.F.,(3,3),(0.,1.),.UNSPECIFIED.);
#1158=B_SPLINE_CURVE_WITH_KNOTS('',2,(#46932,#46933,#46934),
 .UNSPECIFIED.,.F.,.F.,(3,3),(0.,1.),.UNSPECIFIED.);
#1159=B_SPLINE_CURVE_WITH_KNOTS('',2,(#46937,#46938,#46939),
 .UNSPECIFIED.,.F.,.F.,(3,3),(0.,1.),.UNSPECIFIED.);
#1160=B_SPLINE_CURVE_WITH_KNOTS('',2,(#46947,#46948,#46949),
 .UNSPECIFIED.,.F.,.F.,(3,3),(0.,1.),.UNSPECIFIED.);
#1161=B_SPLINE_CURVE_WITH_KNOTS('',2,(#46952,#46953,#46954),
 .UNSPECIFIED.,.F.,.F.,(3,3),(0.,1.),.UNSPECIFIED.);
#1162=B_SPLINE_CURVE_WITH_KNOTS('',2,(#46962,#46963,#46964),
 .UNSPECIFIED.,.F.,.F.,(3,3),(0.,1.),.UNSPECIFIED.);
#1163=B_SPLINE_CURVE_WITH_KNOTS('',2,(#46967,#46968,#46969),
 .UNSPECIFIED.,.F.,.F.,(3,3),(0.,1.),.UNSPECIFIED.);
#1164=B_SPLINE_CURVE_WITH_KNOTS('',2,(#46983,#46984,#46985),
 .UNSPECIFIED.,.F.,.F.,(3,3),(0.,1.),.UNSPECIFIED.);
#1165=B_SPLINE_CURVE_WITH_KNOTS('',2,(#46988,#46989,#46990),
 .UNSPECIFIED.,.F.,.F.,(3,3),(0.,1.),.UNSPECIFIED.);
#1166=B_SPLINE_CURVE_WITH_KNOTS('',2,(#46998,#46999,#47000),
 .UNSPECIFIED.,.F.,.F.,(3,3),(0.,1.),.UNSPECIFIED.);
#1167=B_SPLINE_CURVE_WITH_KNOTS('',2,(#47003,#47004,#47005),
 .UNSPECIFIED.,.F.,.F.,(3,3),(0.,1.),.UNSPECIFIED.);
#1168=B_SPLINE_CURVE_WITH_KNOTS('',2,(#47013,#47014,#47015),
 .UNSPECIFIED.,.F.,.F.,(3,3),(0.,1.),.UNSPECIFIED.);
#1169=B_SPLINE_CURVE_WITH_KNOTS('',2,(#47018,#47019,#47020),
 .UNSPECIFIED.,.F.,.F.,(3,3),(0.,1.),.UNSPECIFIED.);
#1170=B_SPLINE_CURVE_WITH_KNOTS('',3,(#47061,#47062,#47063,#47064,#47065,
#47066,#47067,#47068,#47069,#47070),.UNSPECIFIED.,.F.,.F.,(4,2,2,2,4),(0.466330361623161,
0.582535633002934,0.698740904382707,0.815700813814515,0.932660723246322),
 .UNSPECIFIED.);
#1171=B_SPLINE_CURVE_WITH_KNOTS('',3,(#47072,#47073,#47074,#47075,#47076,
#47077,#47078,#47079,#47080,#47081),.UNSPECIFIED.,.F.,.F.,(4,2,2,2,4),(0.,
0.116959909431808,0.233919818863615,0.350125090243388,0.466330361623161),
 .UNSPECIFIED.);
#1172=B_SPLINE_CURVE_WITH_KNOTS('',3,(#47083,#47084,#47085,#47086,#47087,
#47088,#47089,#47090,#47091,#47092),.UNSPECIFIED.,.F.,.F.,(4,2,2,2,4),(1.39899108486948,
1.51519635624926,1.63140162762903,1.74836153706084,1.86532144649264),
 .UNSPECIFIED.);
#1173=B_SPLINE_CURVE_WITH_KNOTS('',3,(#47093,#47094,#47095,#47096,#47097,
#47098,#47099,#47100,#47101,#47102),.UNSPECIFIED.,.F.,.F.,(4,2,2,2,4),(0.932660723246322,
1.04962063267813,1.16658054210994,1.28278581348971,1.39899108486948),
 .UNSPECIFIED.);
#1174=B_SPLINE_CURVE_WITH_KNOTS('',3,(#47118,#47119,#47120,#47121,#47122,
#47123,#47124,#47125,#47126,#47127,#47128,#47129,#47130,#47131,#47132,#47133,
#47134,#47135,#47136,#47137,#47138,#47139,#47140,#47141,#47142,#47143),
 .UNSPECIFIED.,.F.,.F.,(4,2,2,2,2,2,2,2,2,2,2,2,4),(1.72309603002439,1.81125279412847,
1.94756976198853,2.21280480266174,2.5211516170085,2.82949843135526,3.44619206004878,
4.06288568874231,4.37123250308907,4.67957931743583,4.94481435810904,5.0811313259691,
5.16928809007318),.UNSPECIFIED.);
#1520=SHAPE_REPRESENTATION_RELATIONSHIP('SRR','None',#59309,#1540);
#1540=ADVANCED_BREP_SHAPE_REPRESENTATION('',(#1587),#59196);
#1566=STYLED_ITEM('',(#59586),#22320);
#1567=STYLED_ITEM('',(#59586),#1587);
#1587=MANIFOLD_SOLID_BREP('Rear cover',#22816);
#1716=FACE_BOUND('',#4623,.T.);
#1717=FACE_BOUND('',#4645,.T.);
#1718=FACE_BOUND('',#4722,.T.);
#1719=FACE_BOUND('',#4833,.T.);
#1720=FACE_BOUND('',#4863,.T.);
#1721=FACE_BOUND('',#4886,.T.);
#1722=FACE_BOUND('',#4911,.T.);
#1723=FACE_BOUND('',#4915,.T.);
#1724=FACE_BOUND('',#4921,.T.);
#1725=FACE_BOUND('',#4922,.T.);
#1726=FACE_BOUND('',#4923,.T.);
#1727=FACE_BOUND('',#4924,.T.);
#1728=FACE_BOUND('',#4925,.T.);
#1729=FACE_BOUND('',#4926,.T.);
#1730=FACE_BOUND('',#4927,.T.);
#1731=FACE_BOUND('',#4928,.T.);
#1732=FACE_BOUND('',#4949,.T.);
#1733=FACE_BOUND('',#4950,.T.);
#1734=FACE_BOUND('',#4951,.T.);
#1735=FACE_BOUND('',#4952,.T.);
#1736=FACE_BOUND('',#4953,.T.);
#1737=FACE_BOUND('',#4954,.T.);
#1738=FACE_BOUND('',#4955,.T.);
#1739=FACE_BOUND('',#4956,.T.);
#1740=FACE_BOUND('',#4957,.T.);
#1741=FACE_BOUND('',#4958,.T.);
#1742=FACE_BOUND('',#4959,.T.);
#1743=FACE_BOUND('',#4960,.T.);
#1744=FACE_BOUND('',#4961,.T.);
#1745=FACE_BOUND('',#4962,.T.);
#1746=FACE_BOUND('',#4967,.T.);
#2051=PLANE('',#23997);
#2052=PLANE('',#23998);
#2053=PLANE('',#23999);
#2054=PLANE('',#24000);
#2055=PLANE('',#24001);
#2056=PLANE('',#24002);
#2057=PLANE('',#24003);
#2058=PLANE('',#24004);
#2059=PLANE('',#24005);
#2060=PLANE('',#24006);
#2061=PLANE('',#24007);
#2062=PLANE('',#24008);
#2063=PLANE('',#24009);
#2064=PLANE('',#24010);
#2065=PLANE('',#24011);
#2066=PLANE('',#24012);
#2067=PLANE('',#24013);
#2068=PLANE('',#24014);
#2069=PLANE('',#24015);
#2070=PLANE('',#24016);
#2071=PLANE('',#24017);
#2072=PLANE('',#24018);
#2073=PLANE('',#24019);
#2074=PLANE('',#24020);
#2075=PLANE('',#24021);
#2076=PLANE('',#24022);
#2077=PLANE('',#24023);
#2078=PLANE('',#24024);
#2079=PLANE('',#24025);
#2080=PLANE('',#24026);
#2081=PLANE('',#24027);
#2082=PLANE('',#24028);
#2083=PLANE('',#24029);
#2084=PLANE('',#24030);
#2085=PLANE('',#24031);
#2086=PLANE('',#24032);
#2087=PLANE('',#24033);
#2088=PLANE('',#24034);
#2089=PLANE('',#24035);
#2090=PLANE('',#24036);
#2091=PLANE('',#24037);
#2092=PLANE('',#24038);
#2093=PLANE('',#24039);
#2094=PLANE('',#24040);
#2095=PLANE('',#24041);
#2096=PLANE('',#24042);
#2097=PLANE('',#24043);
#2098=PLANE('',#24044);
#2099=PLANE('',#24045);
#2100=PLANE('',#24046);
#2101=PLANE('',#24047);
#2102=PLANE('',#24048);
#2103=PLANE('',#24049);
#2104=PLANE('',#24050);
#2105=PLANE('',#24051);
#2106=PLANE('',#24052);
#2107=PLANE('',#24053);
#2108=PLANE('',#24054);
#2109=PLANE('',#24055);
#2110=PLANE('',#24056);
#2111=PLANE('',#24057);
#2112=PLANE('',#24058);
#2113=PLANE('',#24059);
#2114=PLANE('',#24060);
#2115=PLANE('',#24061);
#2116=PLANE('',#24062);
#2117=PLANE('',#24063);
#2118=PLANE('',#24064);
#2119=PLANE('',#24065);
#2120=PLANE('',#24066);
#2121=PLANE('',#24067);
#2122=PLANE('',#24068);
#2123=PLANE('',#24069);
#2124=PLANE('',#24070);
#2125=PLANE('',#24071);
#2126=PLANE('',#24072);
#2127=PLANE('',#24073);
#2128=PLANE('',#24074);
#2129=PLANE('',#24075);
#2130=PLANE('',#24076);
#2131=PLANE('',#24077);
#2132=PLANE('',#24078);
#2133=PLANE('',#24079);
#2134=PLANE('',#24080);
#2135=PLANE('',#24081);
#2136=PLANE('',#24082);
#2137=PLANE('',#24083);
#2138=PLANE('',#24084);
#2139=PLANE('',#24085);
#2140=PLANE('',#24093);
#2141=PLANE('',#24098);
#2142=PLANE('',#24099);
#2143=PLANE('',#24111);
#2144=PLANE('',#24152);
#2145=PLANE('',#24154);
#2146=PLANE('',#24158);
#2553=CYLINDRICAL_SURFACE('',#24086,0.3);
#2554=CYLINDRICAL_SURFACE('',#24091,0.8381);
#2555=CYLINDRICAL_SURFACE('',#24096,0.5);
#2556=CYLINDRICAL_SURFACE('',#24101,7.);
#2557=CYLINDRICAL_SURFACE('',#24119,0.404999999999999);
#2558=CYLINDRICAL_SURFACE('',#24123,0.404999999999999);
#2559=CYLINDRICAL_SURFACE('',#24127,0.405);
#2560=CYLINDRICAL_SURFACE('',#24131,0.404999999999999);
#2561=CYLINDRICAL_SURFACE('',#24135,0.405);
#2562=CYLINDRICAL_SURFACE('',#24139,0.404999999999999);
#2563=CYLINDRICAL_SURFACE('',#24150,2.6);
#2564=CYLINDRICAL_SURFACE('',#24156,2.4);
#3163=FACE_OUTER_BOUND('',#4585,.T.);
#3164=FACE_OUTER_BOUND('',#4586,.T.);
#3165=FACE_OUTER_BOUND('',#4587,.T.);
#3166=FACE_OUTER_BOUND('',#4588,.T.);
#3167=FACE_OUTER_BOUND('',#4589,.T.);
#3168=FACE_OUTER_BOUND('',#4590,.T.);
#3169=FACE_OUTER_BOUND('',#4591,.T.);
#3170=FACE_OUTER_BOUND('',#4592,.T.);
#3171=FACE_OUTER_BOUND('',#4593,.T.);
#3172=FACE_OUTER_BOUND('',#4594,.T.);
#3173=FACE_OUTER_BOUND('',#4595,.T.);
#3174=FACE_OUTER_BOUND('',#4596,.T.);
#3175=FACE_OUTER_BOUND('',#4597,.T.);
#3176=FACE_OUTER_BOUND('',#4598,.T.);
#3177=FACE_OUTER_BOUND('',#4599,.T.);
#3178=FACE_OUTER_BOUND('',#4600,.T.);
#3179=FACE_OUTER_BOUND('',#4601,.T.);
#3180=FACE_OUTER_BOUND('',#4602,.T.);
#3181=FACE_OUTER_BOUND('',#4603,.T.);
#3182=FACE_OUTER_BOUND('',#4604,.T.);
#3183=FACE_OUTER_BOUND('',#4605,.T.);
#3184=FACE_OUTER_BOUND('',#4606,.T.);
#3185=FACE_OUTER_BOUND('',#4607,.T.);
#3186=FACE_OUTER_BOUND('',#4608,.T.);
#3187=FACE_OUTER_BOUND('',#4609,.T.);
#3188=FACE_OUTER_BOUND('',#4610,.T.);
#3189=FACE_OUTER_BOUND('',#4611,.T.);
#3190=FACE_OUTER_BOUND('',#4612,.T.);
#3191=FACE_OUTER_BOUND('',#4613,.T.);
#3192=FACE_OUTER_BOUND('',#4614,.T.);
#3193=FACE_OUTER_BOUND('',#4615,.T.);
#3194=FACE_OUTER_BOUND('',#4616,.T.);
#3195=FACE_OUTER_BOUND('',#4617,.T.);
#3196=FACE_OUTER_BOUND('',#4618,.T.);
#3197=FACE_OUTER_BOUND('',#4619,.T.);
#3198=FACE_OUTER_BOUND('',#4620,.T.);
#3199=FACE_OUTER_BOUND('',#4621,.T.);
#3200=FACE_OUTER_BOUND('',#4622,.T.);
#3201=FACE_OUTER_BOUND('',#4624,.T.);
#3202=FACE_OUTER_BOUND('',#4625,.T.);
#3203=FACE_OUTER_BOUND('',#4626,.T.);
#3204=FACE_OUTER_BOUND('',#4627,.T.);
#3205=FACE_OUTER_BOUND('',#4628,.T.);
#3206=FACE_OUTER_BOUND('',#4629,.T.);
#3207=FACE_OUTER_BOUND('',#4630,.T.);
#3208=FACE_OUTER_BOUND('',#4631,.T.);
#3209=FACE_OUTER_BOUND('',#4632,.T.);
#3210=FACE_OUTER_BOUND('',#4633,.T.);
#3211=FACE_OUTER_BOUND('',#4634,.T.);
#3212=FACE_OUTER_BOUND('',#4635,.T.);
#3213=FACE_OUTER_BOUND('',#4636,.T.);
#3214=FACE_OUTER_BOUND('',#4637,.T.);
#3215=FACE_OUTER_BOUND('',#4638,.T.);
#3216=FACE_OUTER_BOUND('',#4639,.T.);
#3217=FACE_OUTER_BOUND('',#4640,.T.);
#3218=FACE_OUTER_BOUND('',#4641,.T.);
#3219=FACE_OUTER_BOUND('',#4642,.T.);
#3220=FACE_OUTER_BOUND('',#4643,.T.);
#3221=FACE_OUTER_BOUND('',#4644,.T.);
#3222=FACE_OUTER_BOUND('',#4646,.T.);
#3223=FACE_OUTER_BOUND('',#4647,.T.);
#3224=FACE_OUTER_BOUND('',#4648,.T.);
#3225=FACE_OUTER_BOUND('',#4649,.T.);
#3226=FACE_OUTER_BOUND('',#4650,.T.);
#3227=FACE_OUTER_BOUND('',#4651,.T.);
#3228=FACE_OUTER_BOUND('',#4652,.T.);
#3229=FACE_OUTER_BOUND('',#4653,.T.);
#3230=FACE_OUTER_BOUND('',#4654,.T.);
#3231=FACE_OUTER_BOUND('',#4655,.T.);
#3232=FACE_OUTER_BOUND('',#4656,.T.);
#3233=FACE_OUTER_BOUND('',#4657,.T.);
#3234=FACE_OUTER_BOUND('',#4658,.T.);
#3235=FACE_OUTER_BOUND('',#4659,.T.);
#3236=FACE_OUTER_BOUND('',#4660,.T.);
#3237=FACE_OUTER_BOUND('',#4661,.T.);
#3238=FACE_OUTER_BOUND('',#4662,.T.);
#3239=FACE_OUTER_BOUND('',#4663,.T.);
#3240=FACE_OUTER_BOUND('',#4664,.T.);
#3241=FACE_OUTER_BOUND('',#4665,.T.);
#3242=FACE_OUTER_BOUND('',#4666,.T.);
#3243=FACE_OUTER_BOUND('',#4667,.T.);
#3244=FACE_OUTER_BOUND('',#4668,.T.);
#3245=FACE_OUTER_BOUND('',#4669,.T.);
#3246=FACE_OUTER_BOUND('',#4670,.T.);
#3247=FACE_OUTER_BOUND('',#4671,.T.);
#3248=FACE_OUTER_BOUND('',#4672,.T.);
#3249=FACE_OUTER_BOUND('',#4673,.T.);
#3250=FACE_OUTER_BOUND('',#4674,.T.);
#3251=FACE_OUTER_BOUND('',#4675,.T.);
#3252=FACE_OUTER_BOUND('',#4676,.T.);
#3253=FACE_OUTER_BOUND('',#4677,.T.);
#3254=FACE_OUTER_BOUND('',#4678,.T.);
#3255=FACE_OUTER_BOUND('',#4679,.T.);
#3256=FACE_OUTER_BOUND('',#4680,.T.);
#3257=FACE_OUTER_BOUND('',#4681,.T.);
#3258=FACE_OUTER_BOUND('',#4682,.T.);
#3259=FACE_OUTER_BOUND('',#4683,.T.);
#3260=FACE_OUTER_BOUND('',#4684,.T.);
#3261=FACE_OUTER_BOUND('',#4685,.T.);
#3262=FACE_OUTER_BOUND('',#4686,.T.);
#3263=FACE_OUTER_BOUND('',#4687,.T.);
#3264=FACE_OUTER_BOUND('',#4688,.T.);
#3265=FACE_OUTER_BOUND('',#4689,.T.);
#3266=FACE_OUTER_BOUND('',#4690,.T.);
#3267=FACE_OUTER_BOUND('',#4691,.T.);
#3268=FACE_OUTER_BOUND('',#4692,.T.);
#3269=FACE_OUTER_BOUND('',#4693,.T.);
#3270=FACE_OUTER_BOUND('',#4694,.T.);
#3271=FACE_OUTER_BOUND('',#4695,.T.);
#3272=FACE_OUTER_BOUND('',#4696,.T.);
#3273=FACE_OUTER_BOUND('',#4697,.T.);
#3274=FACE_OUTER_BOUND('',#4698,.T.);
#3275=FACE_OUTER_BOUND('',#4699,.T.);
#3276=FACE_OUTER_BOUND('',#4700,.T.);
#3277=FACE_OUTER_BOUND('',#4701,.T.);
#3278=FACE_OUTER_BOUND('',#4702,.T.);
#3279=FACE_OUTER_BOUND('',#4703,.T.);
#3280=FACE_OUTER_BOUND('',#4704,.T.);
#3281=FACE_OUTER_BOUND('',#4705,.T.);
#3282=FACE_OUTER_BOUND('',#4706,.T.);
#3283=FACE_OUTER_BOUND('',#4707,.T.);
#3284=FACE_OUTER_BOUND('',#4708,.T.);
#3285=FACE_OUTER_BOUND('',#4709,.T.);
#3286=FACE_OUTER_BOUND('',#4710,.T.);
#3287=FACE_OUTER_BOUND('',#4711,.T.);
#3288=FACE_OUTER_BOUND('',#4712,.T.);
#3289=FACE_OUTER_BOUND('',#4713,.T.);
#3290=FACE_OUTER_BOUND('',#4714,.T.);
#3291=FACE_OUTER_BOUND('',#4715,.T.);
#3292=FACE_OUTER_BOUND('',#4716,.T.);
#3293=FACE_OUTER_BOUND('',#4717,.T.);
#3294=FACE_OUTER_BOUND('',#4718,.T.);
#3295=FACE_OUTER_BOUND('',#4719,.T.);
#3296=FACE_OUTER_BOUND('',#4720,.T.);
#3297=FACE_OUTER_BOUND('',#4721,.T.);
#3298=FACE_OUTER_BOUND('',#4723,.T.);
#3299=FACE_OUTER_BOUND('',#4724,.T.);
#3300=FACE_OUTER_BOUND('',#4725,.T.);
#3301=FACE_OUTER_BOUND('',#4726,.T.);
#3302=FACE_OUTER_BOUND('',#4727,.T.);
#3303=FACE_OUTER_BOUND('',#4728,.T.);
#3304=FACE_OUTER_BOUND('',#4729,.T.);
#3305=FACE_OUTER_BOUND('',#4730,.T.);
#3306=FACE_OUTER_BOUND('',#4731,.T.);
#3307=FACE_OUTER_BOUND('',#4732,.T.);
#3308=FACE_OUTER_BOUND('',#4733,.T.);
#3309=FACE_OUTER_BOUND('',#4734,.T.);
#3310=FACE_OUTER_BOUND('',#4735,.T.);
#3311=FACE_OUTER_BOUND('',#4736,.T.);
#3312=FACE_OUTER_BOUND('',#4737,.T.);
#3313=FACE_OUTER_BOUND('',#4738,.T.);
#3314=FACE_OUTER_BOUND('',#4739,.T.);
#3315=FACE_OUTER_BOUND('',#4740,.T.);
#3316=FACE_OUTER_BOUND('',#4741,.T.);
#3317=FACE_OUTER_BOUND('',#4742,.T.);
#3318=FACE_OUTER_BOUND('',#4743,.T.);
#3319=FACE_OUTER_BOUND('',#4744,.T.);
#3320=FACE_OUTER_BOUND('',#4745,.T.);
#3321=FACE_OUTER_BOUND('',#4746,.T.);
#3322=FACE_OUTER_BOUND('',#4747,.T.);
#3323=FACE_OUTER_BOUND('',#4748,.T.);
#3324=FACE_OUTER_BOUND('',#4749,.T.);
#3325=FACE_OUTER_BOUND('',#4750,.T.);
#3326=FACE_OUTER_BOUND('',#4751,.T.);
#3327=FACE_OUTER_BOUND('',#4752,.T.);
#3328=FACE_OUTER_BOUND('',#4753,.T.);
#3329=FACE_OUTER_BOUND('',#4754,.T.);
#3330=FACE_OUTER_BOUND('',#4755,.T.);
#3331=FACE_OUTER_BOUND('',#4756,.T.);
#3332=FACE_OUTER_BOUND('',#4757,.T.);
#3333=FACE_OUTER_BOUND('',#4758,.T.);
#3334=FACE_OUTER_BOUND('',#4759,.T.);
#3335=FACE_OUTER_BOUND('',#4760,.T.);
#3336=FACE_OUTER_BOUND('',#4761,.T.);
#3337=FACE_OUTER_BOUND('',#4762,.T.);
#3338=FACE_OUTER_BOUND('',#4763,.T.);
#3339=FACE_OUTER_BOUND('',#4764,.T.);
#3340=FACE_OUTER_BOUND('',#4765,.T.);
#3341=FACE_OUTER_BOUND('',#4766,.T.);
#3342=FACE_OUTER_BOUND('',#4767,.T.);
#3343=FACE_OUTER_BOUND('',#4768,.T.);
#3344=FACE_OUTER_BOUND('',#4769,.T.);
#3345=FACE_OUTER_BOUND('',#4770,.T.);
#3346=FACE_OUTER_BOUND('',#4771,.T.);
#3347=FACE_OUTER_BOUND('',#4772,.T.);
#3348=FACE_OUTER_BOUND('',#4773,.T.);
#3349=FACE_OUTER_BOUND('',#4774,.T.);
#3350=FACE_OUTER_BOUND('',#4775,.T.);
#3351=FACE_OUTER_BOUND('',#4776,.T.);
#3352=FACE_OUTER_BOUND('',#4777,.T.);
#3353=FACE_OUTER_BOUND('',#4778,.T.);
#3354=FACE_OUTER_BOUND('',#4779,.T.);
#3355=FACE_OUTER_BOUND('',#4780,.T.);
#3356=FACE_OUTER_BOUND('',#4781,.T.);
#3357=FACE_OUTER_BOUND('',#4782,.T.);
#3358=FACE_OUTER_BOUND('',#4783,.T.);
#3359=FACE_OUTER_BOUND('',#4784,.T.);
#3360=FACE_OUTER_BOUND('',#4785,.T.);
#3361=FACE_OUTER_BOUND('',#4786,.T.);
#3362=FACE_OUTER_BOUND('',#4787,.T.);
#3363=FACE_OUTER_BOUND('',#4788,.T.);
#3364=FACE_OUTER_BOUND('',#4789,.T.);
#3365=FACE_OUTER_BOUND('',#4790,.T.);
#3366=FACE_OUTER_BOUND('',#4791,.T.);
#3367=FACE_OUTER_BOUND('',#4792,.T.);
#3368=FACE_OUTER_BOUND('',#4793,.T.);
#3369=FACE_OUTER_BOUND('',#4794,.T.);
#3370=FACE_OUTER_BOUND('',#4795,.T.);
#3371=FACE_OUTER_BOUND('',#4796,.T.);
#3372=FACE_OUTER_BOUND('',#4797,.T.);
#3373=FACE_OUTER_BOUND('',#4798,.T.);
#3374=FACE_OUTER_BOUND('',#4799,.T.);
#3375=FACE_OUTER_BOUND('',#4800,.T.);
#3376=FACE_OUTER_BOUND('',#4801,.T.);
#3377=FACE_OUTER_BOUND('',#4802,.T.);
#3378=FACE_OUTER_BOUND('',#4803,.T.);
#3379=FACE_OUTER_BOUND('',#4804,.T.);
#3380=FACE_OUTER_BOUND('',#4805,.T.);
#3381=FACE_OUTER_BOUND('',#4806,.T.);
#3382=FACE_OUTER_BOUND('',#4807,.T.);
#3383=FACE_OUTER_BOUND('',#4808,.T.);
#3384=FACE_OUTER_BOUND('',#4809,.T.);
#3385=FACE_OUTER_BOUND('',#4810,.T.);
#3386=FACE_OUTER_BOUND('',#4811,.T.);
#3387=FACE_OUTER_BOUND('',#4812,.T.);
#3388=FACE_OUTER_BOUND('',#4813,.T.);
#3389=FACE_OUTER_BOUND('',#4814,.T.);
#3390=FACE_OUTER_BOUND('',#4815,.T.);
#3391=FACE_OUTER_BOUND('',#4816,.T.);
#3392=FACE_OUTER_BOUND('',#4817,.T.);
#3393=FACE_OUTER_BOUND('',#4818,.T.);
#3394=FACE_OUTER_BOUND('',#4819,.T.);
#3395=FACE_OUTER_BOUND('',#4820,.T.);
#3396=FACE_OUTER_BOUND('',#4821,.T.);
#3397=FACE_OUTER_BOUND('',#4822,.T.);
#3398=FACE_OUTER_BOUND('',#4823,.T.);
#3399=FACE_OUTER_BOUND('',#4824,.T.);
#3400=FACE_OUTER_BOUND('',#4825,.T.);
#3401=FACE_OUTER_BOUND('',#4826,.T.);
#3402=FACE_OUTER_BOUND('',#4827,.T.);
#3403=FACE_OUTER_BOUND('',#4828,.T.);
#3404=FACE_OUTER_BOUND('',#4829,.T.);
#3405=FACE_OUTER_BOUND('',#4830,.T.);
#3406=FACE_OUTER_BOUND('',#4831,.T.);
#3407=FACE_OUTER_BOUND('',#4832,.T.);
#3408=FACE_OUTER_BOUND('',#4834,.T.);
#3409=FACE_OUTER_BOUND('',#4835,.T.);
#3410=FACE_OUTER_BOUND('',#4836,.T.);
#3411=FACE_OUTER_BOUND('',#4837,.T.);
#3412=FACE_OUTER_BOUND('',#4838,.T.);
#3413=FACE_OUTER_BOUND('',#4839,.T.);
#3414=FACE_OUTER_BOUND('',#4840,.T.);
#3415=FACE_OUTER_BOUND('',#4841,.T.);
#3416=FACE_OUTER_BOUND('',#4842,.T.);
#3417=FACE_OUTER_BOUND('',#4843,.T.);
#3418=FACE_OUTER_BOUND('',#4844,.T.);
#3419=FACE_OUTER_BOUND('',#4845,.T.);
#3420=FACE_OUTER_BOUND('',#4846,.T.);
#3421=FACE_OUTER_BOUND('',#4847,.T.);
#3422=FACE_OUTER_BOUND('',#4848,.T.);
#3423=FACE_OUTER_BOUND('',#4849,.T.);
#3424=FACE_OUTER_BOUND('',#4850,.T.);
#3425=FACE_OUTER_BOUND('',#4851,.T.);
#3426=FACE_OUTER_BOUND('',#4852,.T.);
#3427=FACE_OUTER_BOUND('',#4853,.T.);
#3428=FACE_OUTER_BOUND('',#4854,.T.);
#3429=FACE_OUTER_BOUND('',#4855,.T.);
#3430=FACE_OUTER_BOUND('',#4856,.T.);
#3431=FACE_OUTER_BOUND('',#4857,.T.);
#3432=FACE_OUTER_BOUND('',#4858,.T.);
#3433=FACE_OUTER_BOUND('',#4859,.T.);
#3434=FACE_OUTER_BOUND('',#4860,.T.);
#3435=FACE_OUTER_BOUND('',#4861,.T.);
#3436=FACE_OUTER_BOUND('',#4862,.T.);
#3437=FACE_OUTER_BOUND('',#4864,.T.);
#3438=FACE_OUTER_BOUND('',#4865,.T.);
#3439=FACE_OUTER_BOUND('',#4866,.T.);
#3440=FACE_OUTER_BOUND('',#4867,.T.);
#3441=FACE_OUTER_BOUND('',#4868,.T.);
#3442=FACE_OUTER_BOUND('',#4869,.T.);
#3443=FACE_OUTER_BOUND('',#4870,.T.);
#3444=FACE_OUTER_BOUND('',#4871,.T.);
#3445=FACE_OUTER_BOUND('',#4872,.T.);
#3446=FACE_OUTER_BOUND('',#4873,.T.);
#3447=FACE_OUTER_BOUND('',#4874,.T.);
#3448=FACE_OUTER_BOUND('',#4875,.T.);
#3449=FACE_OUTER_BOUND('',#4876,.T.);
#3450=FACE_OUTER_BOUND('',#4877,.T.);
#3451=FACE_OUTER_BOUND('',#4878,.T.);
#3452=FACE_OUTER_BOUND('',#4879,.T.);
#3453=FACE_OUTER_BOUND('',#4880,.T.);
#3454=FACE_OUTER_BOUND('',#4881,.T.);
#3455=FACE_OUTER_BOUND('',#4882,.T.);
#3456=FACE_OUTER_BOUND('',#4883,.T.);
#3457=FACE_OUTER_BOUND('',#4884,.T.);
#3458=FACE_OUTER_BOUND('',#4885,.T.);
#3459=FACE_OUTER_BOUND('',#4887,.T.);
#3460=FACE_OUTER_BOUND('',#4888,.T.);
#3461=FACE_OUTER_BOUND('',#4889,.T.);
#3462=FACE_OUTER_BOUND('',#4890,.T.);
#3463=FACE_OUTER_BOUND('',#4891,.T.);
#3464=FACE_OUTER_BOUND('',#4892,.T.);
#3465=FACE_OUTER_BOUND('',#4893,.T.);
#3466=FACE_OUTER_BOUND('',#4894,.T.);
#3467=FACE_OUTER_BOUND('',#4895,.T.);
#3468=FACE_OUTER_BOUND('',#4896,.T.);
#3469=FACE_OUTER_BOUND('',#4897,.T.);
#3470=FACE_OUTER_BOUND('',#4898,.T.);
#3471=FACE_OUTER_BOUND('',#4899,.T.);
#3472=FACE_OUTER_BOUND('',#4900,.T.);
#3473=FACE_OUTER_BOUND('',#4901,.T.);
#3474=FACE_OUTER_BOUND('',#4902,.T.);
#3475=FACE_OUTER_BOUND('',#4903,.T.);
#3476=FACE_OUTER_BOUND('',#4904,.T.);
#3477=FACE_OUTER_BOUND('',#4905,.T.);
#3478=FACE_OUTER_BOUND('',#4906,.T.);
#3479=FACE_OUTER_BOUND('',#4907,.T.);
#3480=FACE_OUTER_BOUND('',#4908,.T.);
#3481=FACE_OUTER_BOUND('',#4909,.T.);
#3482=FACE_OUTER_BOUND('',#4910,.T.);
#3483=FACE_OUTER_BOUND('',#4912,.T.);
#3484=FACE_OUTER_BOUND('',#4913,.T.);
#3485=FACE_OUTER_BOUND('',#4914,.T.);
#3486=FACE_OUTER_BOUND('',#4916,.T.);
#3487=FACE_OUTER_BOUND('',#4917,.T.);
#3488=FACE_OUTER_BOUND('',#4918,.T.);
#3489=FACE_OUTER_BOUND('',#4919,.T.);
#3490=FACE_OUTER_BOUND('',#4920,.T.);
#3491=FACE_OUTER_BOUND('',#4929,.T.);
#3492=FACE_OUTER_BOUND('',#4930,.T.);
#3493=FACE_OUTER_BOUND('',#4931,.T.);
#3494=FACE_OUTER_BOUND('',#4932,.T.);
#3495=FACE_OUTER_BOUND('',#4933,.T.);
#3496=FACE_OUTER_BOUND('',#4934,.T.);
#3497=FACE_OUTER_BOUND('',#4935,.T.);
#3498=FACE_OUTER_BOUND('',#4936,.T.);
#3499=FACE_OUTER_BOUND('',#4937,.T.);
#3500=FACE_OUTER_BOUND('',#4938,.T.);
#3501=FACE_OUTER_BOUND('',#4939,.T.);
#3502=FACE_OUTER_BOUND('',#4940,.T.);
#3503=FACE_OUTER_BOUND('',#4941,.T.);
#3504=FACE_OUTER_BOUND('',#4942,.T.);
#3505=FACE_OUTER_BOUND('',#4943,.T.);
#3506=FACE_OUTER_BOUND('',#4944,.T.);
#3507=FACE_OUTER_BOUND('',#4945,.T.);
#3508=FACE_OUTER_BOUND('',#4946,.T.);
#3509=FACE_OUTER_BOUND('',#4947,.T.);
#3510=FACE_OUTER_BOUND('',#4948,.T.);
#3511=FACE_OUTER_BOUND('',#4963,.T.);
#3512=FACE_OUTER_BOUND('',#4964,.T.);
#3513=FACE_OUTER_BOUND('',#4965,.T.);
#3514=FACE_OUTER_BOUND('',#4966,.T.);
#4585=EDGE_LOOP('',(#17030,#17031,#17032,#17033));
#4586=EDGE_LOOP('',(#17034,#17035,#17036,#17037));
#4587=EDGE_LOOP('',(#17038,#17039,#17040,#17041));
#4588=EDGE_LOOP('',(#17042,#17043,#17044,#17045));
#4589=EDGE_LOOP('',(#17046,#17047,#17048,#17049));
#4590=EDGE_LOOP('',(#17050,#17051,#17052,#17053));
#4591=EDGE_LOOP('',(#17054,#17055,#17056,#17057));
#4592=EDGE_LOOP('',(#17058,#17059,#17060,#17061));
#4593=EDGE_LOOP('',(#17062,#17063,#17064,#17065));
#4594=EDGE_LOOP('',(#17066,#17067,#17068,#17069));
#4595=EDGE_LOOP('',(#17070,#17071,#17072,#17073));
#4596=EDGE_LOOP('',(#17074,#17075,#17076,#17077));
#4597=EDGE_LOOP('',(#17078,#17079,#17080,#17081));
#4598=EDGE_LOOP('',(#17082,#17083,#17084,#17085));
#4599=EDGE_LOOP('',(#17086,#17087,#17088,#17089));
#4600=EDGE_LOOP('',(#17090,#17091,#17092,#17093));
#4601=EDGE_LOOP('',(#17094,#17095,#17096,#17097));
#4602=EDGE_LOOP('',(#17098,#17099,#17100,#17101));
#4603=EDGE_LOOP('',(#17102,#17103,#17104,#17105));
#4604=EDGE_LOOP('',(#17106,#17107,#17108,#17109));
#4605=EDGE_LOOP('',(#17110,#17111,#17112,#17113));
#4606=EDGE_LOOP('',(#17114,#17115,#17116,#17117));
#4607=EDGE_LOOP('',(#17118,#17119,#17120,#17121));
#4608=EDGE_LOOP('',(#17122,#17123,#17124,#17125));
#4609=EDGE_LOOP('',(#17126,#17127,#17128,#17129));
#4610=EDGE_LOOP('',(#17130,#17131,#17132,#17133));
#4611=EDGE_LOOP('',(#17134,#17135,#17136,#17137));
#4612=EDGE_LOOP('',(#17138,#17139,#17140,#17141));
#4613=EDGE_LOOP('',(#17142,#17143,#17144,#17145));
#4614=EDGE_LOOP('',(#17146,#17147,#17148,#17149));
#4615=EDGE_LOOP('',(#17150,#17151,#17152,#17153));
#4616=EDGE_LOOP('',(#17154,#17155,#17156,#17157));
#4617=EDGE_LOOP('',(#17158,#17159,#17160,#17161));
#4618=EDGE_LOOP('',(#17162,#17163,#17164,#17165));
#4619=EDGE_LOOP('',(#17166,#17167,#17168,#17169));
#4620=EDGE_LOOP('',(#17170,#17171,#17172,#17173));
#4621=EDGE_LOOP('',(#17174,#17175,#17176,#17177));
#4622=EDGE_LOOP('',(#17178,#17179,#17180,#17181,#17182,#17183,#17184,#17185,
#17186,#17187,#17188,#17189,#17190,#17191,#17192,#17193,#17194,#17195,#17196,
#17197,#17198,#17199,#17200,#17201,#17202,#17203,#17204));
#4623=EDGE_LOOP('',(#17205,#17206,#17207,#17208,#17209,#17210,#17211,#17212,
#17213,#17214));
#4624=EDGE_LOOP('',(#17215,#17216,#17217,#17218));
#4625=EDGE_LOOP('',(#17219,#17220,#17221,#17222));
#4626=EDGE_LOOP('',(#17223,#17224,#17225,#17226));
#4627=EDGE_LOOP('',(#17227,#17228,#17229,#17230));
#4628=EDGE_LOOP('',(#17231,#17232,#17233,#17234));
#4629=EDGE_LOOP('',(#17235,#17236,#17237,#17238));
#4630=EDGE_LOOP('',(#17239,#17240,#17241,#17242));
#4631=EDGE_LOOP('',(#17243,#17244,#17245,#17246));
#4632=EDGE_LOOP('',(#17247,#17248,#17249,#17250));
#4633=EDGE_LOOP('',(#17251,#17252,#17253,#17254));
#4634=EDGE_LOOP('',(#17255,#17256,#17257,#17258));
#4635=EDGE_LOOP('',(#17259,#17260,#17261,#17262));
#4636=EDGE_LOOP('',(#17263,#17264,#17265,#17266));
#4637=EDGE_LOOP('',(#17267,#17268,#17269,#17270));
#4638=EDGE_LOOP('',(#17271,#17272,#17273,#17274));
#4639=EDGE_LOOP('',(#17275,#17276,#17277,#17278));
#4640=EDGE_LOOP('',(#17279,#17280,#17281,#17282));
#4641=EDGE_LOOP('',(#17283,#17284,#17285,#17286));
#4642=EDGE_LOOP('',(#17287,#17288,#17289,#17290));
#4643=EDGE_LOOP('',(#17291,#17292,#17293,#17294));
#4644=EDGE_LOOP('',(#17295,#17296,#17297,#17298,#17299,#17300,#17301,#17302,
#17303,#17304,#17305,#17306));
#4645=EDGE_LOOP('',(#17307,#17308,#17309,#17310,#17311,#17312,#17313,#17314));
#4646=EDGE_LOOP('',(#17315,#17316,#17317,#17318));
#4647=EDGE_LOOP('',(#17319,#17320,#17321,#17322));
#4648=EDGE_LOOP('',(#17323,#17324,#17325,#17326));
#4649=EDGE_LOOP('',(#17327,#17328,#17329,#17330));
#4650=EDGE_LOOP('',(#17331,#17332,#17333,#17334));
#4651=EDGE_LOOP('',(#17335,#17336,#17337,#17338));
#4652=EDGE_LOOP('',(#17339,#17340,#17341,#17342));
#4653=EDGE_LOOP('',(#17343,#17344,#17345,#17346));
#4654=EDGE_LOOP('',(#17347,#17348,#17349,#17350));
#4655=EDGE_LOOP('',(#17351,#17352,#17353,#17354,#17355,#17356,#17357,#17358,
#17359));
#4656=EDGE_LOOP('',(#17360,#17361,#17362,#17363));
#4657=EDGE_LOOP('',(#17364,#17365,#17366,#17367));
#4658=EDGE_LOOP('',(#17368,#17369,#17370,#17371));
#4659=EDGE_LOOP('',(#17372,#17373,#17374,#17375));
#4660=EDGE_LOOP('',(#17376,#17377,#17378,#17379));
#4661=EDGE_LOOP('',(#17380,#17381,#17382,#17383));
#4662=EDGE_LOOP('',(#17384,#17385,#17386,#17387));
#4663=EDGE_LOOP('',(#17388,#17389,#17390,#17391));
#4664=EDGE_LOOP('',(#17392,#17393,#17394,#17395));
#4665=EDGE_LOOP('',(#17396,#17397,#17398,#17399));
#4666=EDGE_LOOP('',(#17400,#17401,#17402,#17403));
#4667=EDGE_LOOP('',(#17404,#17405,#17406,#17407));
#4668=EDGE_LOOP('',(#17408,#17409,#17410,#17411));
#4669=EDGE_LOOP('',(#17412,#17413,#17414,#17415));
#4670=EDGE_LOOP('',(#17416,#17417,#17418,#17419));
#4671=EDGE_LOOP('',(#17420,#17421,#17422,#17423,#17424,#17425,#17426,#17427,
#17428,#17429,#17430,#17431,#17432,#17433,#17434));
#4672=EDGE_LOOP('',(#17435,#17436,#17437,#17438));
#4673=EDGE_LOOP('',(#17439,#17440,#17441,#17442));
#4674=EDGE_LOOP('',(#17443,#17444,#17445,#17446));
#4675=EDGE_LOOP('',(#17447,#17448,#17449,#17450));
#4676=EDGE_LOOP('',(#17451,#17452,#17453,#17454));
#4677=EDGE_LOOP('',(#17455,#17456,#17457,#17458));
#4678=EDGE_LOOP('',(#17459,#17460,#17461,#17462));
#4679=EDGE_LOOP('',(#17463,#17464,#17465,#17466));
#4680=EDGE_LOOP('',(#17467,#17468,#17469,#17470));
#4681=EDGE_LOOP('',(#17471,#17472,#17473,#17474));
#4682=EDGE_LOOP('',(#17475,#17476,#17477,#17478));
#4683=EDGE_LOOP('',(#17479,#17480,#17481,#17482));
#4684=EDGE_LOOP('',(#17483,#17484,#17485,#17486));
#4685=EDGE_LOOP('',(#17487,#17488,#17489,#17490));
#4686=EDGE_LOOP('',(#17491,#17492,#17493,#17494));
#4687=EDGE_LOOP('',(#17495,#17496,#17497,#17498));
#4688=EDGE_LOOP('',(#17499,#17500,#17501,#17502));
#4689=EDGE_LOOP('',(#17503,#17504,#17505,#17506));
#4690=EDGE_LOOP('',(#17507,#17508,#17509,#17510));
#4691=EDGE_LOOP('',(#17511,#17512,#17513,#17514));
#4692=EDGE_LOOP('',(#17515,#17516,#17517,#17518));
#4693=EDGE_LOOP('',(#17519,#17520,#17521,#17522));
#4694=EDGE_LOOP('',(#17523,#17524,#17525,#17526));
#4695=EDGE_LOOP('',(#17527,#17528,#17529,#17530));
#4696=EDGE_LOOP('',(#17531,#17532,#17533,#17534));
#4697=EDGE_LOOP('',(#17535,#17536,#17537,#17538));
#4698=EDGE_LOOP('',(#17539,#17540,#17541,#17542));
#4699=EDGE_LOOP('',(#17543,#17544,#17545,#17546));
#4700=EDGE_LOOP('',(#17547,#17548,#17549,#17550));
#4701=EDGE_LOOP('',(#17551,#17552,#17553,#17554));
#4702=EDGE_LOOP('',(#17555,#17556,#17557,#17558,#17559,#17560,#17561,#17562,
#17563,#17564,#17565,#17566,#17567,#17568,#17569,#17570,#17571,#17572,#17573,
#17574,#17575,#17576,#17577,#17578,#17579,#17580,#17581,#17582,#17583,#17584));
#4703=EDGE_LOOP('',(#17585,#17586,#17587,#17588));
#4704=EDGE_LOOP('',(#17589,#17590,#17591,#17592));
#4705=EDGE_LOOP('',(#17593,#17594,#17595,#17596));
#4706=EDGE_LOOP('',(#17597,#17598,#17599,#17600));
#4707=EDGE_LOOP('',(#17601,#17602,#17603,#17604));
#4708=EDGE_LOOP('',(#17605,#17606,#17607,#17608));
#4709=EDGE_LOOP('',(#17609,#17610,#17611,#17612));
#4710=EDGE_LOOP('',(#17613,#17614,#17615,#17616));
#4711=EDGE_LOOP('',(#17617,#17618,#17619,#17620));
#4712=EDGE_LOOP('',(#17621,#17622,#17623,#17624));
#4713=EDGE_LOOP('',(#17625,#17626,#17627,#17628));
#4714=EDGE_LOOP('',(#17629,#17630,#17631,#17632));
#4715=EDGE_LOOP('',(#17633,#17634,#17635,#17636));
#4716=EDGE_LOOP('',(#17637,#17638,#17639,#17640));
#4717=EDGE_LOOP('',(#17641,#17642,#17643,#17644));
#4718=EDGE_LOOP('',(#17645,#17646,#17647,#17648));
#4719=EDGE_LOOP('',(#17649,#17650,#17651,#17652));
#4720=EDGE_LOOP('',(#17653,#17654,#17655,#17656));
#4721=EDGE_LOOP('',(#17657,#17658,#17659,#17660,#17661,#17662,#17663,#17664));
#4722=EDGE_LOOP('',(#17665,#17666,#17667,#17668,#17669));
#4723=EDGE_LOOP('',(#17670,#17671,#17672,#17673));
#4724=EDGE_LOOP('',(#17674,#17675,#17676,#17677));
#4725=EDGE_LOOP('',(#17678,#17679,#17680,#17681));
#4726=EDGE_LOOP('',(#17682,#17683,#17684,#17685));
#4727=EDGE_LOOP('',(#17686,#17687,#17688,#17689));
#4728=EDGE_LOOP('',(#17690,#17691,#17692,#17693));
#4729=EDGE_LOOP('',(#17694,#17695,#17696,#17697));
#4730=EDGE_LOOP('',(#17698,#17699,#17700,#17701));
#4731=EDGE_LOOP('',(#17702,#17703,#17704,#17705));
#4732=EDGE_LOOP('',(#17706,#17707,#17708,#17709));
#4733=EDGE_LOOP('',(#17710,#17711,#17712,#17713));
#4734=EDGE_LOOP('',(#17714,#17715,#17716,#17717));
#4735=EDGE_LOOP('',(#17718,#17719,#17720,#17721));
#4736=EDGE_LOOP('',(#17722,#17723,#17724,#17725));
#4737=EDGE_LOOP('',(#17726,#17727,#17728,#17729));
#4738=EDGE_LOOP('',(#17730,#17731,#17732,#17733));
#4739=EDGE_LOOP('',(#17734,#17735,#17736,#17737));
#4740=EDGE_LOOP('',(#17738,#17739,#17740,#17741));
#4741=EDGE_LOOP('',(#17742,#17743,#17744,#17745));
#4742=EDGE_LOOP('',(#17746,#17747,#17748,#17749));
#4743=EDGE_LOOP('',(#17750,#17751,#17752,#17753));
#4744=EDGE_LOOP('',(#17754,#17755,#17756,#17757));
#4745=EDGE_LOOP('',(#17758,#17759,#17760,#17761));
#4746=EDGE_LOOP('',(#17762,#17763,#17764,#17765));
#4747=EDGE_LOOP('',(#17766,#17767,#17768,#17769));
#4748=EDGE_LOOP('',(#17770,#17771,#17772,#17773));
#4749=EDGE_LOOP('',(#17774,#17775,#17776,#17777));
#4750=EDGE_LOOP('',(#17778,#17779,#17780,#17781));
#4751=EDGE_LOOP('',(#17782,#17783,#17784,#17785));
#4752=EDGE_LOOP('',(#17786,#17787,#17788,#17789));
#4753=EDGE_LOOP('',(#17790,#17791,#17792,#17793));
#4754=EDGE_LOOP('',(#17794,#17795,#17796,#17797));
#4755=EDGE_LOOP('',(#17798,#17799,#17800,#17801));
#4756=EDGE_LOOP('',(#17802,#17803,#17804,#17805));
#4757=EDGE_LOOP('',(#17806,#17807,#17808,#17809));
#4758=EDGE_LOOP('',(#17810,#17811,#17812,#17813,#17814,#17815,#17816,#17817,
#17818,#17819,#17820,#17821,#17822,#17823,#17824,#17825,#17826,#17827,#17828,
#17829,#17830,#17831,#17832,#17833,#17834,#17835,#17836,#17837,#17838,#17839,
#17840,#17841,#17842,#17843,#17844));
#4759=EDGE_LOOP('',(#17845,#17846,#17847,#17848));
#4760=EDGE_LOOP('',(#17849,#17850,#17851,#17852));
#4761=EDGE_LOOP('',(#17853,#17854,#17855,#17856));
#4762=EDGE_LOOP('',(#17857,#17858,#17859,#17860));
#4763=EDGE_LOOP('',(#17861,#17862,#17863,#17864));
#4764=EDGE_LOOP('',(#17865,#17866,#17867,#17868));
#4765=EDGE_LOOP('',(#17869,#17870,#17871,#17872));
#4766=EDGE_LOOP('',(#17873,#17874,#17875,#17876));
#4767=EDGE_LOOP('',(#17877,#17878,#17879,#17880));
#4768=EDGE_LOOP('',(#17881,#17882,#17883,#17884));
#4769=EDGE_LOOP('',(#17885,#17886,#17887,#17888));
#4770=EDGE_LOOP('',(#17889,#17890,#17891,#17892));
#4771=EDGE_LOOP('',(#17893,#17894,#17895,#17896));
#4772=EDGE_LOOP('',(#17897,#17898,#17899,#17900));
#4773=EDGE_LOOP('',(#17901,#17902,#17903,#17904));
#4774=EDGE_LOOP('',(#17905,#17906,#17907,#17908));
#4775=EDGE_LOOP('',(#17909,#17910,#17911,#17912));
#4776=EDGE_LOOP('',(#17913,#17914,#17915,#17916));
#4777=EDGE_LOOP('',(#17917,#17918,#17919,#17920));
#4778=EDGE_LOOP('',(#17921,#17922,#17923,#17924));
#4779=EDGE_LOOP('',(#17925,#17926,#17927,#17928));
#4780=EDGE_LOOP('',(#17929,#17930,#17931,#17932));
#4781=EDGE_LOOP('',(#17933,#17934,#17935,#17936));
#4782=EDGE_LOOP('',(#17937,#17938,#17939,#17940));
#4783=EDGE_LOOP('',(#17941,#17942,#17943,#17944));
#4784=EDGE_LOOP('',(#17945,#17946,#17947,#17948));
#4785=EDGE_LOOP('',(#17949,#17950,#17951,#17952));
#4786=EDGE_LOOP('',(#17953,#17954,#17955,#17956));
#4787=EDGE_LOOP('',(#17957,#17958,#17959,#17960));
#4788=EDGE_LOOP('',(#17961,#17962,#17963,#17964));
#4789=EDGE_LOOP('',(#17965,#17966,#17967,#17968,#17969,#17970,#17971,#17972,
#17973,#17974,#17975,#17976,#17977,#17978,#17979,#17980,#17981,#17982,#17983,
#17984,#17985,#17986,#17987,#17988,#17989,#17990,#17991,#17992,#17993,#17994));
#4790=EDGE_LOOP('',(#17995,#17996,#17997,#17998));
#4791=EDGE_LOOP('',(#17999,#18000,#18001,#18002));
#4792=EDGE_LOOP('',(#18003,#18004,#18005,#18006));
#4793=EDGE_LOOP('',(#18007,#18008,#18009,#18010));
#4794=EDGE_LOOP('',(#18011,#18012,#18013,#18014));
#4795=EDGE_LOOP('',(#18015,#18016,#18017,#18018));
#4796=EDGE_LOOP('',(#18019,#18020,#18021,#18022));
#4797=EDGE_LOOP('',(#18023,#18024,#18025,#18026));
#4798=EDGE_LOOP('',(#18027,#18028,#18029,#18030));
#4799=EDGE_LOOP('',(#18031,#18032,#18033,#18034));
#4800=EDGE_LOOP('',(#18035,#18036,#18037,#18038));
#4801=EDGE_LOOP('',(#18039,#18040,#18041,#18042));
#4802=EDGE_LOOP('',(#18043,#18044,#18045,#18046));
#4803=EDGE_LOOP('',(#18047,#18048,#18049,#18050));
#4804=EDGE_LOOP('',(#18051,#18052,#18053,#18054));
#4805=EDGE_LOOP('',(#18055,#18056,#18057,#18058));
#4806=EDGE_LOOP('',(#18059,#18060,#18061,#18062));
#4807=EDGE_LOOP('',(#18063,#18064,#18065,#18066));
#4808=EDGE_LOOP('',(#18067,#18068,#18069,#18070));
#4809=EDGE_LOOP('',(#18071,#18072,#18073,#18074));
#4810=EDGE_LOOP('',(#18075,#18076,#18077,#18078));
#4811=EDGE_LOOP('',(#18079,#18080,#18081,#18082));
#4812=EDGE_LOOP('',(#18083,#18084,#18085,#18086,#18087,#18088,#18089,#18090,
#18091,#18092,#18093,#18094,#18095,#18096,#18097,#18098,#18099,#18100,#18101,
#18102,#18103,#18104));
#4813=EDGE_LOOP('',(#18105,#18106,#18107,#18108));
#4814=EDGE_LOOP('',(#18109,#18110,#18111,#18112));
#4815=EDGE_LOOP('',(#18113,#18114,#18115,#18116));
#4816=EDGE_LOOP('',(#18117,#18118,#18119,#18120));
#4817=EDGE_LOOP('',(#18121,#18122,#18123,#18124));
#4818=EDGE_LOOP('',(#18125,#18126,#18127,#18128));
#4819=EDGE_LOOP('',(#18129,#18130,#18131,#18132));
#4820=EDGE_LOOP('',(#18133,#18134,#18135,#18136));
#4821=EDGE_LOOP('',(#18137,#18138,#18139,#18140));
#4822=EDGE_LOOP('',(#18141,#18142,#18143,#18144));
#4823=EDGE_LOOP('',(#18145,#18146,#18147,#18148));
#4824=EDGE_LOOP('',(#18149,#18150,#18151,#18152));
#4825=EDGE_LOOP('',(#18153,#18154,#18155,#18156));
#4826=EDGE_LOOP('',(#18157,#18158,#18159,#18160));
#4827=EDGE_LOOP('',(#18161,#18162,#18163,#18164));
#4828=EDGE_LOOP('',(#18165,#18166,#18167,#18168));
#4829=EDGE_LOOP('',(#18169,#18170,#18171,#18172));
#4830=EDGE_LOOP('',(#18173,#18174,#18175,#18176));
#4831=EDGE_LOOP('',(#18177,#18178,#18179,#18180));
#4832=EDGE_LOOP('',(#18181,#18182,#18183,#18184,#18185,#18186,#18187,#18188,
#18189,#18190,#18191));
#4833=EDGE_LOOP('',(#18192,#18193,#18194,#18195,#18196,#18197,#18198,#18199));
#4834=EDGE_LOOP('',(#18200,#18201,#18202,#18203));
#4835=EDGE_LOOP('',(#18204,#18205,#18206,#18207));
#4836=EDGE_LOOP('',(#18208,#18209,#18210,#18211));
#4837=EDGE_LOOP('',(#18212,#18213,#18214,#18215));
#4838=EDGE_LOOP('',(#18216,#18217,#18218,#18219));
#4839=EDGE_LOOP('',(#18220,#18221,#18222,#18223));
#4840=EDGE_LOOP('',(#18224,#18225,#18226,#18227));
#4841=EDGE_LOOP('',(#18228,#18229,#18230,#18231));
#4842=EDGE_LOOP('',(#18232,#18233,#18234,#18235));
#4843=EDGE_LOOP('',(#18236,#18237,#18238,#18239));
#4844=EDGE_LOOP('',(#18240,#18241,#18242,#18243));
#4845=EDGE_LOOP('',(#18244,#18245,#18246,#18247));
#4846=EDGE_LOOP('',(#18248,#18249,#18250,#18251));
#4847=EDGE_LOOP('',(#18252,#18253,#18254,#18255));
#4848=EDGE_LOOP('',(#18256,#18257,#18258,#18259));
#4849=EDGE_LOOP('',(#18260,#18261,#18262,#18263));
#4850=EDGE_LOOP('',(#18264,#18265,#18266,#18267));
#4851=EDGE_LOOP('',(#18268,#18269,#18270,#18271));
#4852=EDGE_LOOP('',(#18272,#18273,#18274,#18275));
#4853=EDGE_LOOP('',(#18276,#18277,#18278,#18279));
#4854=EDGE_LOOP('',(#18280,#18281,#18282,#18283));
#4855=EDGE_LOOP('',(#18284,#18285,#18286,#18287));
#4856=EDGE_LOOP('',(#18288,#18289,#18290,#18291));
#4857=EDGE_LOOP('',(#18292,#18293,#18294,#18295));
#4858=EDGE_LOOP('',(#18296,#18297,#18298,#18299));
#4859=EDGE_LOOP('',(#18300,#18301,#18302,#18303));
#4860=EDGE_LOOP('',(#18304,#18305,#18306,#18307));
#4861=EDGE_LOOP('',(#18308,#18309,#18310,#18311));
#4862=EDGE_LOOP('',(#18312,#18313,#18314,#18315,#18316,#18317,#18318,#18319,
#18320,#18321,#18322,#18323,#18324,#18325,#18326,#18327,#18328,#18329,#18330));
#4863=EDGE_LOOP('',(#18331,#18332,#18333,#18334,#18335,#18336,#18337,#18338,
#18339));
#4864=EDGE_LOOP('',(#18340,#18341,#18342,#18343));
#4865=EDGE_LOOP('',(#18344,#18345,#18346,#18347));
#4866=EDGE_LOOP('',(#18348,#18349,#18350,#18351));
#4867=EDGE_LOOP('',(#18352,#18353,#18354,#18355));
#4868=EDGE_LOOP('',(#18356,#18357,#18358,#18359));
#4869=EDGE_LOOP('',(#18360,#18361,#18362,#18363));
#4870=EDGE_LOOP('',(#18364,#18365,#18366,#18367));
#4871=EDGE_LOOP('',(#18368,#18369,#18370,#18371));
#4872=EDGE_LOOP('',(#18372,#18373,#18374,#18375));
#4873=EDGE_LOOP('',(#18376,#18377,#18378,#18379));
#4874=EDGE_LOOP('',(#18380,#18381,#18382,#18383));
#4875=EDGE_LOOP('',(#18384,#18385,#18386,#18387));
#4876=EDGE_LOOP('',(#18388,#18389,#18390,#18391));
#4877=EDGE_LOOP('',(#18392,#18393,#18394,#18395));
#4878=EDGE_LOOP('',(#18396,#18397,#18398,#18399));
#4879=EDGE_LOOP('',(#18400,#18401,#18402,#18403));
#4880=EDGE_LOOP('',(#18404,#18405,#18406,#18407));
#4881=EDGE_LOOP('',(#18408,#18409,#18410,#18411));
#4882=EDGE_LOOP('',(#18412,#18413,#18414,#18415));
#4883=EDGE_LOOP('',(#18416,#18417,#18418,#18419));
#4884=EDGE_LOOP('',(#18420,#18421,#18422,#18423));
#4885=EDGE_LOOP('',(#18424,#18425,#18426,#18427,#18428,#18429,#18430,#18431,
#18432,#18433,#18434,#18435,#18436));
#4886=EDGE_LOOP('',(#18437,#18438,#18439,#18440,#18441,#18442,#18443,#18444));
#4887=EDGE_LOOP('',(#18445,#18446,#18447,#18448));
#4888=EDGE_LOOP('',(#18449,#18450,#18451,#18452));
#4889=EDGE_LOOP('',(#18453,#18454,#18455,#18456));
#4890=EDGE_LOOP('',(#18457,#18458,#18459,#18460));
#4891=EDGE_LOOP('',(#18461,#18462,#18463,#18464));
#4892=EDGE_LOOP('',(#18465,#18466,#18467,#18468));
#4893=EDGE_LOOP('',(#18469,#18470,#18471,#18472));
#4894=EDGE_LOOP('',(#18473,#18474,#18475,#18476));
#4895=EDGE_LOOP('',(#18477,#18478,#18479,#18480));
#4896=EDGE_LOOP('',(#18481,#18482,#18483,#18484));
#4897=EDGE_LOOP('',(#18485,#18486,#18487,#18488));
#4898=EDGE_LOOP('',(#18489,#18490,#18491,#18492));
#4899=EDGE_LOOP('',(#18493,#18494,#18495,#18496));
#4900=EDGE_LOOP('',(#18497,#18498,#18499,#18500,#18501,#18502,#18503,#18504,
#18505,#18506,#18507,#18508,#18509));
#4901=EDGE_LOOP('',(#18510,#18511,#18512,#18513,#18514,#18515,#18516,#18517));
#4902=EDGE_LOOP('',(#18518,#18519,#18520,#18521,#18522,#18523,#18524,#18525,
#18526));
#4903=EDGE_LOOP('',(#18527,#18528,#18529,#18530,#18531,#18532,#18533,#18534));
#4904=EDGE_LOOP('',(#18535,#18536,#18537,#18538,#18539));
#4905=EDGE_LOOP('',(#18540,#18541,#18542,#18543,#18544,#18545,#18546,#18547));
#4906=EDGE_LOOP('',(#18548,#18549,#18550,#18551,#18552,#18553,#18554,#18555,
#18556,#18557));
#4907=EDGE_LOOP('',(#18558,#18559,#18560,#18561,#18562,#18563,#18564));
#4908=EDGE_LOOP('',(#18565,#18566,#18567,#18568));
#4909=EDGE_LOOP('',(#18569,#18570,#18571,#18572));
#4910=EDGE_LOOP('',(#18573,#18574,#18575,#18576));
#4911=EDGE_LOOP('',(#18577));
#4912=EDGE_LOOP('',(#18578,#18579,#18580));
#4913=EDGE_LOOP('',(#18581,#18582,#18583,#18584,#18585,#18586,#18587,#18588,
#18589,#18590));
#4914=EDGE_LOOP('',(#18591));
#4915=EDGE_LOOP('',(#18592));
#4916=EDGE_LOOP('',(#18593,#18594));
#4917=EDGE_LOOP('',(#18595,#18596,#18597,#18598,#18599,#18600,#18601,#18602));
#4918=EDGE_LOOP('',(#18603,#18604,#18605,#18606,#18607,#18608));
#4919=EDGE_LOOP('',(#18609,#18610,#18611,#18612));
#4920=EDGE_LOOP('',(#18613));
#4921=EDGE_LOOP('',(#18614));
#4922=EDGE_LOOP('',(#18615));
#4923=EDGE_LOOP('',(#18616));
#4924=EDGE_LOOP('',(#18617));
#4925=EDGE_LOOP('',(#18618));
#4926=EDGE_LOOP('',(#18619));
#4927=EDGE_LOOP('',(#18620));
#4928=EDGE_LOOP('',(#18621));
#4929=EDGE_LOOP('',(#18622,#18623,#18624,#18625));
#4930=EDGE_LOOP('',(#18626,#18627,#18628,#18629));
#4931=EDGE_LOOP('',(#18630,#18631,#18632,#18633));
#4932=EDGE_LOOP('',(#18634,#18635,#18636,#18637));
#4933=EDGE_LOOP('',(#18638,#18639,#18640,#18641));
#4934=EDGE_LOOP('',(#18642,#18643,#18644,#18645));
#4935=EDGE_LOOP('',(#18646,#18647,#18648,#18649));
#4936=EDGE_LOOP('',(#18650,#18651,#18652,#18653));
#4937=EDGE_LOOP('',(#18654,#18655,#18656,#18657));
#4938=EDGE_LOOP('',(#18658,#18659,#18660,#18661));
#4939=EDGE_LOOP('',(#18662,#18663,#18664,#18665));
#4940=EDGE_LOOP('',(#18666,#18667,#18668));
#4941=EDGE_LOOP('',(#18669,#18670,#18671));
#4942=EDGE_LOOP('',(#18672,#18673,#18674));
#4943=EDGE_LOOP('',(#18675,#18676,#18677));
#4944=EDGE_LOOP('',(#18678,#18679,#18680));
#4945=EDGE_LOOP('',(#18681,#18682,#18683));
#4946=EDGE_LOOP('',(#18684,#18685,#18686,#18687,#18688));
#4947=EDGE_LOOP('',(#18689,#18690,#18691,#18692,#18693));
#4948=EDGE_LOOP('',(#18694));
#4949=EDGE_LOOP('',(#18695,#18696,#18697,#18698,#18699,#18700,#18701,#18702,
#18703,#18704,#18705,#18706,#18707));
#4950=EDGE_LOOP('',(#18708,#18709,#18710,#18711,#18712,#18713,#18714,#18715,
#18716,#18717,#18718,#18719,#18720));
#4951=EDGE_LOOP('',(#18721,#18722,#18723,#18724,#18725,#18726,#18727,#18728,
#18729,#18730,#18731,#18732,#18733,#18734,#18735,#18736,#18737,#18738,#18739));
#4952=EDGE_LOOP('',(#18740,#18741,#18742,#18743,#18744,#18745,#18746,#18747,
#18748,#18749,#18750));
#4953=EDGE_LOOP('',(#18751,#18752,#18753,#18754,#18755,#18756,#18757,#18758,
#18759,#18760,#18761,#18762,#18763,#18764,#18765,#18766,#18767,#18768,#18769,
#18770,#18771,#18772));
#4954=EDGE_LOOP('',(#18773,#18774,#18775,#18776,#18777,#18778,#18779,#18780,
#18781,#18782,#18783,#18784,#18785,#18786,#18787,#18788,#18789,#18790,#18791,
#18792,#18793,#18794,#18795,#18796,#18797,#18798,#18799,#18800,#18801,#18802));
#4955=EDGE_LOOP('',(#18803,#18804,#18805,#18806,#18807,#18808,#18809,#18810,
#18811,#18812,#18813,#18814,#18815,#18816,#18817,#18818,#18819,#18820,#18821,
#18822,#18823,#18824,#18825,#18826,#18827,#18828,#18829,#18830,#18831,#18832,
#18833,#18834,#18835,#18836,#18837));
#4956=EDGE_LOOP('',(#18838,#18839,#18840,#18841,#18842,#18843,#18844,#18845));
#4957=EDGE_LOOP('',(#18846,#18847,#18848,#18849));
#4958=EDGE_LOOP('',(#18850,#18851,#18852,#18853,#18854,#18855,#18856,#18857,
#18858,#18859,#18860,#18861,#18862,#18863,#18864,#18865,#18866,#18867,#18868,
#18869,#18870,#18871,#18872,#18873,#18874,#18875,#18876,#18877,#18878,#18879));
#4959=EDGE_LOOP('',(#18880,#18881,#18882,#18883,#18884,#18885,#18886,#18887,
#18888,#18889,#18890,#18891,#18892,#18893,#18894));
#4960=EDGE_LOOP('',(#18895,#18896,#18897,#18898,#18899,#18900,#18901,#18902,
#18903));
#4961=EDGE_LOOP('',(#18904,#18905,#18906,#18907,#18908,#18909,#18910,#18911,
#18912,#18913,#18914,#18915));
#4962=EDGE_LOOP('',(#18916,#18917,#18918,#18919,#18920,#18921,#18922,#18923,
#18924,#18925,#18926,#18927,#18928,#18929,#18930,#18931,#18932,#18933,#18934,
#18935,#18936,#18937,#18938,#18939,#18940,#18941,#18942));
#4963=EDGE_LOOP('',(#18943,#18944,#18945,#18946));
#4964=EDGE_LOOP('',(#18947));
#4965=EDGE_LOOP('',(#18948,#18949,#18950,#18951));
#4966=EDGE_LOOP('',(#18952));
#4967=EDGE_LOOP('',(#18953));
#6023=LINE('',#43228,#7456);
#6024=LINE('',#43233,#7457);
#6025=LINE('',#43245,#7458);
#6026=LINE('',#43260,#7459);
#6027=LINE('',#43275,#7460);
#6028=LINE('',#43290,#7461);
#6029=LINE('',#43305,#7462);
#6030=LINE('',#43320,#7463);
#6031=LINE('',#43335,#7464);
#6032=LINE('',#43350,#7465);
#6033=LINE('',#43355,#7466);
#6034=LINE('',#43356,#7467);
#6035=LINE('',#43369,#7468);
#6036=LINE('',#43374,#7469);
#6037=LINE('',#43386,#7470);
#6038=LINE('',#43392,#7471);
#6039=LINE('',#43394,#7472);
#6040=LINE('',#43395,#7473);
#6041=LINE('',#43407,#7474);
#6042=LINE('',#43422,#7475);
#6043=LINE('',#43437,#7476);
#6044=LINE('',#43452,#7477);
#6045=LINE('',#43467,#7478);
#6046=LINE('',#43482,#7479);
#6047=LINE('',#43497,#7480);
#6048=LINE('',#43503,#7481);
#6049=LINE('',#43505,#7482);
#6050=LINE('',#43506,#7483);
#6051=LINE('',#43518,#7484);
#6052=LINE('',#43533,#7485);
#6053=LINE('',#43548,#7486);
#6054=LINE('',#43563,#7487);
#6055=LINE('',#43578,#7488);
#6056=LINE('',#43593,#7489);
#6057=LINE('',#43608,#7490);
#6058=LINE('',#43623,#7491);
#6059=LINE('',#43638,#7492);
#6060=LINE('',#43653,#7493);
#6061=LINE('',#43668,#7494);
#6062=LINE('',#43683,#7495);
#6063=LINE('',#43698,#7496);
#6064=LINE('',#43713,#7497);
#6065=LINE('',#43728,#7498);
#6066=LINE('',#43733,#7499);
#6067=LINE('',#43734,#7500);
#6068=LINE('',#43748,#7501);
#6069=LINE('',#43753,#7502);
#6070=LINE('',#43765,#7503);
#6071=LINE('',#43780,#7504);
#6072=LINE('',#43795,#7505);
#6073=LINE('',#43810,#7506);
#6074=LINE('',#43825,#7507);
#6075=LINE('',#43840,#7508);
#6076=LINE('',#43868,#7509);
#6077=LINE('',#43873,#7510);
#6078=LINE('',#43885,#7511);
#6079=LINE('',#43900,#7512);
#6080=LINE('',#43915,#7513);
#6081=LINE('',#43930,#7514);
#6082=LINE('',#43945,#7515);
#6083=LINE('',#43960,#7516);
#6084=LINE('',#43975,#7517);
#6085=LINE('',#43990,#7518);
#6086=LINE('',#44005,#7519);
#6087=LINE('',#44020,#7520);
#6088=LINE('',#44049,#7521);
#6089=LINE('',#44054,#7522);
#6090=LINE('',#44066,#7523);
#6091=LINE('',#44072,#7524);
#6092=LINE('',#44074,#7525);
#6093=LINE('',#44075,#7526);
#6094=LINE('',#44087,#7527);
#6095=LINE('',#44102,#7528);
#6096=LINE('',#44108,#7529);
#6097=LINE('',#44110,#7530);
#6098=LINE('',#44111,#7531);
#6099=LINE('',#44114,#7532);
#6100=LINE('',#44116,#7533);
#6101=LINE('',#44117,#7534);
#6102=LINE('',#44120,#7535);
#6103=LINE('',#44122,#7536);
#6104=LINE('',#44123,#7537);
#6105=LINE('',#44125,#7538);
#6106=LINE('',#44126,#7539);
#6107=LINE('',#44131,#7540);
#6108=LINE('',#44133,#7541);
#6109=LINE('',#44135,#7542);
#6110=LINE('',#44136,#7543);
#6111=LINE('',#44139,#7544);
#6112=LINE('',#44141,#7545);
#6113=LINE('',#44142,#7546);
#6114=LINE('',#44145,#7547);
#6115=LINE('',#44147,#7548);
#6116=LINE('',#44148,#7549);
#6117=LINE('',#44151,#7550);
#6118=LINE('',#44153,#7551);
#6119=LINE('',#44154,#7552);
#6120=LINE('',#44157,#7553);
#6121=LINE('',#44159,#7554);
#6122=LINE('',#44160,#7555);
#6123=LINE('',#44163,#7556);
#6124=LINE('',#44165,#7557);
#6125=LINE('',#44166,#7558);
#6126=LINE('',#44169,#7559);
#6127=LINE('',#44171,#7560);
#6128=LINE('',#44172,#7561);
#6129=LINE('',#44175,#7562);
#6130=LINE('',#44177,#7563);
#6131=LINE('',#44178,#7564);
#6132=LINE('',#44190,#7565);
#6133=LINE('',#44205,#7566);
#6134=LINE('',#44211,#7567);
#6135=LINE('',#44213,#7568);
#6136=LINE('',#44214,#7569);
#6137=LINE('',#44217,#7570);
#6138=LINE('',#44219,#7571);
#6139=LINE('',#44220,#7572);
#6140=LINE('',#44223,#7573);
#6141=LINE('',#44225,#7574);
#6142=LINE('',#44226,#7575);
#6143=LINE('',#44229,#7576);
#6144=LINE('',#44231,#7577);
#6145=LINE('',#44232,#7578);
#6146=LINE('',#44234,#7579);
#6147=LINE('',#44235,#7580);
#6148=LINE('',#44249,#7581);
#6149=LINE('',#44254,#7582);
#6150=LINE('',#44266,#7583);
#6151=LINE('',#44281,#7584);
#6152=LINE('',#44296,#7585);
#6153=LINE('',#44311,#7586);
#6154=LINE('',#44326,#7587);
#6155=LINE('',#44341,#7588);
#6156=LINE('',#44356,#7589);
#6157=LINE('',#44371,#7590);
#6158=LINE('',#44386,#7591);
#6159=LINE('',#44401,#7592);
#6160=LINE('',#44407,#7593);
#6161=LINE('',#44409,#7594);
#6162=LINE('',#44410,#7595);
#6163=LINE('',#44422,#7596);
#6164=LINE('',#44437,#7597);
#6165=LINE('',#44452,#7598);
#6166=LINE('',#44467,#7599);
#6167=LINE('',#44482,#7600);
#6168=LINE('',#44497,#7601);
#6169=LINE('',#44512,#7602);
#6170=LINE('',#44518,#7603);
#6171=LINE('',#44520,#7604);
#6172=LINE('',#44521,#7605);
#6173=LINE('',#44533,#7606);
#6174=LINE('',#44548,#7607);
#6175=LINE('',#44563,#7608);
#6176=LINE('',#44578,#7609);
#6177=LINE('',#44593,#7610);
#6178=LINE('',#44608,#7611);
#6179=LINE('',#44623,#7612);
#6180=LINE('',#44629,#7613);
#6181=LINE('',#44631,#7614);
#6182=LINE('',#44632,#7615);
#6183=LINE('',#44644,#7616);
#6184=LINE('',#44664,#7617);
#6185=LINE('',#44666,#7618);
#6186=LINE('',#44668,#7619);
#6187=LINE('',#44669,#7620);
#6188=LINE('',#44672,#7621);
#6189=LINE('',#44674,#7622);
#6190=LINE('',#44675,#7623);
#6191=LINE('',#44678,#7624);
#6192=LINE('',#44680,#7625);
#6193=LINE('',#44681,#7626);
#6194=LINE('',#44683,#7627);
#6195=LINE('',#44684,#7628);
#6196=LINE('',#44698,#7629);
#6197=LINE('',#44703,#7630);
#6198=LINE('',#44715,#7631);
#6199=LINE('',#44721,#7632);
#6200=LINE('',#44723,#7633);
#6201=LINE('',#44724,#7634);
#6202=LINE('',#44727,#7635);
#6203=LINE('',#44729,#7636);
#6204=LINE('',#44730,#7637);
#6205=LINE('',#44732,#7638);
#6206=LINE('',#44733,#7639);
#6207=LINE('',#44737,#7640);
#6208=LINE('',#44739,#7641);
#6209=LINE('',#44741,#7642);
#6210=LINE('',#44742,#7643);
#6211=LINE('',#44745,#7644);
#6212=LINE('',#44747,#7645);
#6213=LINE('',#44748,#7646);
#6214=LINE('',#44751,#7647);
#6215=LINE('',#44753,#7648);
#6216=LINE('',#44754,#7649);
#6217=LINE('',#44757,#7650);
#6218=LINE('',#44759,#7651);
#6219=LINE('',#44760,#7652);
#6220=LINE('',#44763,#7653);
#6221=LINE('',#44765,#7654);
#6222=LINE('',#44766,#7655);
#6223=LINE('',#44769,#7656);
#6224=LINE('',#44771,#7657);
#6225=LINE('',#44772,#7658);
#6226=LINE('',#44775,#7659);
#6227=LINE('',#44777,#7660);
#6228=LINE('',#44778,#7661);
#6229=LINE('',#44780,#7662);
#6230=LINE('',#44781,#7663);
#6231=LINE('',#44795,#7664);
#6232=LINE('',#44800,#7665);
#6233=LINE('',#44812,#7666);
#6234=LINE('',#44827,#7667);
#6235=LINE('',#44842,#7668);
#6236=LINE('',#44857,#7669);
#6237=LINE('',#44872,#7670);
#6238=LINE('',#44887,#7671);
#6239=LINE('',#44902,#7672);
#6240=LINE('',#44917,#7673);
#6241=LINE('',#44932,#7674);
#6242=LINE('',#44947,#7675);
#6243=LINE('',#44962,#7676);
#6244=LINE('',#44977,#7677);
#6245=LINE('',#44983,#7678);
#6246=LINE('',#44985,#7679);
#6247=LINE('',#44986,#7680);
#6248=LINE('',#44998,#7681);
#6249=LINE('',#45013,#7682);
#6250=LINE('',#45028,#7683);
#6251=LINE('',#45043,#7684);
#6252=LINE('',#45058,#7685);
#6253=LINE('',#45073,#7686);
#6254=LINE('',#45088,#7687);
#6255=LINE('',#45103,#7688);
#6256=LINE('',#45118,#7689);
#6257=LINE('',#45133,#7690);
#6258=LINE('',#45148,#7691);
#6259=LINE('',#45163,#7692);
#6260=LINE('',#45178,#7693);
#6261=LINE('',#45193,#7694);
#6262=LINE('',#45208,#7695);
#6263=LINE('',#45223,#7696);
#6264=LINE('',#45238,#7697);
#6265=LINE('',#45253,#7698);
#6266=LINE('',#45259,#7699);
#6267=LINE('',#45261,#7700);
#6268=LINE('',#45262,#7701);
#6269=LINE('',#45274,#7702);
#6270=LINE('',#45303,#7703);
#6271=LINE('',#45308,#7704);
#6272=LINE('',#45320,#7705);
#6273=LINE('',#45335,#7706);
#6274=LINE('',#45350,#7707);
#6275=LINE('',#45365,#7708);
#6276=LINE('',#45380,#7709);
#6277=LINE('',#45395,#7710);
#6278=LINE('',#45410,#7711);
#6279=LINE('',#45425,#7712);
#6280=LINE('',#45440,#7713);
#6281=LINE('',#45455,#7714);
#6282=LINE('',#45461,#7715);
#6283=LINE('',#45463,#7716);
#6284=LINE('',#45464,#7717);
#6285=LINE('',#45476,#7718);
#6286=LINE('',#45491,#7719);
#6287=LINE('',#45506,#7720);
#6288=LINE('',#45521,#7721);
#6289=LINE('',#45536,#7722);
#6290=LINE('',#45551,#7723);
#6291=LINE('',#45566,#7724);
#6292=LINE('',#45572,#7725);
#6293=LINE('',#45574,#7726);
#6294=LINE('',#45575,#7727);
#6295=LINE('',#45587,#7728);
#6296=LINE('',#45602,#7729);
#6297=LINE('',#45617,#7730);
#6298=LINE('',#45632,#7731);
#6299=LINE('',#45647,#7732);
#6300=LINE('',#45662,#7733);
#6301=LINE('',#45677,#7734);
#6302=LINE('',#45683,#7735);
#6303=LINE('',#45685,#7736);
#6304=LINE('',#45686,#7737);
#6305=LINE('',#45698,#7738);
#6306=LINE('',#45727,#7739);
#6307=LINE('',#45732,#7740);
#6308=LINE('',#45744,#7741);
#6309=LINE('',#45759,#7742);
#6310=LINE('',#45774,#7743);
#6311=LINE('',#45789,#7744);
#6312=LINE('',#45804,#7745);
#6313=LINE('',#45819,#7746);
#6314=LINE('',#45834,#7747);
#6315=LINE('',#45840,#7748);
#6316=LINE('',#45842,#7749);
#6317=LINE('',#45843,#7750);
#6318=LINE('',#45855,#7751);
#6319=LINE('',#45870,#7752);
#6320=LINE('',#45885,#7753);
#6321=LINE('',#45900,#7754);
#6322=LINE('',#45915,#7755);
#6323=LINE('',#45930,#7756);
#6324=LINE('',#45945,#7757);
#6325=LINE('',#45960,#7758);
#6326=LINE('',#45975,#7759);
#6327=LINE('',#45981,#7760);
#6328=LINE('',#45983,#7761);
#6329=LINE('',#45984,#7762);
#6330=LINE('',#45987,#7763);
#6331=LINE('',#45989,#7764);
#6332=LINE('',#45990,#7765);
#6333=LINE('',#45993,#7766);
#6334=LINE('',#45995,#7767);
#6335=LINE('',#45996,#7768);
#6336=LINE('',#46013,#7769);
#6337=LINE('',#46015,#7770);
#6338=LINE('',#46017,#7771);
#6339=LINE('',#46018,#7772);
#6340=LINE('',#46030,#7773);
#6341=LINE('',#46045,#7774);
#6342=LINE('',#46060,#7775);
#6343=LINE('',#46075,#7776);
#6344=LINE('',#46090,#7777);
#6345=LINE('',#46096,#7778);
#6346=LINE('',#46098,#7779);
#6347=LINE('',#46099,#7780);
#6348=LINE('',#46101,#7781);
#6349=LINE('',#46102,#7782);
#6350=LINE('',#46106,#7783);
#6351=LINE('',#46108,#7784);
#6352=LINE('',#46110,#7785);
#6353=LINE('',#46111,#7786);
#6354=LINE('',#46123,#7787);
#6355=LINE('',#46138,#7788);
#6356=LINE('',#46153,#7789);
#6357=LINE('',#46168,#7790);
#6358=LINE('',#46183,#7791);
#6359=LINE('',#46198,#7792);
#6360=LINE('',#46204,#7793);
#6361=LINE('',#46206,#7794);
#6362=LINE('',#46207,#7795);
#6363=LINE('',#46210,#7796);
#6364=LINE('',#46212,#7797);
#6365=LINE('',#46213,#7798);
#6366=LINE('',#46216,#7799);
#6367=LINE('',#46218,#7800);
#6368=LINE('',#46219,#7801);
#6369=LINE('',#46221,#7802);
#6370=LINE('',#46222,#7803);
#6371=LINE('',#46236,#7804);
#6372=LINE('',#46241,#7805);
#6373=LINE('',#46253,#7806);
#6374=LINE('',#46268,#7807);
#6375=LINE('',#46283,#7808);
#6376=LINE('',#46298,#7809);
#6377=LINE('',#46313,#7810);
#6378=LINE('',#46328,#7811);
#6379=LINE('',#46343,#7812);
#6380=LINE('',#46371,#7813);
#6381=LINE('',#46376,#7814);
#6382=LINE('',#46388,#7815);
#6383=LINE('',#46403,#7816);
#6384=LINE('',#46418,#7817);
#6385=LINE('',#46433,#7818);
#6386=LINE('',#46448,#7819);
#6387=LINE('',#46463,#7820);
#6388=LINE('',#46478,#7821);
#6389=LINE('',#46493,#7822);
#6390=LINE('',#46508,#7823);
#6391=LINE('',#46523,#7824);
#6392=LINE('',#46538,#7825);
#6393=LINE('',#46553,#7826);
#6394=LINE('',#46568,#7827);
#6395=LINE('',#46583,#7828);
#6396=LINE('',#46598,#7829);
#6397=LINE('',#46604,#7830);
#6398=LINE('',#46606,#7831);
#6399=LINE('',#46607,#7832);
#6400=LINE('',#46619,#7833);
#6401=LINE('',#46648,#7834);
#6402=LINE('',#46653,#7835);
#6403=LINE('',#46665,#7836);
#6404=LINE('',#46680,#7837);
#6405=LINE('',#46695,#7838);
#6406=LINE('',#46710,#7839);
#6407=LINE('',#46725,#7840);
#6408=LINE('',#46740,#7841);
#6409=LINE('',#46768,#7842);
#6410=LINE('',#46773,#7843);
#6411=LINE('',#46785,#7844);
#6412=LINE('',#46800,#7845);
#6413=LINE('',#46815,#7846);
#6414=LINE('',#46830,#7847);
#6415=LINE('',#46845,#7848);
#6416=LINE('',#46860,#7849);
#6417=LINE('',#46866,#7850);
#6418=LINE('',#46868,#7851);
#6419=LINE('',#46869,#7852);
#6420=LINE('',#46872,#7853);
#6421=LINE('',#46874,#7854);
#6422=LINE('',#46875,#7855);
#6423=LINE('',#46878,#7856);
#6424=LINE('',#46880,#7857);
#6425=LINE('',#46881,#7858);
#6426=LINE('',#46884,#7859);
#6427=LINE('',#46886,#7860);
#6428=LINE('',#46887,#7861);
#6429=LINE('',#46890,#7862);
#6430=LINE('',#46892,#7863);
#6431=LINE('',#46893,#7864);
#6432=LINE('',#46919,#7865);
#6433=LINE('',#46924,#7866);
#6434=LINE('',#46936,#7867);
#6435=LINE('',#46951,#7868);
#6436=LINE('',#46966,#7869);
#6437=LINE('',#46972,#7870);
#6438=LINE('',#46974,#7871);
#6439=LINE('',#46975,#7872);
#6440=LINE('',#46987,#7873);
#6441=LINE('',#47002,#7874);
#6442=LINE('',#47017,#7875);
#6443=LINE('',#47023,#7876);
#6444=LINE('',#47025,#7877);
#6445=LINE('',#47026,#7878);
#6446=LINE('',#47029,#7879);
#6447=LINE('',#47031,#7880);
#6448=LINE('',#47032,#7881);
#6449=LINE('',#47035,#7882);
#6450=LINE('',#47037,#7883);
#6451=LINE('',#47038,#7884);
#6452=LINE('',#47041,#7885);
#6453=LINE('',#47043,#7886);
#6454=LINE('',#47044,#7887);
#6455=LINE('',#47046,#7888);
#6456=LINE('',#47047,#7889);
#6457=LINE('',#47059,#7890);
#6458=LINE('',#47107,#7891);
#6459=LINE('',#47112,#7892);
#6460=LINE('',#47116,#7893);
#6461=LINE('',#47145,#7894);
#6462=LINE('',#47146,#7895);
#6463=LINE('',#47150,#7896);
#6464=LINE('',#47153,#7897);
#6465=LINE('',#47155,#7898);
#6466=LINE('',#47164,#7899);
#6467=LINE('',#47175,#7900);
#6468=LINE('',#47194,#7901);
#6469=LINE('',#47198,#7902);
#6470=LINE('',#47202,#7903);
#6471=LINE('',#47206,#7904);
#6472=LINE('',#47210,#7905);
#6473=LINE('',#47214,#7906);
#6474=LINE('',#47218,#7907);
#6475=LINE('',#47222,#7908);
#6476=LINE('',#47226,#7909);
#6477=LINE('',#47230,#7910);
#6478=LINE('',#47234,#7911);
#6479=LINE('',#47238,#7912);
#6480=LINE('',#47241,#7913);
#6481=LINE('',#47244,#7914);
#6482=LINE('',#47247,#7915);
#6483=LINE('',#47250,#7916);
#6484=LINE('',#47253,#7917);
#6485=LINE('',#47256,#7918);
#6486=LINE('',#47263,#7919);
#6487=LINE('',#47266,#7920);
#6488=LINE('',#47272,#7921);
#7456=VECTOR('',#27553,1.);
#7457=VECTOR('',#27554,1.);
#7458=VECTOR('',#27555,1.);
#7459=VECTOR('',#27556,1.);
#7460=VECTOR('',#27557,1.);
#7461=VECTOR('',#27558,1.);
#7462=VECTOR('',#27559,1.);
#7463=VECTOR('',#27560,1.);
#7464=VECTOR('',#27561,1.);
#7465=VECTOR('',#27562,1.);
#7466=VECTOR('',#27565,1.);
#7467=VECTOR('',#27566,1.);
#7468=VECTOR('',#27567,1.);
#7469=VECTOR('',#27568,1.);
#7470=VECTOR('',#27569,1.);
#7471=VECTOR('',#27572,1.);
#7472=VECTOR('',#27573,1.);
#7473=VECTOR('',#27574,1.);
#7474=VECTOR('',#27575,1.);
#7475=VECTOR('',#27576,1.);
#7476=VECTOR('',#27577,1.);
#7477=VECTOR('',#27578,1.);
#7478=VECTOR('',#27579,1.);
#7479=VECTOR('',#27580,1.);
#7480=VECTOR('',#27581,1.);
#7481=VECTOR('',#27584,1.);
#7482=VECTOR('',#27585,1.);
#7483=VECTOR('',#27586,1.);
#7484=VECTOR('',#27587,1.);
#7485=VECTOR('',#27588,1.);
#7486=VECTOR('',#27589,1.);
#7487=VECTOR('',#27590,1.);
#7488=VECTOR('',#27591,1.);
#7489=VECTOR('',#27592,1.);
#7490=VECTOR('',#27593,1.);
#7491=VECTOR('',#27594,1.);
#7492=VECTOR('',#27595,1.);
#7493=VECTOR('',#27596,1.);
#7494=VECTOR('',#27597,1.);
#7495=VECTOR('',#27598,1.);
#7496=VECTOR('',#27599,1.);
#7497=VECTOR('',#27600,1.);
#7498=VECTOR('',#27601,1.);
#7499=VECTOR('',#27604,1.);
#7500=VECTOR('',#27605,1.);
#7501=VECTOR('',#27608,1.);
#7502=VECTOR('',#27609,1.);
#7503=VECTOR('',#27610,1.);
#7504=VECTOR('',#27611,1.);
#7505=VECTOR('',#27612,1.);
#7506=VECTOR('',#27613,1.);
#7507=VECTOR('',#27614,1.);
#7508=VECTOR('',#27615,1.);
#7509=VECTOR('',#27616,1.);
#7510=VECTOR('',#27617,1.);
#7511=VECTOR('',#27618,1.);
#7512=VECTOR('',#27619,1.);
#7513=VECTOR('',#27620,1.);
#7514=VECTOR('',#27621,1.);
#7515=VECTOR('',#27622,1.);
#7516=VECTOR('',#27623,1.);
#7517=VECTOR('',#27624,1.);
#7518=VECTOR('',#27625,1.);
#7519=VECTOR('',#27626,1.);
#7520=VECTOR('',#27627,1.);
#7521=VECTOR('',#27630,1.);
#7522=VECTOR('',#27631,1.);
#7523=VECTOR('',#27632,1.);
#7524=VECTOR('',#27635,1.);
#7525=VECTOR('',#27636,1.);
#7526=VECTOR('',#27637,1.);
#7527=VECTOR('',#27638,1.);
#7528=VECTOR('',#27639,1.);
#7529=VECTOR('',#27642,1.);
#7530=VECTOR('',#27643,1.);
#7531=VECTOR('',#27644,1.);
#7532=VECTOR('',#27647,1.);
#7533=VECTOR('',#27648,1.);
#7534=VECTOR('',#27649,1.);
#7535=VECTOR('',#27652,1.);
#7536=VECTOR('',#27653,1.);
#7537=VECTOR('',#27654,1.);
#7538=VECTOR('',#27657,1.);
#7539=VECTOR('',#27658,1.);
#7540=VECTOR('',#27663,1.);
#7541=VECTOR('',#27664,1.);
#7542=VECTOR('',#27665,1.);
#7543=VECTOR('',#27666,1.);
#7544=VECTOR('',#27669,1.);
#7545=VECTOR('',#27670,1.);
#7546=VECTOR('',#27671,1.);
#7547=VECTOR('',#27674,1.);
#7548=VECTOR('',#27675,1.);
#7549=VECTOR('',#27676,1.);
#7550=VECTOR('',#27679,1.);
#7551=VECTOR('',#27680,1.);
#7552=VECTOR('',#27681,1.);
#7553=VECTOR('',#27684,1.);
#7554=VECTOR('',#27685,1.);
#7555=VECTOR('',#27686,1.);
#7556=VECTOR('',#27689,1.);
#7557=VECTOR('',#27690,1.);
#7558=VECTOR('',#27691,1.);
#7559=VECTOR('',#27694,1.);
#7560=VECTOR('',#27695,1.);
#7561=VECTOR('',#27696,1.);
#7562=VECTOR('',#27699,1.);
#7563=VECTOR('',#27700,1.);
#7564=VECTOR('',#27701,1.);
#7565=VECTOR('',#27702,1.);
#7566=VECTOR('',#27703,1.);
#7567=VECTOR('',#27706,1.);
#7568=VECTOR('',#27707,1.);
#7569=VECTOR('',#27708,1.);
#7570=VECTOR('',#27711,1.);
#7571=VECTOR('',#27712,1.);
#7572=VECTOR('',#27713,1.);
#7573=VECTOR('',#27716,1.);
#7574=VECTOR('',#27717,1.);
#7575=VECTOR('',#27718,1.);
#7576=VECTOR('',#27721,1.);
#7577=VECTOR('',#27722,1.);
#7578=VECTOR('',#27723,1.);
#7579=VECTOR('',#27726,1.);
#7580=VECTOR('',#27727,1.);
#7581=VECTOR('',#27730,1.);
#7582=VECTOR('',#27731,1.);
#7583=VECTOR('',#27732,1.);
#7584=VECTOR('',#27733,1.);
#7585=VECTOR('',#27734,1.);
#7586=VECTOR('',#27735,1.);
#7587=VECTOR('',#27736,1.);
#7588=VECTOR('',#27737,1.);
#7589=VECTOR('',#27738,1.);
#7590=VECTOR('',#27739,1.);
#7591=VECTOR('',#27740,1.);
#7592=VECTOR('',#27741,1.);
#7593=VECTOR('',#27744,1.);
#7594=VECTOR('',#27745,1.);
#7595=VECTOR('',#27746,1.);
#7596=VECTOR('',#27747,1.);
#7597=VECTOR('',#27748,1.);
#7598=VECTOR('',#27749,1.);
#7599=VECTOR('',#27750,1.);
#7600=VECTOR('',#27751,1.);
#7601=VECTOR('',#27752,1.);
#7602=VECTOR('',#27753,1.);
#7603=VECTOR('',#27756,1.);
#7604=VECTOR('',#27757,1.);
#7605=VECTOR('',#27758,1.);
#7606=VECTOR('',#27759,1.);
#7607=VECTOR('',#27760,1.);
#7608=VECTOR('',#27761,1.);
#7609=VECTOR('',#27762,1.);
#7610=VECTOR('',#27763,1.);
#7611=VECTOR('',#27764,1.);
#7612=VECTOR('',#27765,1.);
#7613=VECTOR('',#27768,1.);
#7614=VECTOR('',#27769,1.);
#7615=VECTOR('',#27770,1.);
#7616=VECTOR('',#27771,1.);
#7617=VECTOR('',#27776,1.);
#7618=VECTOR('',#27777,1.);
#7619=VECTOR('',#27778,1.);
#7620=VECTOR('',#27779,1.);
#7621=VECTOR('',#27782,1.);
#7622=VECTOR('',#27783,1.);
#7623=VECTOR('',#27784,1.);
#7624=VECTOR('',#27787,1.);
#7625=VECTOR('',#27788,1.);
#7626=VECTOR('',#27789,1.);
#7627=VECTOR('',#27792,1.);
#7628=VECTOR('',#27793,1.);
#7629=VECTOR('',#27796,1.);
#7630=VECTOR('',#27797,1.);
#7631=VECTOR('',#27798,1.);
#7632=VECTOR('',#27801,1.);
#7633=VECTOR('',#27802,1.);
#7634=VECTOR('',#27803,1.);
#7635=VECTOR('',#27806,1.);
#7636=VECTOR('',#27807,1.);
#7637=VECTOR('',#27808,1.);
#7638=VECTOR('',#27811,1.);
#7639=VECTOR('',#27812,1.);
#7640=VECTOR('',#27815,1.);
#7641=VECTOR('',#27816,1.);
#7642=VECTOR('',#27817,1.);
#7643=VECTOR('',#27818,1.);
#7644=VECTOR('',#27821,1.);
#7645=VECTOR('',#27822,1.);
#7646=VECTOR('',#27823,1.);
#7647=VECTOR('',#27826,1.);
#7648=VECTOR('',#27827,1.);
#7649=VECTOR('',#27828,1.);
#7650=VECTOR('',#27831,1.);
#7651=VECTOR('',#27832,1.);
#7652=VECTOR('',#27833,1.);
#7653=VECTOR('',#27836,1.);
#7654=VECTOR('',#27837,1.);
#7655=VECTOR('',#27838,1.);
#7656=VECTOR('',#27841,1.);
#7657=VECTOR('',#27842,1.);
#7658=VECTOR('',#27843,1.);
#7659=VECTOR('',#27846,1.);
#7660=VECTOR('',#27847,1.);
#7661=VECTOR('',#27848,1.);
#7662=VECTOR('',#27851,1.);
#7663=VECTOR('',#27852,1.);
#7664=VECTOR('',#27855,1.);
#7665=VECTOR('',#27856,1.);
#7666=VECTOR('',#27857,1.);
#7667=VECTOR('',#27858,1.);
#7668=VECTOR('',#27859,1.);
#7669=VECTOR('',#27860,1.);
#7670=VECTOR('',#27861,1.);
#7671=VECTOR('',#27862,1.);
#7672=VECTOR('',#27863,1.);
#7673=VECTOR('',#27864,1.);
#7674=VECTOR('',#27865,1.);
#7675=VECTOR('',#27866,1.);
#7676=VECTOR('',#27867,1.);
#7677=VECTOR('',#27868,1.);
#7678=VECTOR('',#27871,1.);
#7679=VECTOR('',#27872,1.);
#7680=VECTOR('',#27873,1.);
#7681=VECTOR('',#27874,1.);
#7682=VECTOR('',#27875,1.);
#7683=VECTOR('',#27876,1.);
#7684=VECTOR('',#27877,1.);
#7685=VECTOR('',#27878,1.);
#7686=VECTOR('',#27879,1.);
#7687=VECTOR('',#27880,1.);
#7688=VECTOR('',#27881,1.);
#7689=VECTOR('',#27882,1.);
#7690=VECTOR('',#27883,1.);
#7691=VECTOR('',#27884,1.);
#7692=VECTOR('',#27885,1.);
#7693=VECTOR('',#27886,1.);
#7694=VECTOR('',#27887,1.);
#7695=VECTOR('',#27888,1.);
#7696=VECTOR('',#27889,1.);
#7697=VECTOR('',#27890,1.);
#7698=VECTOR('',#27891,1.);
#7699=VECTOR('',#27894,1.);
#7700=VECTOR('',#27895,1.);
#7701=VECTOR('',#27896,1.);
#7702=VECTOR('',#27897,1.);
#7703=VECTOR('',#27900,1.);
#7704=VECTOR('',#27901,1.);
#7705=VECTOR('',#27902,1.);
#7706=VECTOR('',#27903,1.);
#7707=VECTOR('',#27904,1.);
#7708=VECTOR('',#27905,1.);
#7709=VECTOR('',#27906,1.);
#7710=VECTOR('',#27907,1.);
#7711=VECTOR('',#27908,1.);
#7712=VECTOR('',#27909,1.);
#7713=VECTOR('',#27910,1.);
#7714=VECTOR('',#27911,1.);
#7715=VECTOR('',#27914,1.);
#7716=VECTOR('',#27915,1.);
#7717=VECTOR('',#27916,1.);
#7718=VECTOR('',#27917,1.);
#7719=VECTOR('',#27918,1.);
#7720=VECTOR('',#27919,1.);
#7721=VECTOR('',#27920,1.);
#7722=VECTOR('',#27921,1.);
#7723=VECTOR('',#27922,1.);
#7724=VECTOR('',#27923,1.);
#7725=VECTOR('',#27926,1.);
#7726=VECTOR('',#27927,1.);
#7727=VECTOR('',#27928,1.);
#7728=VECTOR('',#27929,1.);
#7729=VECTOR('',#27930,1.);
#7730=VECTOR('',#27931,1.);
#7731=VECTOR('',#27932,1.);
#7732=VECTOR('',#27933,1.);
#7733=VECTOR('',#27934,1.);
#7734=VECTOR('',#27935,1.);
#7735=VECTOR('',#27938,1.);
#7736=VECTOR('',#27939,1.);
#7737=VECTOR('',#27940,1.);
#7738=VECTOR('',#27941,1.);
#7739=VECTOR('',#27944,1.);
#7740=VECTOR('',#27945,1.);
#7741=VECTOR('',#27946,1.);
#7742=VECTOR('',#27947,1.);
#7743=VECTOR('',#27948,1.);
#7744=VECTOR('',#27949,1.);
#7745=VECTOR('',#27950,1.);
#7746=VECTOR('',#27951,1.);
#7747=VECTOR('',#27952,1.);
#7748=VECTOR('',#27955,1.);
#7749=VECTOR('',#27956,1.);
#7750=VECTOR('',#27957,1.);
#7751=VECTOR('',#27958,1.);
#7752=VECTOR('',#27959,1.);
#7753=VECTOR('',#27960,1.);
#7754=VECTOR('',#27961,1.);
#7755=VECTOR('',#27962,1.);
#7756=VECTOR('',#27963,1.);
#7757=VECTOR('',#27964,1.);
#7758=VECTOR('',#27965,1.);
#7759=VECTOR('',#27966,1.);
#7760=VECTOR('',#27969,1.);
#7761=VECTOR('',#27970,1.);
#7762=VECTOR('',#27971,1.);
#7763=VECTOR('',#27974,1.);
#7764=VECTOR('',#27975,1.);
#7765=VECTOR('',#27976,1.);
#7766=VECTOR('',#27979,1.);
#7767=VECTOR('',#27980,1.);
#7768=VECTOR('',#27981,1.);
#7769=VECTOR('',#27986,1.);
#7770=VECTOR('',#27987,1.);
#7771=VECTOR('',#27988,1.);
#7772=VECTOR('',#27989,1.);
#7773=VECTOR('',#27990,1.);
#7774=VECTOR('',#27991,1.);
#7775=VECTOR('',#27992,1.);
#7776=VECTOR('',#27993,1.);
#7777=VECTOR('',#27994,1.);
#7778=VECTOR('',#27997,1.);
#7779=VECTOR('',#27998,1.);
#7780=VECTOR('',#27999,1.);
#7781=VECTOR('',#28002,1.);
#7782=VECTOR('',#28003,1.);
#7783=VECTOR('',#28006,1.);
#7784=VECTOR('',#28007,1.);
#7785=VECTOR('',#28008,1.);
#7786=VECTOR('',#28009,1.);
#7787=VECTOR('',#28010,1.);
#7788=VECTOR('',#28011,1.);
#7789=VECTOR('',#28012,1.);
#7790=VECTOR('',#28013,1.);
#7791=VECTOR('',#28014,1.);
#7792=VECTOR('',#28015,1.);
#7793=VECTOR('',#28018,1.);
#7794=VECTOR('',#28019,1.);
#7795=VECTOR('',#28020,1.);
#7796=VECTOR('',#28023,1.);
#7797=VECTOR('',#28024,1.);
#7798=VECTOR('',#28025,1.);
#7799=VECTOR('',#28028,1.);
#7800=VECTOR('',#28029,1.);
#7801=VECTOR('',#28030,1.);
#7802=VECTOR('',#28033,1.);
#7803=VECTOR('',#28034,1.);
#7804=VECTOR('',#28037,1.);
#7805=VECTOR('',#28038,1.);
#7806=VECTOR('',#28039,1.);
#7807=VECTOR('',#28040,1.);
#7808=VECTOR('',#28041,1.);
#7809=VECTOR('',#28042,1.);
#7810=VECTOR('',#28043,1.);
#7811=VECTOR('',#28044,1.);
#7812=VECTOR('',#28045,1.);
#7813=VECTOR('',#28046,1.);
#7814=VECTOR('',#28047,1.);
#7815=VECTOR('',#28048,1.);
#7816=VECTOR('',#28049,1.);
#7817=VECTOR('',#28050,1.);
#7818=VECTOR('',#28051,1.);
#7819=VECTOR('',#28052,1.);
#7820=VECTOR('',#28053,1.);
#7821=VECTOR('',#28054,1.);
#7822=VECTOR('',#28055,1.);
#7823=VECTOR('',#28056,1.);
#7824=VECTOR('',#28057,1.);
#7825=VECTOR('',#28058,1.);
#7826=VECTOR('',#28059,1.);
#7827=VECTOR('',#28060,1.);
#7828=VECTOR('',#28061,1.);
#7829=VECTOR('',#28062,1.);
#7830=VECTOR('',#28065,1.);
#7831=VECTOR('',#28066,1.);
#7832=VECTOR('',#28067,1.);
#7833=VECTOR('',#28068,1.);
#7834=VECTOR('',#28071,1.);
#7835=VECTOR('',#28072,1.);
#7836=VECTOR('',#28073,1.);
#7837=VECTOR('',#28074,1.);
#7838=VECTOR('',#28075,1.);
#7839=VECTOR('',#28076,1.);
#7840=VECTOR('',#28077,1.);
#7841=VECTOR('',#28078,1.);
#7842=VECTOR('',#28079,1.);
#7843=VECTOR('',#28080,1.);
#7844=VECTOR('',#28081,1.);
#7845=VECTOR('',#28082,1.);
#7846=VECTOR('',#28083,1.);
#7847=VECTOR('',#28084,1.);
#7848=VECTOR('',#28085,1.);
#7849=VECTOR('',#28086,1.);
#7850=VECTOR('',#28089,1.);
#7851=VECTOR('',#28090,1.);
#7852=VECTOR('',#28091,1.);
#7853=VECTOR('',#28094,1.);
#7854=VECTOR('',#28095,1.);
#7855=VECTOR('',#28096,1.);
#7856=VECTOR('',#28099,1.);
#7857=VECTOR('',#28100,1.);
#7858=VECTOR('',#28101,1.);
#7859=VECTOR('',#28104,1.);
#7860=VECTOR('',#28105,1.);
#7861=VECTOR('',#28106,1.);
#7862=VECTOR('',#28109,1.);
#7863=VECTOR('',#28110,1.);
#7864=VECTOR('',#28111,1.);
#7865=VECTOR('',#28114,1.);
#7866=VECTOR('',#28115,1.);
#7867=VECTOR('',#28116,1.);
#7868=VECTOR('',#28117,1.);
#7869=VECTOR('',#28118,1.);
#7870=VECTOR('',#28121,1.);
#7871=VECTOR('',#28122,1.);
#7872=VECTOR('',#28123,1.);
#7873=VECTOR('',#28124,1.);
#7874=VECTOR('',#28125,1.);
#7875=VECTOR('',#28126,1.);
#7876=VECTOR('',#28129,1.);
#7877=VECTOR('',#28130,1.);
#7878=VECTOR('',#28131,1.);
#7879=VECTOR('',#28134,1.);
#7880=VECTOR('',#28135,1.);
#7881=VECTOR('',#28136,1.);
#7882=VECTOR('',#28139,1.);
#7883=VECTOR('',#28140,1.);
#7884=VECTOR('',#28141,1.);
#7885=VECTOR('',#28144,1.);
#7886=VECTOR('',#28145,1.);
#7887=VECTOR('',#28146,1.);
#7888=VECTOR('',#28149,1.);
#7889=VECTOR('',#28150,1.);
#7890=VECTOR('',#28169,0.3);
#7891=VECTOR('',#28174,0.8781);
#7892=VECTOR('',#28181,0.8381);
#7893=VECTOR('',#28184,1.);
#7894=VECTOR('',#28185,1.);
#7895=VECTOR('',#28186,1.);
#7896=VECTOR('',#28189,0.25);
#7897=VECTOR('',#28194,0.5);
#7898=VECTOR('',#28195,0.5);
#7899=VECTOR('',#28208,7.);
#7900=VECTOR('',#28223,0.429999999999999);
#7901=VECTOR('',#28244,0.404999999999999);
#7902=VECTOR('',#28249,0.429999999999999);
#7903=VECTOR('',#28254,0.404999999999999);
#7904=VECTOR('',#28259,0.43);
#7905=VECTOR('',#28264,0.405);
#7906=VECTOR('',#28269,0.429999999999999);
#7907=VECTOR('',#28274,0.404999999999999);
#7908=VECTOR('',#28279,0.43);
#7909=VECTOR('',#28284,0.405);
#7910=VECTOR('',#28289,0.429999999999999);
#7911=VECTOR('',#28294,0.404999999999999);
#7912=VECTOR('',#28299,0.404999999999999);
#7913=VECTOR('',#28302,0.405);
#7914=VECTOR('',#28305,0.404999999999999);
#7915=VECTOR('',#28308,0.405);
#7916=VECTOR('',#28311,0.404999999999999);
#7917=VECTOR('',#28314,0.404999999999999);
#7918=VECTOR('',#28317,2.63);
#7919=VECTOR('',#28326,2.6);
#7920=VECTOR('',#28331,6.975);
#7921=VECTOR('',#28338,2.4);
#8818=CIRCLE('',#24087,0.3);
#8819=CIRCLE('',#24089,0.9181);
#8820=CIRCLE('',#24090,0.8381);
#8821=CIRCLE('',#24092,0.8381);
#8822=CIRCLE('',#24095,0.5);
#8823=CIRCLE('',#24097,0.5);
#8824=CIRCLE('',#24100,7.);
#8825=CIRCLE('',#24102,7.);
#8826=CIRCLE('',#24103,7.);
#8827=CIRCLE('',#24104,7.);
#8828=CIRCLE('',#24106,6.3);
#8829=CIRCLE('',#24107,0.7);
#8830=CIRCLE('',#24109,0.454999999999999);
#8831=CIRCLE('',#24110,0.404999999999999);
#8832=CIRCLE('',#24112,6.95);
#8833=CIRCLE('',#24113,0.455);
#8834=CIRCLE('',#24114,0.455);
#8835=CIRCLE('',#24115,2.66);
#8836=CIRCLE('',#24116,0.454999999999999);
#8837=CIRCLE('',#24117,0.454999999999999);
#8838=CIRCLE('',#24118,0.454999999999999);
#8839=CIRCLE('',#24120,0.404999999999999);
#8840=CIRCLE('',#24122,0.404999999999999);
#8841=CIRCLE('',#24124,0.404999999999999);
#8842=CIRCLE('',#24126,0.405);
#8843=CIRCLE('',#24128,0.405);
#8844=CIRCLE('',#24130,0.404999999999999);
#8845=CIRCLE('',#24132,0.404999999999999);
#8846=CIRCLE('',#24134,0.405);
#8847=CIRCLE('',#24136,0.405);
#8848=CIRCLE('',#24138,0.404999999999999);
#8849=CIRCLE('',#24140,0.404999999999999);
#8850=CIRCLE('',#24148,2.6);
#8851=CIRCLE('',#24149,2.6);
#8852=CIRCLE('',#24151,2.6);
#8853=CIRCLE('',#24155,2.4);
#8854=CIRCLE('',#24157,2.4);
#9941=VERTEX_POINT('',#43222);
#9942=VERTEX_POINT('',#43223);
#9943=VERTEX_POINT('',#43227);
#9944=VERTEX_POINT('',#43229);
#9945=VERTEX_POINT('',#43240);
#9946=VERTEX_POINT('',#43244);
#9947=VERTEX_POINT('',#43255);
#9948=VERTEX_POINT('',#43259);
#9949=VERTEX_POINT('',#43270);
#9950=VERTEX_POINT('',#43274);
#9951=VERTEX_POINT('',#43285);
#9952=VERTEX_POINT('',#43289);
#9953=VERTEX_POINT('',#43300);
#9954=VERTEX_POINT('',#43304);
#9955=VERTEX_POINT('',#43315);
#9956=VERTEX_POINT('',#43319);
#9957=VERTEX_POINT('',#43330);
#9958=VERTEX_POINT('',#43334);
#9959=VERTEX_POINT('',#43345);
#9960=VERTEX_POINT('',#43349);
#9961=VERTEX_POINT('',#43363);
#9962=VERTEX_POINT('',#43364);
#9963=VERTEX_POINT('',#43368);
#9964=VERTEX_POINT('',#43370);
#9965=VERTEX_POINT('',#43381);
#9966=VERTEX_POINT('',#43385);
#9967=VERTEX_POINT('',#43391);
#9968=VERTEX_POINT('',#43393);
#9969=VERTEX_POINT('',#43402);
#9970=VERTEX_POINT('',#43406);
#9971=VERTEX_POINT('',#43417);
#9972=VERTEX_POINT('',#43421);
#9973=VERTEX_POINT('',#43432);
#9974=VERTEX_POINT('',#43436);
#9975=VERTEX_POINT('',#43447);
#9976=VERTEX_POINT('',#43451);
#9977=VERTEX_POINT('',#43462);
#9978=VERTEX_POINT('',#43466);
#9979=VERTEX_POINT('',#43477);
#9980=VERTEX_POINT('',#43481);
#9981=VERTEX_POINT('',#43492);
#9982=VERTEX_POINT('',#43496);
#9983=VERTEX_POINT('',#43502);
#9984=VERTEX_POINT('',#43504);
#9985=VERTEX_POINT('',#43513);
#9986=VERTEX_POINT('',#43517);
#9987=VERTEX_POINT('',#43528);
#9988=VERTEX_POINT('',#43532);
#9989=VERTEX_POINT('',#43543);
#9990=VERTEX_POINT('',#43547);
#9991=VERTEX_POINT('',#43558);
#9992=VERTEX_POINT('',#43562);
#9993=VERTEX_POINT('',#43573);
#9994=VERTEX_POINT('',#43577);
#9995=VERTEX_POINT('',#43588);
#9996=VERTEX_POINT('',#43592);
#9997=VERTEX_POINT('',#43603);
#9998=VERTEX_POINT('',#43607);
#9999=VERTEX_POINT('',#43618);
#10000=VERTEX_POINT('',#43622);
#10001=VERTEX_POINT('',#43633);
#10002=VERTEX_POINT('',#43637);
#10003=VERTEX_POINT('',#43648);
#10004=VERTEX_POINT('',#43652);
#10005=VERTEX_POINT('',#43663);
#10006=VERTEX_POINT('',#43667);
#10007=VERTEX_POINT('',#43678);
#10008=VERTEX_POINT('',#43682);
#10009=VERTEX_POINT('',#43693);
#10010=VERTEX_POINT('',#43697);
#10011=VERTEX_POINT('',#43708);
#10012=VERTEX_POINT('',#43712);
#10013=VERTEX_POINT('',#43723);
#10014=VERTEX_POINT('',#43727);
#10015=VERTEX_POINT('',#43742);
#10016=VERTEX_POINT('',#43743);
#10017=VERTEX_POINT('',#43747);
#10018=VERTEX_POINT('',#43749);
#10019=VERTEX_POINT('',#43760);
#10020=VERTEX_POINT('',#43764);
#10021=VERTEX_POINT('',#43775);
#10022=VERTEX_POINT('',#43779);
#10023=VERTEX_POINT('',#43790);
#10024=VERTEX_POINT('',#43794);
#10025=VERTEX_POINT('',#43805);
#10026=VERTEX_POINT('',#43809);
#10027=VERTEX_POINT('',#43820);
#10028=VERTEX_POINT('',#43824);
#10029=VERTEX_POINT('',#43835);
#10030=VERTEX_POINT('',#43839);
#10031=VERTEX_POINT('',#43862);
#10032=VERTEX_POINT('',#43863);
#10033=VERTEX_POINT('',#43867);
#10034=VERTEX_POINT('',#43869);
#10035=VERTEX_POINT('',#43880);
#10036=VERTEX_POINT('',#43884);
#10037=VERTEX_POINT('',#43895);
#10038=VERTEX_POINT('',#43899);
#10039=VERTEX_POINT('',#43910);
#10040=VERTEX_POINT('',#43914);
#10041=VERTEX_POINT('',#43925);
#10042=VERTEX_POINT('',#43929);
#10043=VERTEX_POINT('',#43940);
#10044=VERTEX_POINT('',#43944);
#10045=VERTEX_POINT('',#43955);
#10046=VERTEX_POINT('',#43959);
#10047=VERTEX_POINT('',#43970);
#10048=VERTEX_POINT('',#43974);
#10049=VERTEX_POINT('',#43985);
#10050=VERTEX_POINT('',#43989);
#10051=VERTEX_POINT('',#44000);
#10052=VERTEX_POINT('',#44004);
#10053=VERTEX_POINT('',#44015);
#10054=VERTEX_POINT('',#44019);
#10055=VERTEX_POINT('',#44043);
#10056=VERTEX_POINT('',#44044);
#10057=VERTEX_POINT('',#44048);
#10058=VERTEX_POINT('',#44050);
#10059=VERTEX_POINT('',#44061);
#10060=VERTEX_POINT('',#44065);
#10061=VERTEX_POINT('',#44071);
#10062=VERTEX_POINT('',#44073);
#10063=VERTEX_POINT('',#44082);
#10064=VERTEX_POINT('',#44086);
#10065=VERTEX_POINT('',#44097);
#10066=VERTEX_POINT('',#44101);
#10067=VERTEX_POINT('',#44107);
#10068=VERTEX_POINT('',#44109);
#10069=VERTEX_POINT('',#44113);
#10070=VERTEX_POINT('',#44115);
#10071=VERTEX_POINT('',#44119);
#10072=VERTEX_POINT('',#44121);
#10073=VERTEX_POINT('',#44129);
#10074=VERTEX_POINT('',#44130);
#10075=VERTEX_POINT('',#44132);
#10076=VERTEX_POINT('',#44134);
#10077=VERTEX_POINT('',#44138);
#10078=VERTEX_POINT('',#44140);
#10079=VERTEX_POINT('',#44144);
#10080=VERTEX_POINT('',#44146);
#10081=VERTEX_POINT('',#44150);
#10082=VERTEX_POINT('',#44152);
#10083=VERTEX_POINT('',#44156);
#10084=VERTEX_POINT('',#44158);
#10085=VERTEX_POINT('',#44162);
#10086=VERTEX_POINT('',#44164);
#10087=VERTEX_POINT('',#44168);
#10088=VERTEX_POINT('',#44170);
#10089=VERTEX_POINT('',#44174);
#10090=VERTEX_POINT('',#44176);
#10091=VERTEX_POINT('',#44185);
#10092=VERTEX_POINT('',#44189);
#10093=VERTEX_POINT('',#44200);
#10094=VERTEX_POINT('',#44204);
#10095=VERTEX_POINT('',#44210);
#10096=VERTEX_POINT('',#44212);
#10097=VERTEX_POINT('',#44216);
#10098=VERTEX_POINT('',#44218);
#10099=VERTEX_POINT('',#44222);
#10100=VERTEX_POINT('',#44224);
#10101=VERTEX_POINT('',#44228);
#10102=VERTEX_POINT('',#44230);
#10103=VERTEX_POINT('',#44243);
#10104=VERTEX_POINT('',#44244);
#10105=VERTEX_POINT('',#44248);
#10106=VERTEX_POINT('',#44250);
#10107=VERTEX_POINT('',#44261);
#10108=VERTEX_POINT('',#44265);
#10109=VERTEX_POINT('',#44276);
#10110=VERTEX_POINT('',#44280);
#10111=VERTEX_POINT('',#44291);
#10112=VERTEX_POINT('',#44295);
#10113=VERTEX_POINT('',#44306);
#10114=VERTEX_POINT('',#44310);
#10115=VERTEX_POINT('',#44321);
#10116=VERTEX_POINT('',#44325);
#10117=VERTEX_POINT('',#44336);
#10118=VERTEX_POINT('',#44340);
#10119=VERTEX_POINT('',#44351);
#10120=VERTEX_POINT('',#44355);
#10121=VERTEX_POINT('',#44366);
#10122=VERTEX_POINT('',#44370);
#10123=VERTEX_POINT('',#44381);
#10124=VERTEX_POINT('',#44385);
#10125=VERTEX_POINT('',#44396);
#10126=VERTEX_POINT('',#44400);
#10127=VERTEX_POINT('',#44406);
#10128=VERTEX_POINT('',#44408);
#10129=VERTEX_POINT('',#44417);
#10130=VERTEX_POINT('',#44421);
#10131=VERTEX_POINT('',#44432);
#10132=VERTEX_POINT('',#44436);
#10133=VERTEX_POINT('',#44447);
#10134=VERTEX_POINT('',#44451);
#10135=VERTEX_POINT('',#44462);
#10136=VERTEX_POINT('',#44466);
#10137=VERTEX_POINT('',#44477);
#10138=VERTEX_POINT('',#44481);
#10139=VERTEX_POINT('',#44492);
#10140=VERTEX_POINT('',#44496);
#10141=VERTEX_POINT('',#44507);
#10142=VERTEX_POINT('',#44511);
#10143=VERTEX_POINT('',#44517);
#10144=VERTEX_POINT('',#44519);
#10145=VERTEX_POINT('',#44528);
#10146=VERTEX_POINT('',#44532);
#10147=VERTEX_POINT('',#44543);
#10148=VERTEX_POINT('',#44547);
#10149=VERTEX_POINT('',#44558);
#10150=VERTEX_POINT('',#44562);
#10151=VERTEX_POINT('',#44573);
#10152=VERTEX_POINT('',#44577);
#10153=VERTEX_POINT('',#44588);
#10154=VERTEX_POINT('',#44592);
#10155=VERTEX_POINT('',#44603);
#10156=VERTEX_POINT('',#44607);
#10157=VERTEX_POINT('',#44618);
#10158=VERTEX_POINT('',#44622);
#10159=VERTEX_POINT('',#44628);
#10160=VERTEX_POINT('',#44630);
#10161=VERTEX_POINT('',#44639);
#10162=VERTEX_POINT('',#44643);
#10163=VERTEX_POINT('',#44662);
#10164=VERTEX_POINT('',#44663);
#10165=VERTEX_POINT('',#44665);
#10166=VERTEX_POINT('',#44667);
#10167=VERTEX_POINT('',#44671);
#10168=VERTEX_POINT('',#44673);
#10169=VERTEX_POINT('',#44677);
#10170=VERTEX_POINT('',#44679);
#10171=VERTEX_POINT('',#44692);
#10172=VERTEX_POINT('',#44693);
#10173=VERTEX_POINT('',#44697);
#10174=VERTEX_POINT('',#44699);
#10175=VERTEX_POINT('',#44710);
#10176=VERTEX_POINT('',#44714);
#10177=VERTEX_POINT('',#44720);
#10178=VERTEX_POINT('',#44722);
#10179=VERTEX_POINT('',#44726);
#10180=VERTEX_POINT('',#44728);
#10181=VERTEX_POINT('',#44735);
#10182=VERTEX_POINT('',#44736);
#10183=VERTEX_POINT('',#44738);
#10184=VERTEX_POINT('',#44740);
#10185=VERTEX_POINT('',#44744);
#10186=VERTEX_POINT('',#44746);
#10187=VERTEX_POINT('',#44750);
#10188=VERTEX_POINT('',#44752);
#10189=VERTEX_POINT('',#44756);
#10190=VERTEX_POINT('',#44758);
#10191=VERTEX_POINT('',#44762);
#10192=VERTEX_POINT('',#44764);
#10193=VERTEX_POINT('',#44768);
#10194=VERTEX_POINT('',#44770);
#10195=VERTEX_POINT('',#44774);
#10196=VERTEX_POINT('',#44776);
#10197=VERTEX_POINT('',#44789);
#10198=VERTEX_POINT('',#44790);
#10199=VERTEX_POINT('',#44794);
#10200=VERTEX_POINT('',#44796);
#10201=VERTEX_POINT('',#44807);
#10202=VERTEX_POINT('',#44811);
#10203=VERTEX_POINT('',#44822);
#10204=VERTEX_POINT('',#44826);
#10205=VERTEX_POINT('',#44837);
#10206=VERTEX_POINT('',#44841);
#10207=VERTEX_POINT('',#44852);
#10208=VERTEX_POINT('',#44856);
#10209=VERTEX_POINT('',#44867);
#10210=VERTEX_POINT('',#44871);
#10211=VERTEX_POINT('',#44882);
#10212=VERTEX_POINT('',#44886);
#10213=VERTEX_POINT('',#44897);
#10214=VERTEX_POINT('',#44901);
#10215=VERTEX_POINT('',#44912);
#10216=VERTEX_POINT('',#44916);
#10217=VERTEX_POINT('',#44927);
#10218=VERTEX_POINT('',#44931);
#10219=VERTEX_POINT('',#44942);
#10220=VERTEX_POINT('',#44946);
#10221=VERTEX_POINT('',#44957);
#10222=VERTEX_POINT('',#44961);
#10223=VERTEX_POINT('',#44972);
#10224=VERTEX_POINT('',#44976);
#10225=VERTEX_POINT('',#44982);
#10226=VERTEX_POINT('',#44984);
#10227=VERTEX_POINT('',#44993);
#10228=VERTEX_POINT('',#44997);
#10229=VERTEX_POINT('',#45008);
#10230=VERTEX_POINT('',#45012);
#10231=VERTEX_POINT('',#45023);
#10232=VERTEX_POINT('',#45027);
#10233=VERTEX_POINT('',#45038);
#10234=VERTEX_POINT('',#45042);
#10235=VERTEX_POINT('',#45053);
#10236=VERTEX_POINT('',#45057);
#10237=VERTEX_POINT('',#45068);
#10238=VERTEX_POINT('',#45072);
#10239=VERTEX_POINT('',#45083);
#10240=VERTEX_POINT('',#45087);
#10241=VERTEX_POINT('',#45098);
#10242=VERTEX_POINT('',#45102);
#10243=VERTEX_POINT('',#45113);
#10244=VERTEX_POINT('',#45117);
#10245=VERTEX_POINT('',#45128);
#10246=VERTEX_POINT('',#45132);
#10247=VERTEX_POINT('',#45143);
#10248=VERTEX_POINT('',#45147);
#10249=VERTEX_POINT('',#45158);
#10250=VERTEX_POINT('',#45162);
#10251=VERTEX_POINT('',#45173);
#10252=VERTEX_POINT('',#45177);
#10253=VERTEX_POINT('',#45188);
#10254=VERTEX_POINT('',#45192);
#10255=VERTEX_POINT('',#45203);
#10256=VERTEX_POINT('',#45207);
#10257=VERTEX_POINT('',#45218);
#10258=VERTEX_POINT('',#45222);
#10259=VERTEX_POINT('',#45233);
#10260=VERTEX_POINT('',#45237);
#10261=VERTEX_POINT('',#45248);
#10262=VERTEX_POINT('',#45252);
#10263=VERTEX_POINT('',#45258);
#10264=VERTEX_POINT('',#45260);
#10265=VERTEX_POINT('',#45269);
#10266=VERTEX_POINT('',#45273);
#10267=VERTEX_POINT('',#45297);
#10268=VERTEX_POINT('',#45298);
#10269=VERTEX_POINT('',#45302);
#10270=VERTEX_POINT('',#45304);
#10271=VERTEX_POINT('',#45315);
#10272=VERTEX_POINT('',#45319);
#10273=VERTEX_POINT('',#45330);
#10274=VERTEX_POINT('',#45334);
#10275=VERTEX_POINT('',#45345);
#10276=VERTEX_POINT('',#45349);
#10277=VERTEX_POINT('',#45360);
#10278=VERTEX_POINT('',#45364);
#10279=VERTEX_POINT('',#45375);
#10280=VERTEX_POINT('',#45379);
#10281=VERTEX_POINT('',#45390);
#10282=VERTEX_POINT('',#45394);
#10283=VERTEX_POINT('',#45405);
#10284=VERTEX_POINT('',#45409);
#10285=VERTEX_POINT('',#45420);
#10286=VERTEX_POINT('',#45424);
#10287=VERTEX_POINT('',#45435);
#10288=VERTEX_POINT('',#45439);
#10289=VERTEX_POINT('',#45450);
#10290=VERTEX_POINT('',#45454);
#10291=VERTEX_POINT('',#45460);
#10292=VERTEX_POINT('',#45462);
#10293=VERTEX_POINT('',#45471);
#10294=VERTEX_POINT('',#45475);
#10295=VERTEX_POINT('',#45486);
#10296=VERTEX_POINT('',#45490);
#10297=VERTEX_POINT('',#45501);
#10298=VERTEX_POINT('',#45505);
#10299=VERTEX_POINT('',#45516);
#10300=VERTEX_POINT('',#45520);
#10301=VERTEX_POINT('',#45531);
#10302=VERTEX_POINT('',#45535);
#10303=VERTEX_POINT('',#45546);
#10304=VERTEX_POINT('',#45550);
#10305=VERTEX_POINT('',#45561);
#10306=VERTEX_POINT('',#45565);
#10307=VERTEX_POINT('',#45571);
#10308=VERTEX_POINT('',#45573);
#10309=VERTEX_POINT('',#45582);
#10310=VERTEX_POINT('',#45586);
#10311=VERTEX_POINT('',#45597);
#10312=VERTEX_POINT('',#45601);
#10313=VERTEX_POINT('',#45612);
#10314=VERTEX_POINT('',#45616);
#10315=VERTEX_POINT('',#45627);
#10316=VERTEX_POINT('',#45631);
#10317=VERTEX_POINT('',#45642);
#10318=VERTEX_POINT('',#45646);
#10319=VERTEX_POINT('',#45657);
#10320=VERTEX_POINT('',#45661);
#10321=VERTEX_POINT('',#45672);
#10322=VERTEX_POINT('',#45676);
#10323=VERTEX_POINT('',#45682);
#10324=VERTEX_POINT('',#45684);
#10325=VERTEX_POINT('',#45693);
#10326=VERTEX_POINT('',#45697);
#10327=VERTEX_POINT('',#45721);
#10328=VERTEX_POINT('',#45722);
#10329=VERTEX_POINT('',#45726);
#10330=VERTEX_POINT('',#45728);
#10331=VERTEX_POINT('',#45739);
#10332=VERTEX_POINT('',#45743);
#10333=VERTEX_POINT('',#45754);
#10334=VERTEX_POINT('',#45758);
#10335=VERTEX_POINT('',#45769);
#10336=VERTEX_POINT('',#45773);
#10337=VERTEX_POINT('',#45784);
#10338=VERTEX_POINT('',#45788);
#10339=VERTEX_POINT('',#45799);
#10340=VERTEX_POINT('',#45803);
#10341=VERTEX_POINT('',#45814);
#10342=VERTEX_POINT('',#45818);
#10343=VERTEX_POINT('',#45829);
#10344=VERTEX_POINT('',#45833);
#10345=VERTEX_POINT('',#45839);
#10346=VERTEX_POINT('',#45841);
#10347=VERTEX_POINT('',#45850);
#10348=VERTEX_POINT('',#45854);
#10349=VERTEX_POINT('',#45865);
#10350=VERTEX_POINT('',#45869);
#10351=VERTEX_POINT('',#45880);
#10352=VERTEX_POINT('',#45884);
#10353=VERTEX_POINT('',#45895);
#10354=VERTEX_POINT('',#45899);
#10355=VERTEX_POINT('',#45910);
#10356=VERTEX_POINT('',#45914);
#10357=VERTEX_POINT('',#45925);
#10358=VERTEX_POINT('',#45929);
#10359=VERTEX_POINT('',#45940);
#10360=VERTEX_POINT('',#45944);
#10361=VERTEX_POINT('',#45955);
#10362=VERTEX_POINT('',#45959);
#10363=VERTEX_POINT('',#45970);
#10364=VERTEX_POINT('',#45974);
#10365=VERTEX_POINT('',#45980);
#10366=VERTEX_POINT('',#45982);
#10367=VERTEX_POINT('',#45986);
#10368=VERTEX_POINT('',#45988);
#10369=VERTEX_POINT('',#45992);
#10370=VERTEX_POINT('',#45994);
#10371=VERTEX_POINT('',#46011);
#10372=VERTEX_POINT('',#46012);
#10373=VERTEX_POINT('',#46014);
#10374=VERTEX_POINT('',#46016);
#10375=VERTEX_POINT('',#46025);
#10376=VERTEX_POINT('',#46029);
#10377=VERTEX_POINT('',#46040);
#10378=VERTEX_POINT('',#46044);
#10379=VERTEX_POINT('',#46055);
#10380=VERTEX_POINT('',#46059);
#10381=VERTEX_POINT('',#46070);
#10382=VERTEX_POINT('',#46074);
#10383=VERTEX_POINT('',#46085);
#10384=VERTEX_POINT('',#46089);
#10385=VERTEX_POINT('',#46095);
#10386=VERTEX_POINT('',#46097);
#10387=VERTEX_POINT('',#46104);
#10388=VERTEX_POINT('',#46105);
#10389=VERTEX_POINT('',#46107);
#10390=VERTEX_POINT('',#46109);
#10391=VERTEX_POINT('',#46118);
#10392=VERTEX_POINT('',#46122);
#10393=VERTEX_POINT('',#46133);
#10394=VERTEX_POINT('',#46137);
#10395=VERTEX_POINT('',#46148);
#10396=VERTEX_POINT('',#46152);
#10397=VERTEX_POINT('',#46163);
#10398=VERTEX_POINT('',#46167);
#10399=VERTEX_POINT('',#46178);
#10400=VERTEX_POINT('',#46182);
#10401=VERTEX_POINT('',#46193);
#10402=VERTEX_POINT('',#46197);
#10403=VERTEX_POINT('',#46203);
#10404=VERTEX_POINT('',#46205);
#10405=VERTEX_POINT('',#46209);
#10406=VERTEX_POINT('',#46211);
#10407=VERTEX_POINT('',#46215);
#10408=VERTEX_POINT('',#46217);
#10409=VERTEX_POINT('',#46230);
#10410=VERTEX_POINT('',#46231);
#10411=VERTEX_POINT('',#46235);
#10412=VERTEX_POINT('',#46237);
#10413=VERTEX_POINT('',#46248);
#10414=VERTEX_POINT('',#46252);
#10415=VERTEX_POINT('',#46263);
#10416=VERTEX_POINT('',#46267);
#10417=VERTEX_POINT('',#46278);
#10418=VERTEX_POINT('',#46282);
#10419=VERTEX_POINT('',#46293);
#10420=VERTEX_POINT('',#46297);
#10421=VERTEX_POINT('',#46308);
#10422=VERTEX_POINT('',#46312);
#10423=VERTEX_POINT('',#46323);
#10424=VERTEX_POINT('',#46327);
#10425=VERTEX_POINT('',#46338);
#10426=VERTEX_POINT('',#46342);
#10427=VERTEX_POINT('',#46365);
#10428=VERTEX_POINT('',#46366);
#10429=VERTEX_POINT('',#46370);
#10430=VERTEX_POINT('',#46372);
#10431=VERTEX_POINT('',#46383);
#10432=VERTEX_POINT('',#46387);
#10433=VERTEX_POINT('',#46398);
#10434=VERTEX_POINT('',#46402);
#10435=VERTEX_POINT('',#46413);
#10436=VERTEX_POINT('',#46417);
#10437=VERTEX_POINT('',#46428);
#10438=VERTEX_POINT('',#46432);
#10439=VERTEX_POINT('',#46443);
#10440=VERTEX_POINT('',#46447);
#10441=VERTEX_POINT('',#46458);
#10442=VERTEX_POINT('',#46462);
#10443=VERTEX_POINT('',#46473);
#10444=VERTEX_POINT('',#46477);
#10445=VERTEX_POINT('',#46488);
#10446=VERTEX_POINT('',#46492);
#10447=VERTEX_POINT('',#46503);
#10448=VERTEX_POINT('',#46507);
#10449=VERTEX_POINT('',#46518);
#10450=VERTEX_POINT('',#46522);
#10451=VERTEX_POINT('',#46533);
#10452=VERTEX_POINT('',#46537);
#10453=VERTEX_POINT('',#46548);
#10454=VERTEX_POINT('',#46552);
#10455=VERTEX_POINT('',#46563);
#10456=VERTEX_POINT('',#46567);
#10457=VERTEX_POINT('',#46578);
#10458=VERTEX_POINT('',#46582);
#10459=VERTEX_POINT('',#46593);
#10460=VERTEX_POINT('',#46597);
#10461=VERTEX_POINT('',#46603);
#10462=VERTEX_POINT('',#46605);
#10463=VERTEX_POINT('',#46614);
#10464=VERTEX_POINT('',#46618);
#10465=VERTEX_POINT('',#46642);
#10466=VERTEX_POINT('',#46643);
#10467=VERTEX_POINT('',#46647);
#10468=VERTEX_POINT('',#46649);
#10469=VERTEX_POINT('',#46660);
#10470=VERTEX_POINT('',#46664);
#10471=VERTEX_POINT('',#46675);
#10472=VERTEX_POINT('',#46679);
#10473=VERTEX_POINT('',#46690);
#10474=VERTEX_POINT('',#46694);
#10475=VERTEX_POINT('',#46705);
#10476=VERTEX_POINT('',#46709);
#10477=VERTEX_POINT('',#46720);
#10478=VERTEX_POINT('',#46724);
#10479=VERTEX_POINT('',#46735);
#10480=VERTEX_POINT('',#46739);
#10481=VERTEX_POINT('',#46762);
#10482=VERTEX_POINT('',#46763);
#10483=VERTEX_POINT('',#46767);
#10484=VERTEX_POINT('',#46769);
#10485=VERTEX_POINT('',#46780);
#10486=VERTEX_POINT('',#46784);
#10487=VERTEX_POINT('',#46795);
#10488=VERTEX_POINT('',#46799);
#10489=VERTEX_POINT('',#46810);
#10490=VERTEX_POINT('',#46814);
#10491=VERTEX_POINT('',#46825);
#10492=VERTEX_POINT('',#46829);
#10493=VERTEX_POINT('',#46840);
#10494=VERTEX_POINT('',#46844);
#10495=VERTEX_POINT('',#46855);
#10496=VERTEX_POINT('',#46859);
#10497=VERTEX_POINT('',#46865);
#10498=VERTEX_POINT('',#46867);
#10499=VERTEX_POINT('',#46871);
#10500=VERTEX_POINT('',#46873);
#10501=VERTEX_POINT('',#46877);
#10502=VERTEX_POINT('',#46879);
#10503=VERTEX_POINT('',#46883);
#10504=VERTEX_POINT('',#46885);
#10505=VERTEX_POINT('',#46889);
#10506=VERTEX_POINT('',#46891);
#10507=VERTEX_POINT('',#46913);
#10508=VERTEX_POINT('',#46914);
#10509=VERTEX_POINT('',#46918);
#10510=VERTEX_POINT('',#46920);
#10511=VERTEX_POINT('',#46931);
#10512=VERTEX_POINT('',#46935);
#10513=VERTEX_POINT('',#46946);
#10514=VERTEX_POINT('',#46950);
#10515=VERTEX_POINT('',#46961);
#10516=VERTEX_POINT('',#46965);
#10517=VERTEX_POINT('',#46971);
#10518=VERTEX_POINT('',#46973);
#10519=VERTEX_POINT('',#46982);
#10520=VERTEX_POINT('',#46986);
#10521=VERTEX_POINT('',#46997);
#10522=VERTEX_POINT('',#47001);
#10523=VERTEX_POINT('',#47012);
#10524=VERTEX_POINT('',#47016);
#10525=VERTEX_POINT('',#47022);
#10526=VERTEX_POINT('',#47024);
#10527=VERTEX_POINT('',#47028);
#10528=VERTEX_POINT('',#47030);
#10529=VERTEX_POINT('',#47034);
#10530=VERTEX_POINT('',#47036);
#10531=VERTEX_POINT('',#47040);
#10532=VERTEX_POINT('',#47042);
#10533=VERTEX_POINT('',#47056);
#10534=VERTEX_POINT('',#47058);
#10535=VERTEX_POINT('',#47060);
#10536=VERTEX_POINT('',#47071);
#10537=VERTEX_POINT('',#47082);
#10538=VERTEX_POINT('',#47104);
#10539=VERTEX_POINT('',#47106);
#10540=VERTEX_POINT('',#47110);
#10541=VERTEX_POINT('',#47114);
#10542=VERTEX_POINT('',#47115);
#10543=VERTEX_POINT('',#47117);
#10544=VERTEX_POINT('',#47144);
#10545=VERTEX_POINT('',#47148);
#10546=VERTEX_POINT('',#47149);
#10547=VERTEX_POINT('',#47154);
#10548=VERTEX_POINT('',#47161);
#10549=VERTEX_POINT('',#47163);
#10550=VERTEX_POINT('',#47168);
#10551=VERTEX_POINT('',#47172);
#10552=VERTEX_POINT('',#47174);
#10553=VERTEX_POINT('',#47178);
#10554=VERTEX_POINT('',#47180);
#10555=VERTEX_POINT('',#47182);
#10556=VERTEX_POINT('',#47184);
#10557=VERTEX_POINT('',#47186);
#10558=VERTEX_POINT('',#47188);
#10559=VERTEX_POINT('',#47190);
#10560=VERTEX_POINT('',#47193);
#10561=VERTEX_POINT('',#47197);
#10562=VERTEX_POINT('',#47201);
#10563=VERTEX_POINT('',#47205);
#10564=VERTEX_POINT('',#47209);
#10565=VERTEX_POINT('',#47213);
#10566=VERTEX_POINT('',#47217);
#10567=VERTEX_POINT('',#47221);
#10568=VERTEX_POINT('',#47225);
#10569=VERTEX_POINT('',#47229);
#10570=VERTEX_POINT('',#47233);
#10571=VERTEX_POINT('',#47237);
#10572=VERTEX_POINT('',#47240);
#10573=VERTEX_POINT('',#47243);
#10574=VERTEX_POINT('',#47246);
#10575=VERTEX_POINT('',#47249);
#10576=VERTEX_POINT('',#47252);
#10577=VERTEX_POINT('',#47255);
#10578=VERTEX_POINT('',#47257);
#10579=VERTEX_POINT('',#47261);
#10580=VERTEX_POINT('',#47268);
#10581=VERTEX_POINT('',#47271);
#12519=EDGE_CURVE('',#9941,#9942,#716,.T.);
#12520=EDGE_CURVE('',#9941,#9943,#6023,.T.);
#12521=EDGE_CURVE('',#9943,#9944,#717,.T.);
#12522=EDGE_CURVE('',#9942,#9944,#6024,.T.);
#12523=EDGE_CURVE('',#9945,#9941,#718,.T.);
#12524=EDGE_CURVE('',#9945,#9946,#6025,.T.);
#12525=EDGE_CURVE('',#9946,#9943,#719,.T.);
#12526=EDGE_CURVE('',#9947,#9945,#720,.T.);
#12527=EDGE_CURVE('',#9947,#9948,#6026,.T.);
#12528=EDGE_CURVE('',#9948,#9946,#721,.T.);
#12529=EDGE_CURVE('',#9949,#9947,#722,.T.);
#12530=EDGE_CURVE('',#9949,#9950,#6027,.T.);
#12531=EDGE_CURVE('',#9950,#9948,#723,.T.);
#12532=EDGE_CURVE('',#9951,#9949,#724,.T.);
#12533=EDGE_CURVE('',#9951,#9952,#6028,.T.);
#12534=EDGE_CURVE('',#9952,#9950,#725,.T.);
#12535=EDGE_CURVE('',#9953,#9951,#726,.T.);
#12536=EDGE_CURVE('',#9953,#9954,#6029,.T.);
#12537=EDGE_CURVE('',#9954,#9952,#727,.T.);
#12538=EDGE_CURVE('',#9955,#9953,#728,.T.);
#12539=EDGE_CURVE('',#9955,#9956,#6030,.T.);
#12540=EDGE_CURVE('',#9956,#9954,#729,.T.);
#12541=EDGE_CURVE('',#9957,#9955,#730,.T.);
#12542=EDGE_CURVE('',#9957,#9958,#6031,.T.);
#12543=EDGE_CURVE('',#9958,#9956,#731,.T.);
#12544=EDGE_CURVE('',#9959,#9957,#732,.T.);
#12545=EDGE_CURVE('',#9959,#9960,#6032,.T.);
#12546=EDGE_CURVE('',#9960,#9958,#733,.T.);
#12547=EDGE_CURVE('',#9942,#9959,#6033,.T.);
#12548=EDGE_CURVE('',#9944,#9960,#6034,.T.);
#12549=EDGE_CURVE('',#9961,#9962,#734,.T.);
#12550=EDGE_CURVE('',#9961,#9963,#6035,.T.);
#12551=EDGE_CURVE('',#9963,#9964,#735,.T.);
#12552=EDGE_CURVE('',#9962,#9964,#6036,.T.);
#12553=EDGE_CURVE('',#9965,#9961,#736,.T.);
#12554=EDGE_CURVE('',#9965,#9966,#6037,.T.);
#12555=EDGE_CURVE('',#9966,#9963,#737,.T.);
#12556=EDGE_CURVE('',#9967,#9965,#6038,.T.);
#12557=EDGE_CURVE('',#9967,#9968,#6039,.T.);
#12558=EDGE_CURVE('',#9968,#9966,#6040,.T.);
#12559=EDGE_CURVE('',#9969,#9967,#738,.T.);
#12560=EDGE_CURVE('',#9969,#9970,#6041,.T.);
#12561=EDGE_CURVE('',#9970,#9968,#739,.T.);
#12562=EDGE_CURVE('',#9971,#9969,#740,.T.);
#12563=EDGE_CURVE('',#9971,#9972,#6042,.T.);
#12564=EDGE_CURVE('',#9972,#9970,#741,.T.);
#12565=EDGE_CURVE('',#9973,#9971,#742,.T.);
#12566=EDGE_CURVE('',#9973,#9974,#6043,.T.);
#12567=EDGE_CURVE('',#9974,#9972,#743,.T.);
#12568=EDGE_CURVE('',#9975,#9973,#744,.T.);
#12569=EDGE_CURVE('',#9975,#9976,#6044,.T.);
#12570=EDGE_CURVE('',#9976,#9974,#745,.T.);
#12571=EDGE_CURVE('',#9977,#9975,#746,.T.);
#12572=EDGE_CURVE('',#9977,#9978,#6045,.T.);
#12573=EDGE_CURVE('',#9978,#9976,#747,.T.);
#12574=EDGE_CURVE('',#9979,#9977,#748,.T.);
#12575=EDGE_CURVE('',#9979,#9980,#6046,.T.);
#12576=EDGE_CURVE('',#9980,#9978,#749,.T.);
#12577=EDGE_CURVE('',#9981,#9979,#750,.T.);
#12578=EDGE_CURVE('',#9981,#9982,#6047,.T.);
#12579=EDGE_CURVE('',#9982,#9980,#751,.T.);
#12580=EDGE_CURVE('',#9983,#9981,#6048,.T.);
#12581=EDGE_CURVE('',#9983,#9984,#6049,.T.);
#12582=EDGE_CURVE('',#9984,#9982,#6050,.T.);
#12583=EDGE_CURVE('',#9985,#9983,#752,.T.);
#12584=EDGE_CURVE('',#9985,#9986,#6051,.T.);
#12585=EDGE_CURVE('',#9986,#9984,#753,.T.);
#12586=EDGE_CURVE('',#9987,#9985,#754,.T.);
#12587=EDGE_CURVE('',#9987,#9988,#6052,.T.);
#12588=EDGE_CURVE('',#9988,#9986,#755,.T.);
#12589=EDGE_CURVE('',#9989,#9987,#756,.T.);
#12590=EDGE_CURVE('',#9989,#9990,#6053,.T.);
#12591=EDGE_CURVE('',#9990,#9988,#757,.T.);
#12592=EDGE_CURVE('',#9991,#9989,#758,.T.);
#12593=EDGE_CURVE('',#9991,#9992,#6054,.T.);
#12594=EDGE_CURVE('',#9992,#9990,#759,.T.);
#12595=EDGE_CURVE('',#9993,#9991,#760,.T.);
#12596=EDGE_CURVE('',#9993,#9994,#6055,.T.);
#12597=EDGE_CURVE('',#9994,#9992,#761,.T.);
#12598=EDGE_CURVE('',#9995,#9993,#762,.T.);
#12599=EDGE_CURVE('',#9995,#9996,#6056,.T.);
#12600=EDGE_CURVE('',#9996,#9994,#763,.T.);
#12601=EDGE_CURVE('',#9997,#9995,#764,.T.);
#12602=EDGE_CURVE('',#9997,#9998,#6057,.T.);
#12603=EDGE_CURVE('',#9998,#9996,#765,.T.);
#12604=EDGE_CURVE('',#9999,#9997,#766,.T.);
#12605=EDGE_CURVE('',#9999,#10000,#6058,.T.);
#12606=EDGE_CURVE('',#10000,#9998,#767,.T.);
#12607=EDGE_CURVE('',#10001,#9999,#768,.T.);
#12608=EDGE_CURVE('',#10001,#10002,#6059,.T.);
#12609=EDGE_CURVE('',#10002,#10000,#769,.T.);
#12610=EDGE_CURVE('',#10003,#10001,#770,.T.);
#12611=EDGE_CURVE('',#10003,#10004,#6060,.T.);
#12612=EDGE_CURVE('',#10004,#10002,#771,.T.);
#12613=EDGE_CURVE('',#10005,#10003,#772,.T.);
#12614=EDGE_CURVE('',#10005,#10006,#6061,.T.);
#12615=EDGE_CURVE('',#10006,#10004,#773,.T.);
#12616=EDGE_CURVE('',#10007,#10005,#774,.T.);
#12617=EDGE_CURVE('',#10007,#10008,#6062,.T.);
#12618=EDGE_CURVE('',#10008,#10006,#775,.T.);
#12619=EDGE_CURVE('',#10009,#10007,#776,.T.);
#12620=EDGE_CURVE('',#10009,#10010,#6063,.T.);
#12621=EDGE_CURVE('',#10010,#10008,#777,.T.);
#12622=EDGE_CURVE('',#10011,#10009,#778,.T.);
#12623=EDGE_CURVE('',#10011,#10012,#6064,.T.);
#12624=EDGE_CURVE('',#10012,#10010,#779,.T.);
#12625=EDGE_CURVE('',#10013,#10011,#780,.T.);
#12626=EDGE_CURVE('',#10013,#10014,#6065,.T.);
#12627=EDGE_CURVE('',#10014,#10012,#781,.T.);
#12628=EDGE_CURVE('',#9962,#10013,#6066,.T.);
#12629=EDGE_CURVE('',#9964,#10014,#6067,.T.);
#12630=EDGE_CURVE('',#10015,#10016,#782,.T.);
#12631=EDGE_CURVE('',#10015,#10017,#6068,.T.);
#12632=EDGE_CURVE('',#10017,#10018,#783,.T.);
#12633=EDGE_CURVE('',#10016,#10018,#6069,.T.);
#12634=EDGE_CURVE('',#10019,#10015,#784,.T.);
#12635=EDGE_CURVE('',#10019,#10020,#6070,.T.);
#12636=EDGE_CURVE('',#10020,#10017,#785,.T.);
#12637=EDGE_CURVE('',#10021,#10019,#786,.T.);
#12638=EDGE_CURVE('',#10021,#10022,#6071,.T.);
#12639=EDGE_CURVE('',#10022,#10020,#787,.T.);
#12640=EDGE_CURVE('',#10023,#10021,#788,.T.);
#12641=EDGE_CURVE('',#10023,#10024,#6072,.T.);
#12642=EDGE_CURVE('',#10024,#10022,#789,.T.);
#12643=EDGE_CURVE('',#10025,#10023,#790,.T.);
#12644=EDGE_CURVE('',#10025,#10026,#6073,.T.);
#12645=EDGE_CURVE('',#10026,#10024,#791,.T.);
#12646=EDGE_CURVE('',#10027,#10025,#792,.T.);
#12647=EDGE_CURVE('',#10027,#10028,#6074,.T.);
#12648=EDGE_CURVE('',#10028,#10026,#793,.T.);
#12649=EDGE_CURVE('',#10029,#10027,#794,.T.);
#12650=EDGE_CURVE('',#10029,#10030,#6075,.T.);
#12651=EDGE_CURVE('',#10030,#10028,#795,.T.);
#12652=EDGE_CURVE('',#10016,#10029,#796,.T.);
#12653=EDGE_CURVE('',#10018,#10030,#797,.T.);
#12654=EDGE_CURVE('',#10031,#10032,#798,.T.);
#12655=EDGE_CURVE('',#10031,#10033,#6076,.T.);
#12656=EDGE_CURVE('',#10033,#10034,#799,.T.);
#12657=EDGE_CURVE('',#10032,#10034,#6077,.T.);
#12658=EDGE_CURVE('',#10035,#10031,#800,.T.);
#12659=EDGE_CURVE('',#10035,#10036,#6078,.T.);
#12660=EDGE_CURVE('',#10036,#10033,#801,.T.);
#12661=EDGE_CURVE('',#10037,#10035,#802,.T.);
#12662=EDGE_CURVE('',#10037,#10038,#6079,.T.);
#12663=EDGE_CURVE('',#10038,#10036,#803,.T.);
#12664=EDGE_CURVE('',#10039,#10037,#804,.T.);
#12665=EDGE_CURVE('',#10039,#10040,#6080,.T.);
#12666=EDGE_CURVE('',#10040,#10038,#805,.T.);
#12667=EDGE_CURVE('',#10041,#10039,#806,.T.);
#12668=EDGE_CURVE('',#10041,#10042,#6081,.T.);
#12669=EDGE_CURVE('',#10042,#10040,#807,.T.);
#12670=EDGE_CURVE('',#10043,#10041,#808,.T.);
#12671=EDGE_CURVE('',#10043,#10044,#6082,.T.);
#12672=EDGE_CURVE('',#10044,#10042,#809,.T.);
#12673=EDGE_CURVE('',#10045,#10043,#810,.T.);
#12674=EDGE_CURVE('',#10045,#10046,#6083,.T.);
#12675=EDGE_CURVE('',#10046,#10044,#811,.T.);
#12676=EDGE_CURVE('',#10047,#10045,#812,.T.);
#12677=EDGE_CURVE('',#10047,#10048,#6084,.T.);
#12678=EDGE_CURVE('',#10048,#10046,#813,.T.);
#12679=EDGE_CURVE('',#10049,#10047,#814,.T.);
#12680=EDGE_CURVE('',#10049,#10050,#6085,.T.);
#12681=EDGE_CURVE('',#10050,#10048,#815,.T.);
#12682=EDGE_CURVE('',#10051,#10049,#816,.T.);
#12683=EDGE_CURVE('',#10051,#10052,#6086,.T.);
#12684=EDGE_CURVE('',#10052,#10050,#817,.T.);
#12685=EDGE_CURVE('',#10053,#10051,#818,.T.);
#12686=EDGE_CURVE('',#10053,#10054,#6087,.T.);
#12687=EDGE_CURVE('',#10054,#10052,#819,.T.);
#12688=EDGE_CURVE('',#10032,#10053,#820,.T.);
#12689=EDGE_CURVE('',#10034,#10054,#821,.T.);
#12690=EDGE_CURVE('',#10055,#10056,#822,.T.);
#12691=EDGE_CURVE('',#10055,#10057,#6088,.T.);
#12692=EDGE_CURVE('',#10057,#10058,#823,.T.);
#12693=EDGE_CURVE('',#10056,#10058,#6089,.T.);
#12694=EDGE_CURVE('',#10059,#10055,#824,.T.);
#12695=EDGE_CURVE('',#10059,#10060,#6090,.T.);
#12696=EDGE_CURVE('',#10060,#10057,#825,.T.);
#12697=EDGE_CURVE('',#10061,#10059,#6091,.T.);
#12698=EDGE_CURVE('',#10061,#10062,#6092,.T.);
#12699=EDGE_CURVE('',#10062,#10060,#6093,.T.);
#12700=EDGE_CURVE('',#10063,#10061,#826,.T.);
#12701=EDGE_CURVE('',#10063,#10064,#6094,.T.);
#12702=EDGE_CURVE('',#10064,#10062,#827,.T.);
#12703=EDGE_CURVE('',#10065,#10063,#828,.T.);
#12704=EDGE_CURVE('',#10065,#10066,#6095,.T.);
#12705=EDGE_CURVE('',#10066,#10064,#829,.T.);
#12706=EDGE_CURVE('',#10067,#10065,#6096,.T.);
#12707=EDGE_CURVE('',#10067,#10068,#6097,.T.);
#12708=EDGE_CURVE('',#10068,#10066,#6098,.T.);
#12709=EDGE_CURVE('',#10069,#10067,#6099,.T.);
#12710=EDGE_CURVE('',#10069,#10070,#6100,.T.);
#12711=EDGE_CURVE('',#10070,#10068,#6101,.T.);
#12712=EDGE_CURVE('',#10071,#10069,#6102,.T.);
#12713=EDGE_CURVE('',#10071,#10072,#6103,.T.);
#12714=EDGE_CURVE('',#10072,#10070,#6104,.T.);
#12715=EDGE_CURVE('',#10056,#10071,#6105,.T.);
#12716=EDGE_CURVE('',#10058,#10072,#6106,.T.);
#12717=EDGE_CURVE('',#10073,#10074,#6107,.T.);
#12718=EDGE_CURVE('',#10073,#10075,#6108,.T.);
#12719=EDGE_CURVE('',#10075,#10076,#6109,.T.);
#12720=EDGE_CURVE('',#10074,#10076,#6110,.T.);
#12721=EDGE_CURVE('',#10077,#10073,#6111,.T.);
#12722=EDGE_CURVE('',#10077,#10078,#6112,.T.);
#12723=EDGE_CURVE('',#10078,#10075,#6113,.T.);
#12724=EDGE_CURVE('',#10079,#10077,#6114,.T.);
#12725=EDGE_CURVE('',#10079,#10080,#6115,.T.);
#12726=EDGE_CURVE('',#10080,#10078,#6116,.T.);
#12727=EDGE_CURVE('',#10081,#10079,#6117,.T.);
#12728=EDGE_CURVE('',#10081,#10082,#6118,.T.);
#12729=EDGE_CURVE('',#10082,#10080,#6119,.T.);
#12730=EDGE_CURVE('',#10083,#10081,#6120,.T.);
#12731=EDGE_CURVE('',#10083,#10084,#6121,.T.);
#12732=EDGE_CURVE('',#10084,#10082,#6122,.T.);
#12733=EDGE_CURVE('',#10085,#10083,#6123,.T.);
#12734=EDGE_CURVE('',#10085,#10086,#6124,.T.);
#12735=EDGE_CURVE('',#10086,#10084,#6125,.T.);
#12736=EDGE_CURVE('',#10087,#10085,#6126,.T.);
#12737=EDGE_CURVE('',#10087,#10088,#6127,.T.);
#12738=EDGE_CURVE('',#10088,#10086,#6128,.T.);
#12739=EDGE_CURVE('',#10089,#10087,#6129,.T.);
#12740=EDGE_CURVE('',#10089,#10090,#6130,.T.);
#12741=EDGE_CURVE('',#10090,#10088,#6131,.T.);
#12742=EDGE_CURVE('',#10091,#10089,#830,.T.);
#12743=EDGE_CURVE('',#10091,#10092,#6132,.T.);
#12744=EDGE_CURVE('',#10092,#10090,#831,.T.);
#12745=EDGE_CURVE('',#10093,#10091,#832,.T.);
#12746=EDGE_CURVE('',#10093,#10094,#6133,.T.);
#12747=EDGE_CURVE('',#10094,#10092,#833,.T.);
#12748=EDGE_CURVE('',#10095,#10093,#6134,.T.);
#12749=EDGE_CURVE('',#10095,#10096,#6135,.T.);
#12750=EDGE_CURVE('',#10096,#10094,#6136,.T.);
#12751=EDGE_CURVE('',#10097,#10095,#6137,.T.);
#12752=EDGE_CURVE('',#10097,#10098,#6138,.T.);
#12753=EDGE_CURVE('',#10098,#10096,#6139,.T.);
#12754=EDGE_CURVE('',#10099,#10097,#6140,.T.);
#12755=EDGE_CURVE('',#10099,#10100,#6141,.T.);
#12756=EDGE_CURVE('',#10100,#10098,#6142,.T.);
#12757=EDGE_CURVE('',#10101,#10099,#6143,.T.);
#12758=EDGE_CURVE('',#10101,#10102,#6144,.T.);
#12759=EDGE_CURVE('',#10102,#10100,#6145,.T.);
#12760=EDGE_CURVE('',#10074,#10101,#6146,.T.);
#12761=EDGE_CURVE('',#10076,#10102,#6147,.T.);
#12762=EDGE_CURVE('',#10103,#10104,#834,.T.);
#12763=EDGE_CURVE('',#10103,#10105,#6148,.T.);
#12764=EDGE_CURVE('',#10105,#10106,#835,.T.);
#12765=EDGE_CURVE('',#10104,#10106,#6149,.T.);
#12766=EDGE_CURVE('',#10107,#10103,#836,.T.);
#12767=EDGE_CURVE('',#10107,#10108,#6150,.T.);
#12768=EDGE_CURVE('',#10108,#10105,#837,.T.);
#12769=EDGE_CURVE('',#10109,#10107,#838,.T.);
#12770=EDGE_CURVE('',#10109,#10110,#6151,.T.);
#12771=EDGE_CURVE('',#10110,#10108,#839,.T.);
#12772=EDGE_CURVE('',#10111,#10109,#840,.T.);
#12773=EDGE_CURVE('',#10111,#10112,#6152,.T.);
#12774=EDGE_CURVE('',#10112,#10110,#841,.T.);
#12775=EDGE_CURVE('',#10113,#10111,#842,.T.);
#12776=EDGE_CURVE('',#10113,#10114,#6153,.T.);
#12777=EDGE_CURVE('',#10114,#10112,#843,.T.);
#12778=EDGE_CURVE('',#10115,#10113,#844,.T.);
#12779=EDGE_CURVE('',#10115,#10116,#6154,.T.);
#12780=EDGE_CURVE('',#10116,#10114,#845,.T.);
#12781=EDGE_CURVE('',#10117,#10115,#846,.T.);
#12782=EDGE_CURVE('',#10117,#10118,#6155,.T.);
#12783=EDGE_CURVE('',#10118,#10116,#847,.T.);
#12784=EDGE_CURVE('',#10119,#10117,#848,.T.);
#12785=EDGE_CURVE('',#10119,#10120,#6156,.T.);
#12786=EDGE_CURVE('',#10120,#10118,#849,.T.);
#12787=EDGE_CURVE('',#10121,#10119,#850,.T.);
#12788=EDGE_CURVE('',#10121,#10122,#6157,.T.);
#12789=EDGE_CURVE('',#10122,#10120,#851,.T.);
#12790=EDGE_CURVE('',#10123,#10121,#852,.T.);
#12791=EDGE_CURVE('',#10123,#10124,#6158,.T.);
#12792=EDGE_CURVE('',#10124,#10122,#853,.T.);
#12793=EDGE_CURVE('',#10125,#10123,#854,.T.);
#12794=EDGE_CURVE('',#10125,#10126,#6159,.T.);
#12795=EDGE_CURVE('',#10126,#10124,#855,.T.);
#12796=EDGE_CURVE('',#10127,#10125,#6160,.T.);
#12797=EDGE_CURVE('',#10127,#10128,#6161,.T.);
#12798=EDGE_CURVE('',#10128,#10126,#6162,.T.);
#12799=EDGE_CURVE('',#10129,#10127,#856,.T.);
#12800=EDGE_CURVE('',#10129,#10130,#6163,.T.);
#12801=EDGE_CURVE('',#10130,#10128,#857,.T.);
#12802=EDGE_CURVE('',#10131,#10129,#858,.T.);
#12803=EDGE_CURVE('',#10131,#10132,#6164,.T.);
#12804=EDGE_CURVE('',#10132,#10130,#859,.T.);
#12805=EDGE_CURVE('',#10133,#10131,#860,.T.);
#12806=EDGE_CURVE('',#10133,#10134,#6165,.T.);
#12807=EDGE_CURVE('',#10134,#10132,#861,.T.);
#12808=EDGE_CURVE('',#10135,#10133,#862,.T.);
#12809=EDGE_CURVE('',#10135,#10136,#6166,.T.);
#12810=EDGE_CURVE('',#10136,#10134,#863,.T.);
#12811=EDGE_CURVE('',#10137,#10135,#864,.T.);
#12812=EDGE_CURVE('',#10137,#10138,#6167,.T.);
#12813=EDGE_CURVE('',#10138,#10136,#865,.T.);
#12814=EDGE_CURVE('',#10139,#10137,#866,.T.);
#12815=EDGE_CURVE('',#10139,#10140,#6168,.T.);
#12816=EDGE_CURVE('',#10140,#10138,#867,.T.);
#12817=EDGE_CURVE('',#10141,#10139,#868,.T.);
#12818=EDGE_CURVE('',#10141,#10142,#6169,.T.);
#12819=EDGE_CURVE('',#10142,#10140,#869,.T.);
#12820=EDGE_CURVE('',#10143,#10141,#6170,.T.);
#12821=EDGE_CURVE('',#10143,#10144,#6171,.T.);
#12822=EDGE_CURVE('',#10144,#10142,#6172,.T.);
#12823=EDGE_CURVE('',#10145,#10143,#870,.T.);
#12824=EDGE_CURVE('',#10145,#10146,#6173,.T.);
#12825=EDGE_CURVE('',#10146,#10144,#871,.T.);
#12826=EDGE_CURVE('',#10147,#10145,#872,.T.);
#12827=EDGE_CURVE('',#10147,#10148,#6174,.T.);
#12828=EDGE_CURVE('',#10148,#10146,#873,.T.);
#12829=EDGE_CURVE('',#10149,#10147,#874,.T.);
#12830=EDGE_CURVE('',#10149,#10150,#6175,.T.);
#12831=EDGE_CURVE('',#10150,#10148,#875,.T.);
#12832=EDGE_CURVE('',#10151,#10149,#876,.T.);
#12833=EDGE_CURVE('',#10151,#10152,#6176,.T.);
#12834=EDGE_CURVE('',#10152,#10150,#877,.T.);
#12835=EDGE_CURVE('',#10153,#10151,#878,.T.);
#12836=EDGE_CURVE('',#10153,#10154,#6177,.T.);
#12837=EDGE_CURVE('',#10154,#10152,#879,.T.);
#12838=EDGE_CURVE('',#10155,#10153,#880,.T.);
#12839=EDGE_CURVE('',#10155,#10156,#6178,.T.);
#12840=EDGE_CURVE('',#10156,#10154,#881,.T.);
#12841=EDGE_CURVE('',#10157,#10155,#882,.T.);
#12842=EDGE_CURVE('',#10157,#10158,#6179,.T.);
#12843=EDGE_CURVE('',#10158,#10156,#883,.T.);
#12844=EDGE_CURVE('',#10159,#10157,#6180,.T.);
#12845=EDGE_CURVE('',#10159,#10160,#6181,.T.);
#12846=EDGE_CURVE('',#10160,#10158,#6182,.T.);
#12847=EDGE_CURVE('',#10161,#10159,#884,.T.);
#12848=EDGE_CURVE('',#10161,#10162,#6183,.T.);
#12849=EDGE_CURVE('',#10162,#10160,#885,.T.);
#12850=EDGE_CURVE('',#10104,#10161,#886,.T.);
#12851=EDGE_CURVE('',#10106,#10162,#887,.T.);
#12852=EDGE_CURVE('',#10163,#10164,#6184,.T.);
#12853=EDGE_CURVE('',#10163,#10165,#6185,.T.);
#12854=EDGE_CURVE('',#10165,#10166,#6186,.T.);
#12855=EDGE_CURVE('',#10164,#10166,#6187,.T.);
#12856=EDGE_CURVE('',#10167,#10163,#6188,.T.);
#12857=EDGE_CURVE('',#10167,#10168,#6189,.T.);
#12858=EDGE_CURVE('',#10168,#10165,#6190,.T.);
#12859=EDGE_CURVE('',#10169,#10167,#6191,.T.);
#12860=EDGE_CURVE('',#10169,#10170,#6192,.T.);
#12861=EDGE_CURVE('',#10170,#10168,#6193,.T.);
#12862=EDGE_CURVE('',#10164,#10169,#6194,.T.);
#12863=EDGE_CURVE('',#10166,#10170,#6195,.T.);
#12864=EDGE_CURVE('',#10171,#10172,#888,.T.);
#12865=EDGE_CURVE('',#10171,#10173,#6196,.T.);
#12866=EDGE_CURVE('',#10173,#10174,#889,.T.);
#12867=EDGE_CURVE('',#10172,#10174,#6197,.T.);
#12868=EDGE_CURVE('',#10175,#10171,#890,.T.);
#12869=EDGE_CURVE('',#10175,#10176,#6198,.T.);
#12870=EDGE_CURVE('',#10176,#10173,#891,.T.);
#12871=EDGE_CURVE('',#10177,#10175,#6199,.T.);
#12872=EDGE_CURVE('',#10177,#10178,#6200,.T.);
#12873=EDGE_CURVE('',#10178,#10176,#6201,.T.);
#12874=EDGE_CURVE('',#10179,#10177,#6202,.T.);
#12875=EDGE_CURVE('',#10179,#10180,#6203,.T.);
#12876=EDGE_CURVE('',#10180,#10178,#6204,.T.);
#12877=EDGE_CURVE('',#10172,#10179,#6205,.T.);
#12878=EDGE_CURVE('',#10174,#10180,#6206,.T.);
#12879=EDGE_CURVE('',#10181,#10182,#6207,.T.);
#12880=EDGE_CURVE('',#10181,#10183,#6208,.T.);
#12881=EDGE_CURVE('',#10183,#10184,#6209,.T.);
#12882=EDGE_CURVE('',#10182,#10184,#6210,.T.);
#12883=EDGE_CURVE('',#10185,#10181,#6211,.T.);
#12884=EDGE_CURVE('',#10185,#10186,#6212,.T.);
#12885=EDGE_CURVE('',#10186,#10183,#6213,.T.);
#12886=EDGE_CURVE('',#10187,#10185,#6214,.T.);
#12887=EDGE_CURVE('',#10187,#10188,#6215,.T.);
#12888=EDGE_CURVE('',#10188,#10186,#6216,.T.);
#12889=EDGE_CURVE('',#10189,#10187,#6217,.T.);
#12890=EDGE_CURVE('',#10189,#10190,#6218,.T.);
#12891=EDGE_CURVE('',#10190,#10188,#6219,.T.);
#12892=EDGE_CURVE('',#10191,#10189,#6220,.T.);
#12893=EDGE_CURVE('',#10191,#10192,#6221,.T.);
#12894=EDGE_CURVE('',#10192,#10190,#6222,.T.);
#12895=EDGE_CURVE('',#10193,#10191,#6223,.T.);
#12896=EDGE_CURVE('',#10193,#10194,#6224,.T.);
#12897=EDGE_CURVE('',#10194,#10192,#6225,.T.);
#12898=EDGE_CURVE('',#10195,#10193,#6226,.T.);
#12899=EDGE_CURVE('',#10195,#10196,#6227,.T.);
#12900=EDGE_CURVE('',#10196,#10194,#6228,.T.);
#12901=EDGE_CURVE('',#10182,#10195,#6229,.T.);
#12902=EDGE_CURVE('',#10184,#10196,#6230,.T.);
#12903=EDGE_CURVE('',#10197,#10198,#892,.T.);
#12904=EDGE_CURVE('',#10197,#10199,#6231,.T.);
#12905=EDGE_CURVE('',#10199,#10200,#893,.T.);
#12906=EDGE_CURVE('',#10198,#10200,#6232,.T.);
#12907=EDGE_CURVE('',#10201,#10197,#894,.T.);
#12908=EDGE_CURVE('',#10201,#10202,#6233,.T.);
#12909=EDGE_CURVE('',#10202,#10199,#895,.T.);
#12910=EDGE_CURVE('',#10203,#10201,#896,.T.);
#12911=EDGE_CURVE('',#10203,#10204,#6234,.T.);
#12912=EDGE_CURVE('',#10204,#10202,#897,.T.);
#12913=EDGE_CURVE('',#10205,#10203,#898,.T.);
#12914=EDGE_CURVE('',#10205,#10206,#6235,.T.);
#12915=EDGE_CURVE('',#10206,#10204,#899,.T.);
#12916=EDGE_CURVE('',#10207,#10205,#900,.T.);
#12917=EDGE_CURVE('',#10207,#10208,#6236,.T.);
#12918=EDGE_CURVE('',#10208,#10206,#901,.T.);
#12919=EDGE_CURVE('',#10209,#10207,#902,.T.);
#12920=EDGE_CURVE('',#10209,#10210,#6237,.T.);
#12921=EDGE_CURVE('',#10210,#10208,#903,.T.);
#12922=EDGE_CURVE('',#10211,#10209,#904,.T.);
#12923=EDGE_CURVE('',#10211,#10212,#6238,.T.);
#12924=EDGE_CURVE('',#10212,#10210,#905,.T.);
#12925=EDGE_CURVE('',#10213,#10211,#906,.T.);
#12926=EDGE_CURVE('',#10213,#10214,#6239,.T.);
#12927=EDGE_CURVE('',#10214,#10212,#907,.T.);
#12928=EDGE_CURVE('',#10215,#10213,#908,.T.);
#12929=EDGE_CURVE('',#10215,#10216,#6240,.T.);
#12930=EDGE_CURVE('',#10216,#10214,#909,.T.);
#12931=EDGE_CURVE('',#10217,#10215,#910,.T.);
#12932=EDGE_CURVE('',#10217,#10218,#6241,.T.);
#12933=EDGE_CURVE('',#10218,#10216,#911,.T.);
#12934=EDGE_CURVE('',#10219,#10217,#912,.T.);
#12935=EDGE_CURVE('',#10219,#10220,#6242,.T.);
#12936=EDGE_CURVE('',#10220,#10218,#913,.T.);
#12937=EDGE_CURVE('',#10221,#10219,#914,.T.);
#12938=EDGE_CURVE('',#10221,#10222,#6243,.T.);
#12939=EDGE_CURVE('',#10222,#10220,#915,.T.);
#12940=EDGE_CURVE('',#10223,#10221,#916,.T.);
#12941=EDGE_CURVE('',#10223,#10224,#6244,.T.);
#12942=EDGE_CURVE('',#10224,#10222,#917,.T.);
#12943=EDGE_CURVE('',#10225,#10223,#6245,.T.);
#12944=EDGE_CURVE('',#10225,#10226,#6246,.T.);
#12945=EDGE_CURVE('',#10226,#10224,#6247,.T.);
#12946=EDGE_CURVE('',#10227,#10225,#918,.T.);
#12947=EDGE_CURVE('',#10227,#10228,#6248,.T.);
#12948=EDGE_CURVE('',#10228,#10226,#919,.T.);
#12949=EDGE_CURVE('',#10229,#10227,#920,.T.);
#12950=EDGE_CURVE('',#10229,#10230,#6249,.T.);
#12951=EDGE_CURVE('',#10230,#10228,#921,.T.);
#12952=EDGE_CURVE('',#10231,#10229,#922,.T.);
#12953=EDGE_CURVE('',#10231,#10232,#6250,.T.);
#12954=EDGE_CURVE('',#10232,#10230,#923,.T.);
#12955=EDGE_CURVE('',#10233,#10231,#924,.T.);
#12956=EDGE_CURVE('',#10233,#10234,#6251,.T.);
#12957=EDGE_CURVE('',#10234,#10232,#925,.T.);
#12958=EDGE_CURVE('',#10235,#10233,#926,.T.);
#12959=EDGE_CURVE('',#10235,#10236,#6252,.T.);
#12960=EDGE_CURVE('',#10236,#10234,#927,.T.);
#12961=EDGE_CURVE('',#10237,#10235,#928,.T.);
#12962=EDGE_CURVE('',#10237,#10238,#6253,.T.);
#12963=EDGE_CURVE('',#10238,#10236,#929,.T.);
#12964=EDGE_CURVE('',#10239,#10237,#930,.T.);
#12965=EDGE_CURVE('',#10239,#10240,#6254,.T.);
#12966=EDGE_CURVE('',#10240,#10238,#931,.T.);
#12967=EDGE_CURVE('',#10241,#10239,#932,.T.);
#12968=EDGE_CURVE('',#10241,#10242,#6255,.T.);
#12969=EDGE_CURVE('',#10242,#10240,#933,.T.);
#12970=EDGE_CURVE('',#10243,#10241,#934,.T.);
#12971=EDGE_CURVE('',#10243,#10244,#6256,.T.);
#12972=EDGE_CURVE('',#10244,#10242,#935,.T.);
#12973=EDGE_CURVE('',#10245,#10243,#936,.T.);
#12974=EDGE_CURVE('',#10245,#10246,#6257,.T.);
#12975=EDGE_CURVE('',#10246,#10244,#937,.T.);
#12976=EDGE_CURVE('',#10247,#10245,#938,.T.);
#12977=EDGE_CURVE('',#10247,#10248,#6258,.T.);
#12978=EDGE_CURVE('',#10248,#10246,#939,.T.);
#12979=EDGE_CURVE('',#10249,#10247,#940,.T.);
#12980=EDGE_CURVE('',#10249,#10250,#6259,.T.);
#12981=EDGE_CURVE('',#10250,#10248,#941,.T.);
#12982=EDGE_CURVE('',#10251,#10249,#942,.T.);
#12983=EDGE_CURVE('',#10251,#10252,#6260,.T.);
#12984=EDGE_CURVE('',#10252,#10250,#943,.T.);
#12985=EDGE_CURVE('',#10253,#10251,#944,.T.);
#12986=EDGE_CURVE('',#10253,#10254,#6261,.T.);
#12987=EDGE_CURVE('',#10254,#10252,#945,.T.);
#12988=EDGE_CURVE('',#10255,#10253,#946,.T.);
#12989=EDGE_CURVE('',#10255,#10256,#6262,.T.);
#12990=EDGE_CURVE('',#10256,#10254,#947,.T.);
#12991=EDGE_CURVE('',#10257,#10255,#948,.T.);
#12992=EDGE_CURVE('',#10257,#10258,#6263,.T.);
#12993=EDGE_CURVE('',#10258,#10256,#949,.T.);
#12994=EDGE_CURVE('',#10259,#10257,#950,.T.);
#12995=EDGE_CURVE('',#10259,#10260,#6264,.T.);
#12996=EDGE_CURVE('',#10260,#10258,#951,.T.);
#12997=EDGE_CURVE('',#10261,#10259,#952,.T.);
#12998=EDGE_CURVE('',#10261,#10262,#6265,.T.);
#12999=EDGE_CURVE('',#10262,#10260,#953,.T.);
#13000=EDGE_CURVE('',#10263,#10261,#6266,.T.);
#13001=EDGE_CURVE('',#10263,#10264,#6267,.T.);
#13002=EDGE_CURVE('',#10264,#10262,#6268,.T.);
#13003=EDGE_CURVE('',#10265,#10263,#954,.T.);
#13004=EDGE_CURVE('',#10265,#10266,#6269,.T.);
#13005=EDGE_CURVE('',#10266,#10264,#955,.T.);
#13006=EDGE_CURVE('',#10198,#10265,#956,.T.);
#13007=EDGE_CURVE('',#10200,#10266,#957,.T.);
#13008=EDGE_CURVE('',#10267,#10268,#958,.T.);
#13009=EDGE_CURVE('',#10267,#10269,#6270,.T.);
#13010=EDGE_CURVE('',#10269,#10270,#959,.T.);
#13011=EDGE_CURVE('',#10268,#10270,#6271,.T.);
#13012=EDGE_CURVE('',#10271,#10267,#960,.T.);
#13013=EDGE_CURVE('',#10271,#10272,#6272,.T.);
#13014=EDGE_CURVE('',#10272,#10269,#961,.T.);
#13015=EDGE_CURVE('',#10273,#10271,#962,.T.);
#13016=EDGE_CURVE('',#10273,#10274,#6273,.T.);
#13017=EDGE_CURVE('',#10274,#10272,#963,.T.);
#13018=EDGE_CURVE('',#10275,#10273,#964,.T.);
#13019=EDGE_CURVE('',#10275,#10276,#6274,.T.);
#13020=EDGE_CURVE('',#10276,#10274,#965,.T.);
#13021=EDGE_CURVE('',#10277,#10275,#966,.T.);
#13022=EDGE_CURVE('',#10277,#10278,#6275,.T.);
#13023=EDGE_CURVE('',#10278,#10276,#967,.T.);
#13024=EDGE_CURVE('',#10279,#10277,#968,.T.);
#13025=EDGE_CURVE('',#10279,#10280,#6276,.T.);
#13026=EDGE_CURVE('',#10280,#10278,#969,.T.);
#13027=EDGE_CURVE('',#10281,#10279,#970,.T.);
#13028=EDGE_CURVE('',#10281,#10282,#6277,.T.);
#13029=EDGE_CURVE('',#10282,#10280,#971,.T.);
#13030=EDGE_CURVE('',#10283,#10281,#972,.T.);
#13031=EDGE_CURVE('',#10283,#10284,#6278,.T.);
#13032=EDGE_CURVE('',#10284,#10282,#973,.T.);
#13033=EDGE_CURVE('',#10285,#10283,#974,.T.);
#13034=EDGE_CURVE('',#10285,#10286,#6279,.T.);
#13035=EDGE_CURVE('',#10286,#10284,#975,.T.);
#13036=EDGE_CURVE('',#10287,#10285,#976,.T.);
#13037=EDGE_CURVE('',#10287,#10288,#6280,.T.);
#13038=EDGE_CURVE('',#10288,#10286,#977,.T.);
#13039=EDGE_CURVE('',#10289,#10287,#978,.T.);
#13040=EDGE_CURVE('',#10289,#10290,#6281,.T.);
#13041=EDGE_CURVE('',#10290,#10288,#979,.T.);
#13042=EDGE_CURVE('',#10291,#10289,#6282,.T.);
#13043=EDGE_CURVE('',#10291,#10292,#6283,.T.);
#13044=EDGE_CURVE('',#10292,#10290,#6284,.T.);
#13045=EDGE_CURVE('',#10293,#10291,#980,.T.);
#13046=EDGE_CURVE('',#10293,#10294,#6285,.T.);
#13047=EDGE_CURVE('',#10294,#10292,#981,.T.);
#13048=EDGE_CURVE('',#10295,#10293,#982,.T.);
#13049=EDGE_CURVE('',#10295,#10296,#6286,.T.);
#13050=EDGE_CURVE('',#10296,#10294,#983,.T.);
#13051=EDGE_CURVE('',#10297,#10295,#984,.T.);
#13052=EDGE_CURVE('',#10297,#10298,#6287,.T.);
#13053=EDGE_CURVE('',#10298,#10296,#985,.T.);
#13054=EDGE_CURVE('',#10299,#10297,#986,.T.);
#13055=EDGE_CURVE('',#10299,#10300,#6288,.T.);
#13056=EDGE_CURVE('',#10300,#10298,#987,.T.);
#13057=EDGE_CURVE('',#10301,#10299,#988,.T.);
#13058=EDGE_CURVE('',#10301,#10302,#6289,.T.);
#13059=EDGE_CURVE('',#10302,#10300,#989,.T.);
#13060=EDGE_CURVE('',#10303,#10301,#990,.T.);
#13061=EDGE_CURVE('',#10303,#10304,#6290,.T.);
#13062=EDGE_CURVE('',#10304,#10302,#991,.T.);
#13063=EDGE_CURVE('',#10305,#10303,#992,.T.);
#13064=EDGE_CURVE('',#10305,#10306,#6291,.T.);
#13065=EDGE_CURVE('',#10306,#10304,#993,.T.);
#13066=EDGE_CURVE('',#10307,#10305,#6292,.T.);
#13067=EDGE_CURVE('',#10307,#10308,#6293,.T.);
#13068=EDGE_CURVE('',#10308,#10306,#6294,.T.);
#13069=EDGE_CURVE('',#10309,#10307,#994,.T.);
#13070=EDGE_CURVE('',#10309,#10310,#6295,.T.);
#13071=EDGE_CURVE('',#10310,#10308,#995,.T.);
#13072=EDGE_CURVE('',#10311,#10309,#996,.T.);
#13073=EDGE_CURVE('',#10311,#10312,#6296,.T.);
#13074=EDGE_CURVE('',#10312,#10310,#997,.T.);
#13075=EDGE_CURVE('',#10313,#10311,#998,.T.);
#13076=EDGE_CURVE('',#10313,#10314,#6297,.T.);
#13077=EDGE_CURVE('',#10314,#10312,#999,.T.);
#13078=EDGE_CURVE('',#10315,#10313,#1000,.T.);
#13079=EDGE_CURVE('',#10315,#10316,#6298,.T.);
#13080=EDGE_CURVE('',#10316,#10314,#1001,.T.);
#13081=EDGE_CURVE('',#10317,#10315,#1002,.T.);
#13082=EDGE_CURVE('',#10317,#10318,#6299,.T.);
#13083=EDGE_CURVE('',#10318,#10316,#1003,.T.);
#13084=EDGE_CURVE('',#10319,#10317,#1004,.T.);
#13085=EDGE_CURVE('',#10319,#10320,#6300,.T.);
#13086=EDGE_CURVE('',#10320,#10318,#1005,.T.);
#13087=EDGE_CURVE('',#10321,#10319,#1006,.T.);
#13088=EDGE_CURVE('',#10321,#10322,#6301,.T.);
#13089=EDGE_CURVE('',#10322,#10320,#1007,.T.);
#13090=EDGE_CURVE('',#10323,#10321,#6302,.T.);
#13091=EDGE_CURVE('',#10323,#10324,#6303,.T.);
#13092=EDGE_CURVE('',#10324,#10322,#6304,.T.);
#13093=EDGE_CURVE('',#10325,#10323,#1008,.T.);
#13094=EDGE_CURVE('',#10325,#10326,#6305,.T.);
#13095=EDGE_CURVE('',#10326,#10324,#1009,.T.);
#13096=EDGE_CURVE('',#10268,#10325,#1010,.T.);
#13097=EDGE_CURVE('',#10270,#10326,#1011,.T.);
#13098=EDGE_CURVE('',#10327,#10328,#1012,.T.);
#13099=EDGE_CURVE('',#10327,#10329,#6306,.T.);
#13100=EDGE_CURVE('',#10329,#10330,#1013,.T.);
#13101=EDGE_CURVE('',#10328,#10330,#6307,.T.);
#13102=EDGE_CURVE('',#10331,#10327,#1014,.T.);
#13103=EDGE_CURVE('',#10331,#10332,#6308,.T.);
#13104=EDGE_CURVE('',#10332,#10329,#1015,.T.);
#13105=EDGE_CURVE('',#10333,#10331,#1016,.T.);
#13106=EDGE_CURVE('',#10333,#10334,#6309,.T.);
#13107=EDGE_CURVE('',#10334,#10332,#1017,.T.);
#13108=EDGE_CURVE('',#10335,#10333,#1018,.T.);
#13109=EDGE_CURVE('',#10335,#10336,#6310,.T.);
#13110=EDGE_CURVE('',#10336,#10334,#1019,.T.);
#13111=EDGE_CURVE('',#10337,#10335,#1020,.T.);
#13112=EDGE_CURVE('',#10337,#10338,#6311,.T.);
#13113=EDGE_CURVE('',#10338,#10336,#1021,.T.);
#13114=EDGE_CURVE('',#10339,#10337,#1022,.T.);
#13115=EDGE_CURVE('',#10339,#10340,#6312,.T.);
#13116=EDGE_CURVE('',#10340,#10338,#1023,.T.);
#13117=EDGE_CURVE('',#10341,#10339,#1024,.T.);
#13118=EDGE_CURVE('',#10341,#10342,#6313,.T.);
#13119=EDGE_CURVE('',#10342,#10340,#1025,.T.);
#13120=EDGE_CURVE('',#10343,#10341,#1026,.T.);
#13121=EDGE_CURVE('',#10343,#10344,#6314,.T.);
#13122=EDGE_CURVE('',#10344,#10342,#1027,.T.);
#13123=EDGE_CURVE('',#10345,#10343,#6315,.T.);
#13124=EDGE_CURVE('',#10345,#10346,#6316,.T.);
#13125=EDGE_CURVE('',#10346,#10344,#6317,.T.);
#13126=EDGE_CURVE('',#10347,#10345,#1028,.T.);
#13127=EDGE_CURVE('',#10347,#10348,#6318,.T.);
#13128=EDGE_CURVE('',#10348,#10346,#1029,.T.);
#13129=EDGE_CURVE('',#10349,#10347,#1030,.T.);
#13130=EDGE_CURVE('',#10349,#10350,#6319,.T.);
#13131=EDGE_CURVE('',#10350,#10348,#1031,.T.);
#13132=EDGE_CURVE('',#10351,#10349,#1032,.T.);
#13133=EDGE_CURVE('',#10351,#10352,#6320,.T.);
#13134=EDGE_CURVE('',#10352,#10350,#1033,.T.);
#13135=EDGE_CURVE('',#10353,#10351,#1034,.T.);
#13136=EDGE_CURVE('',#10353,#10354,#6321,.T.);
#13137=EDGE_CURVE('',#10354,#10352,#1035,.T.);
#13138=EDGE_CURVE('',#10355,#10353,#1036,.T.);
#13139=EDGE_CURVE('',#10355,#10356,#6322,.T.);
#13140=EDGE_CURVE('',#10356,#10354,#1037,.T.);
#13141=EDGE_CURVE('',#10357,#10355,#1038,.T.);
#13142=EDGE_CURVE('',#10357,#10358,#6323,.T.);
#13143=EDGE_CURVE('',#10358,#10356,#1039,.T.);
#13144=EDGE_CURVE('',#10359,#10357,#1040,.T.);
#13145=EDGE_CURVE('',#10359,#10360,#6324,.T.);
#13146=EDGE_CURVE('',#10360,#10358,#1041,.T.);
#13147=EDGE_CURVE('',#10361,#10359,#1042,.T.);
#13148=EDGE_CURVE('',#10361,#10362,#6325,.T.);
#13149=EDGE_CURVE('',#10362,#10360,#1043,.T.);
#13150=EDGE_CURVE('',#10363,#10361,#1044,.T.);
#13151=EDGE_CURVE('',#10363,#10364,#6326,.T.);
#13152=EDGE_CURVE('',#10364,#10362,#1045,.T.);
#13153=EDGE_CURVE('',#10365,#10363,#6327,.T.);
#13154=EDGE_CURVE('',#10365,#10366,#6328,.T.);
#13155=EDGE_CURVE('',#10366,#10364,#6329,.T.);
#13156=EDGE_CURVE('',#10367,#10365,#6330,.T.);
#13157=EDGE_CURVE('',#10367,#10368,#6331,.T.);
#13158=EDGE_CURVE('',#10368,#10366,#6332,.T.);
#13159=EDGE_CURVE('',#10369,#10367,#6333,.T.);
#13160=EDGE_CURVE('',#10369,#10370,#6334,.T.);
#13161=EDGE_CURVE('',#10370,#10368,#6335,.T.);
#13162=EDGE_CURVE('',#10328,#10369,#1046,.T.);
#13163=EDGE_CURVE('',#10330,#10370,#1047,.T.);
#13164=EDGE_CURVE('',#10371,#10372,#6336,.T.);
#13165=EDGE_CURVE('',#10371,#10373,#6337,.T.);
#13166=EDGE_CURVE('',#10373,#10374,#6338,.T.);
#13167=EDGE_CURVE('',#10372,#10374,#6339,.T.);
#13168=EDGE_CURVE('',#10375,#10371,#1048,.T.);
#13169=EDGE_CURVE('',#10375,#10376,#6340,.T.);
#13170=EDGE_CURVE('',#10376,#10373,#1049,.T.);
#13171=EDGE_CURVE('',#10377,#10375,#1050,.T.);
#13172=EDGE_CURVE('',#10377,#10378,#6341,.T.);
#13173=EDGE_CURVE('',#10378,#10376,#1051,.T.);
#13174=EDGE_CURVE('',#10379,#10377,#1052,.T.);
#13175=EDGE_CURVE('',#10379,#10380,#6342,.T.);
#13176=EDGE_CURVE('',#10380,#10378,#1053,.T.);
#13177=EDGE_CURVE('',#10381,#10379,#1054,.T.);
#13178=EDGE_CURVE('',#10381,#10382,#6343,.T.);
#13179=EDGE_CURVE('',#10382,#10380,#1055,.T.);
#13180=EDGE_CURVE('',#10383,#10381,#1056,.T.);
#13181=EDGE_CURVE('',#10383,#10384,#6344,.T.);
#13182=EDGE_CURVE('',#10384,#10382,#1057,.T.);
#13183=EDGE_CURVE('',#10385,#10383,#6345,.T.);
#13184=EDGE_CURVE('',#10385,#10386,#6346,.T.);
#13185=EDGE_CURVE('',#10386,#10384,#6347,.T.);
#13186=EDGE_CURVE('',#10372,#10385,#6348,.T.);
#13187=EDGE_CURVE('',#10374,#10386,#6349,.T.);
#13188=EDGE_CURVE('',#10387,#10388,#6350,.T.);
#13189=EDGE_CURVE('',#10387,#10389,#6351,.T.);
#13190=EDGE_CURVE('',#10389,#10390,#6352,.T.);
#13191=EDGE_CURVE('',#10388,#10390,#6353,.T.);
#13192=EDGE_CURVE('',#10391,#10387,#1058,.T.);
#13193=EDGE_CURVE('',#10391,#10392,#6354,.T.);
#13194=EDGE_CURVE('',#10392,#10389,#1059,.T.);
#13195=EDGE_CURVE('',#10393,#10391,#1060,.T.);
#13196=EDGE_CURVE('',#10393,#10394,#6355,.T.);
#13197=EDGE_CURVE('',#10394,#10392,#1061,.T.);
#13198=EDGE_CURVE('',#10395,#10393,#1062,.T.);
#13199=EDGE_CURVE('',#10395,#10396,#6356,.T.);
#13200=EDGE_CURVE('',#10396,#10394,#1063,.T.);
#13201=EDGE_CURVE('',#10397,#10395,#1064,.T.);
#13202=EDGE_CURVE('',#10397,#10398,#6357,.T.);
#13203=EDGE_CURVE('',#10398,#10396,#1065,.T.);
#13204=EDGE_CURVE('',#10399,#10397,#1066,.T.);
#13205=EDGE_CURVE('',#10399,#10400,#6358,.T.);
#13206=EDGE_CURVE('',#10400,#10398,#1067,.T.);
#13207=EDGE_CURVE('',#10401,#10399,#1068,.T.);
#13208=EDGE_CURVE('',#10401,#10402,#6359,.T.);
#13209=EDGE_CURVE('',#10402,#10400,#1069,.T.);
#13210=EDGE_CURVE('',#10403,#10401,#6360,.T.);
#13211=EDGE_CURVE('',#10403,#10404,#6361,.T.);
#13212=EDGE_CURVE('',#10404,#10402,#6362,.T.);
#13213=EDGE_CURVE('',#10405,#10403,#6363,.T.);
#13214=EDGE_CURVE('',#10405,#10406,#6364,.T.);
#13215=EDGE_CURVE('',#10406,#10404,#6365,.T.);
#13216=EDGE_CURVE('',#10407,#10405,#6366,.T.);
#13217=EDGE_CURVE('',#10407,#10408,#6367,.T.);
#13218=EDGE_CURVE('',#10408,#10406,#6368,.T.);
#13219=EDGE_CURVE('',#10388,#10407,#6369,.T.);
#13220=EDGE_CURVE('',#10390,#10408,#6370,.T.);
#13221=EDGE_CURVE('',#10409,#10410,#1070,.T.);
#13222=EDGE_CURVE('',#10409,#10411,#6371,.T.);
#13223=EDGE_CURVE('',#10411,#10412,#1071,.T.);
#13224=EDGE_CURVE('',#10410,#10412,#6372,.T.);
#13225=EDGE_CURVE('',#10413,#10409,#1072,.T.);
#13226=EDGE_CURVE('',#10413,#10414,#6373,.T.);
#13227=EDGE_CURVE('',#10414,#10411,#1073,.T.);
#13228=EDGE_CURVE('',#10415,#10413,#1074,.T.);
#13229=EDGE_CURVE('',#10415,#10416,#6374,.T.);
#13230=EDGE_CURVE('',#10416,#10414,#1075,.T.);
#13231=EDGE_CURVE('',#10417,#10415,#1076,.T.);
#13232=EDGE_CURVE('',#10417,#10418,#6375,.T.);
#13233=EDGE_CURVE('',#10418,#10416,#1077,.T.);
#13234=EDGE_CURVE('',#10419,#10417,#1078,.T.);
#13235=EDGE_CURVE('',#10419,#10420,#6376,.T.);
#13236=EDGE_CURVE('',#10420,#10418,#1079,.T.);
#13237=EDGE_CURVE('',#10421,#10419,#1080,.T.);
#13238=EDGE_CURVE('',#10421,#10422,#6377,.T.);
#13239=EDGE_CURVE('',#10422,#10420,#1081,.T.);
#13240=EDGE_CURVE('',#10423,#10421,#1082,.T.);
#13241=EDGE_CURVE('',#10423,#10424,#6378,.T.);
#13242=EDGE_CURVE('',#10424,#10422,#1083,.T.);
#13243=EDGE_CURVE('',#10425,#10423,#1084,.T.);
#13244=EDGE_CURVE('',#10425,#10426,#6379,.T.);
#13245=EDGE_CURVE('',#10426,#10424,#1085,.T.);
#13246=EDGE_CURVE('',#10410,#10425,#1086,.T.);
#13247=EDGE_CURVE('',#10412,#10426,#1087,.T.);
#13248=EDGE_CURVE('',#10427,#10428,#1088,.T.);
#13249=EDGE_CURVE('',#10427,#10429,#6380,.T.);
#13250=EDGE_CURVE('',#10429,#10430,#1089,.T.);
#13251=EDGE_CURVE('',#10428,#10430,#6381,.T.);
#13252=EDGE_CURVE('',#10431,#10427,#1090,.T.);
#13253=EDGE_CURVE('',#10431,#10432,#6382,.T.);
#13254=EDGE_CURVE('',#10432,#10429,#1091,.T.);
#13255=EDGE_CURVE('',#10433,#10431,#1092,.T.);
#13256=EDGE_CURVE('',#10433,#10434,#6383,.T.);
#13257=EDGE_CURVE('',#10434,#10432,#1093,.T.);
#13258=EDGE_CURVE('',#10435,#10433,#1094,.T.);
#13259=EDGE_CURVE('',#10435,#10436,#6384,.T.);
#13260=EDGE_CURVE('',#10436,#10434,#1095,.T.);
#13261=EDGE_CURVE('',#10437,#10435,#1096,.T.);
#13262=EDGE_CURVE('',#10437,#10438,#6385,.T.);
#13263=EDGE_CURVE('',#10438,#10436,#1097,.T.);
#13264=EDGE_CURVE('',#10439,#10437,#1098,.T.);
#13265=EDGE_CURVE('',#10439,#10440,#6386,.T.);
#13266=EDGE_CURVE('',#10440,#10438,#1099,.T.);
#13267=EDGE_CURVE('',#10441,#10439,#1100,.T.);
#13268=EDGE_CURVE('',#10441,#10442,#6387,.T.);
#13269=EDGE_CURVE('',#10442,#10440,#1101,.T.);
#13270=EDGE_CURVE('',#10443,#10441,#1102,.T.);
#13271=EDGE_CURVE('',#10443,#10444,#6388,.T.);
#13272=EDGE_CURVE('',#10444,#10442,#1103,.T.);
#13273=EDGE_CURVE('',#10445,#10443,#1104,.T.);
#13274=EDGE_CURVE('',#10445,#10446,#6389,.T.);
#13275=EDGE_CURVE('',#10446,#10444,#1105,.T.);
#13276=EDGE_CURVE('',#10447,#10445,#1106,.T.);
#13277=EDGE_CURVE('',#10447,#10448,#6390,.T.);
#13278=EDGE_CURVE('',#10448,#10446,#1107,.T.);
#13279=EDGE_CURVE('',#10449,#10447,#1108,.T.);
#13280=EDGE_CURVE('',#10449,#10450,#6391,.T.);
#13281=EDGE_CURVE('',#10450,#10448,#1109,.T.);
#13282=EDGE_CURVE('',#10451,#10449,#1110,.T.);
#13283=EDGE_CURVE('',#10451,#10452,#6392,.T.);
#13284=EDGE_CURVE('',#10452,#10450,#1111,.T.);
#13285=EDGE_CURVE('',#10453,#10451,#1112,.T.);
#13286=EDGE_CURVE('',#10453,#10454,#6393,.T.);
#13287=EDGE_CURVE('',#10454,#10452,#1113,.T.);
#13288=EDGE_CURVE('',#10455,#10453,#1114,.T.);
#13289=EDGE_CURVE('',#10455,#10456,#6394,.T.);
#13290=EDGE_CURVE('',#10456,#10454,#1115,.T.);
#13291=EDGE_CURVE('',#10457,#10455,#1116,.T.);
#13292=EDGE_CURVE('',#10457,#10458,#6395,.T.);
#13293=EDGE_CURVE('',#10458,#10456,#1117,.T.);
#13294=EDGE_CURVE('',#10459,#10457,#1118,.T.);
#13295=EDGE_CURVE('',#10459,#10460,#6396,.T.);
#13296=EDGE_CURVE('',#10460,#10458,#1119,.T.);
#13297=EDGE_CURVE('',#10461,#10459,#6397,.T.);
#13298=EDGE_CURVE('',#10461,#10462,#6398,.T.);
#13299=EDGE_CURVE('',#10462,#10460,#6399,.T.);
#13300=EDGE_CURVE('',#10463,#10461,#1120,.T.);
#13301=EDGE_CURVE('',#10463,#10464,#6400,.T.);
#13302=EDGE_CURVE('',#10464,#10462,#1121,.T.);
#13303=EDGE_CURVE('',#10428,#10463,#1122,.T.);
#13304=EDGE_CURVE('',#10430,#10464,#1123,.T.);
#13305=EDGE_CURVE('',#10465,#10466,#1124,.T.);
#13306=EDGE_CURVE('',#10465,#10467,#6401,.T.);
#13307=EDGE_CURVE('',#10467,#10468,#1125,.T.);
#13308=EDGE_CURVE('',#10466,#10468,#6402,.T.);
#13309=EDGE_CURVE('',#10469,#10465,#1126,.T.);
#13310=EDGE_CURVE('',#10469,#10470,#6403,.T.);
#13311=EDGE_CURVE('',#10470,#10467,#1127,.T.);
#13312=EDGE_CURVE('',#10471,#10469,#1128,.T.);
#13313=EDGE_CURVE('',#10471,#10472,#6404,.T.);
#13314=EDGE_CURVE('',#10472,#10470,#1129,.T.);
#13315=EDGE_CURVE('',#10473,#10471,#1130,.T.);
#13316=EDGE_CURVE('',#10473,#10474,#6405,.T.);
#13317=EDGE_CURVE('',#10474,#10472,#1131,.T.);
#13318=EDGE_CURVE('',#10475,#10473,#1132,.T.);
#13319=EDGE_CURVE('',#10475,#10476,#6406,.T.);
#13320=EDGE_CURVE('',#10476,#10474,#1133,.T.);
#13321=EDGE_CURVE('',#10477,#10475,#1134,.T.);
#13322=EDGE_CURVE('',#10477,#10478,#6407,.T.);
#13323=EDGE_CURVE('',#10478,#10476,#1135,.T.);
#13324=EDGE_CURVE('',#10479,#10477,#1136,.T.);
#13325=EDGE_CURVE('',#10479,#10480,#6408,.T.);
#13326=EDGE_CURVE('',#10480,#10478,#1137,.T.);
#13327=EDGE_CURVE('',#10466,#10479,#1138,.T.);
#13328=EDGE_CURVE('',#10468,#10480,#1139,.T.);
#13329=EDGE_CURVE('',#10481,#10482,#1140,.T.);
#13330=EDGE_CURVE('',#10481,#10483,#6409,.T.);
#13331=EDGE_CURVE('',#10483,#10484,#1141,.T.);
#13332=EDGE_CURVE('',#10482,#10484,#6410,.T.);
#13333=EDGE_CURVE('',#10485,#10481,#1142,.T.);
#13334=EDGE_CURVE('',#10485,#10486,#6411,.T.);
#13335=EDGE_CURVE('',#10486,#10483,#1143,.T.);
#13336=EDGE_CURVE('',#10487,#10485,#1144,.T.);
#13337=EDGE_CURVE('',#10487,#10488,#6412,.T.);
#13338=EDGE_CURVE('',#10488,#10486,#1145,.T.);
#13339=EDGE_CURVE('',#10489,#10487,#1146,.T.);
#13340=EDGE_CURVE('',#10489,#10490,#6413,.T.);
#13341=EDGE_CURVE('',#10490,#10488,#1147,.T.);
#13342=EDGE_CURVE('',#10491,#10489,#1148,.T.);
#13343=EDGE_CURVE('',#10491,#10492,#6414,.T.);
#13344=EDGE_CURVE('',#10492,#10490,#1149,.T.);
#13345=EDGE_CURVE('',#10493,#10491,#1150,.T.);
#13346=EDGE_CURVE('',#10493,#10494,#6415,.T.);
#13347=EDGE_CURVE('',#10494,#10492,#1151,.T.);
#13348=EDGE_CURVE('',#10495,#10493,#1152,.T.);
#13349=EDGE_CURVE('',#10495,#10496,#6416,.T.);
#13350=EDGE_CURVE('',#10496,#10494,#1153,.T.);
#13351=EDGE_CURVE('',#10497,#10495,#6417,.T.);
#13352=EDGE_CURVE('',#10497,#10498,#6418,.T.);
#13353=EDGE_CURVE('',#10498,#10496,#6419,.T.);
#13354=EDGE_CURVE('',#10499,#10497,#6420,.T.);
#13355=EDGE_CURVE('',#10499,#10500,#6421,.T.);
#13356=EDGE_CURVE('',#10500,#10498,#6422,.T.);
#13357=EDGE_CURVE('',#10501,#10499,#6423,.T.);
#13358=EDGE_CURVE('',#10501,#10502,#6424,.T.);
#13359=EDGE_CURVE('',#10502,#10500,#6425,.T.);
#13360=EDGE_CURVE('',#10503,#10501,#6426,.T.);
#13361=EDGE_CURVE('',#10503,#10504,#6427,.T.);
#13362=EDGE_CURVE('',#10504,#10502,#6428,.T.);
#13363=EDGE_CURVE('',#10505,#10503,#6429,.T.);
#13364=EDGE_CURVE('',#10505,#10506,#6430,.T.);
#13365=EDGE_CURVE('',#10506,#10504,#6431,.T.);
#13366=EDGE_CURVE('',#10482,#10505,#1154,.T.);
#13367=EDGE_CURVE('',#10484,#10506,#1155,.T.);
#13368=EDGE_CURVE('',#10507,#10508,#1156,.T.);
#13369=EDGE_CURVE('',#10507,#10509,#6432,.T.);
#13370=EDGE_CURVE('',#10509,#10510,#1157,.T.);
#13371=EDGE_CURVE('',#10508,#10510,#6433,.T.);
#13372=EDGE_CURVE('',#10511,#10507,#1158,.T.);
#13373=EDGE_CURVE('',#10511,#10512,#6434,.T.);
#13374=EDGE_CURVE('',#10512,#10509,#1159,.T.);
#13375=EDGE_CURVE('',#10513,#10511,#1160,.T.);
#13376=EDGE_CURVE('',#10513,#10514,#6435,.T.);
#13377=EDGE_CURVE('',#10514,#10512,#1161,.T.);
#13378=EDGE_CURVE('',#10515,#10513,#1162,.T.);
#13379=EDGE_CURVE('',#10515,#10516,#6436,.T.);
#13380=EDGE_CURVE('',#10516,#10514,#1163,.T.);
#13381=EDGE_CURVE('',#10517,#10515,#6437,.T.);
#13382=EDGE_CURVE('',#10517,#10518,#6438,.T.);
#13383=EDGE_CURVE('',#10518,#10516,#6439,.T.);
#13384=EDGE_CURVE('',#10519,#10517,#1164,.T.);
#13385=EDGE_CURVE('',#10519,#10520,#6440,.T.);
#13386=EDGE_CURVE('',#10520,#10518,#1165,.T.);
#13387=EDGE_CURVE('',#10521,#10519,#1166,.T.);
#13388=EDGE_CURVE('',#10521,#10522,#6441,.T.);
#13389=EDGE_CURVE('',#10522,#10520,#1167,.T.);
#13390=EDGE_CURVE('',#10523,#10521,#1168,.T.);
#13391=EDGE_CURVE('',#10523,#10524,#6442,.T.);
#13392=EDGE_CURVE('',#10524,#10522,#1169,.T.);
#13393=EDGE_CURVE('',#10525,#10523,#6443,.T.);
#13394=EDGE_CURVE('',#10525,#10526,#6444,.T.);
#13395=EDGE_CURVE('',#10526,#10524,#6445,.T.);
#13396=EDGE_CURVE('',#10527,#10525,#6446,.T.);
#13397=EDGE_CURVE('',#10527,#10528,#6447,.T.);
#13398=EDGE_CURVE('',#10528,#10526,#6448,.T.);
#13399=EDGE_CURVE('',#10529,#10527,#6449,.T.);
#13400=EDGE_CURVE('',#10529,#10530,#6450,.T.);
#13401=EDGE_CURVE('',#10530,#10528,#6451,.T.);
#13402=EDGE_CURVE('',#10531,#10529,#6452,.T.);
#13403=EDGE_CURVE('',#10531,#10532,#6453,.T.);
#13404=EDGE_CURVE('',#10532,#10530,#6454,.T.);
#13405=EDGE_CURVE('',#10508,#10531,#6455,.T.);
#13406=EDGE_CURVE('',#10510,#10532,#6456,.T.);
#13407=EDGE_CURVE('',#10533,#10533,#8818,.T.);
#13408=EDGE_CURVE('',#10533,#10534,#6457,.T.);
#13409=EDGE_CURVE('',#10535,#10534,#1170,.T.);
#13410=EDGE_CURVE('',#10536,#10535,#1171,.T.);
#13411=EDGE_CURVE('',#10537,#10536,#1172,.T.);
#13412=EDGE_CURVE('',#10534,#10537,#1173,.T.);
#13413=EDGE_CURVE('',#10538,#10538,#8819,.T.);
#13414=EDGE_CURVE('',#10538,#10539,#6458,.T.);
#13415=EDGE_CURVE('',#10539,#10539,#8820,.T.);
#13416=EDGE_CURVE('',#10540,#10540,#8821,.T.);
#13417=EDGE_CURVE('',#10540,#10539,#6459,.T.);
#13418=EDGE_CURVE('',#10541,#10542,#6460,.T.);
#13419=EDGE_CURVE('',#10543,#10541,#1174,.T.);
#13420=EDGE_CURVE('',#10544,#10543,#6461,.T.);
#13421=EDGE_CURVE('',#10542,#10544,#6462,.T.);
#13422=EDGE_CURVE('',#10545,#10546,#6463,.T.);
#13423=EDGE_CURVE('',#10546,#10546,#8822,.T.);
#13424=EDGE_CURVE('',#10546,#10535,#6464,.T.);
#13425=EDGE_CURVE('',#10537,#10547,#6465,.T.);
#13426=EDGE_CURVE('',#10547,#10547,#8823,.T.);
#13427=EDGE_CURVE('',#10542,#10544,#8824,.T.);
#13428=EDGE_CURVE('',#10548,#10543,#8825,.T.);
#13429=EDGE_CURVE('',#10548,#10549,#6466,.T.);
#13430=EDGE_CURVE('',#10549,#10549,#8826,.T.);
#13431=EDGE_CURVE('',#10541,#10548,#8827,.T.);
#13432=EDGE_CURVE('',#10550,#10550,#8828,.T.);
#13433=EDGE_CURVE('',#10550,#10548,#8829,.T.);
#13434=EDGE_CURVE('',#10551,#10551,#8830,.T.);
#13435=EDGE_CURVE('',#10551,#10552,#6467,.T.);
#13436=EDGE_CURVE('',#10552,#10552,#8831,.T.);
#13437=EDGE_CURVE('',#10553,#10553,#8832,.T.);
#13438=EDGE_CURVE('',#10554,#10554,#8833,.T.);
#13439=EDGE_CURVE('',#10555,#10555,#8834,.T.);
#13440=EDGE_CURVE('',#10556,#10556,#8835,.T.);
#13441=EDGE_CURVE('',#10557,#10557,#8836,.T.);
#13442=EDGE_CURVE('',#10558,#10558,#8837,.T.);
#13443=EDGE_CURVE('',#10559,#10559,#8838,.T.);
#13444=EDGE_CURVE('',#10552,#10560,#6468,.T.);
#13445=EDGE_CURVE('',#10560,#10560,#8839,.T.);
#13446=EDGE_CURVE('',#10559,#10561,#6469,.T.);
#13447=EDGE_CURVE('',#10561,#10561,#8840,.T.);
#13448=EDGE_CURVE('',#10561,#10562,#6470,.T.);
#13449=EDGE_CURVE('',#10562,#10562,#8841,.T.);
#13450=EDGE_CURVE('',#10554,#10563,#6471,.T.);
#13451=EDGE_CURVE('',#10563,#10563,#8842,.T.);
#13452=EDGE_CURVE('',#10563,#10564,#6472,.T.);
#13453=EDGE_CURVE('',#10564,#10564,#8843,.T.);
#13454=EDGE_CURVE('',#10558,#10565,#6473,.T.);
#13455=EDGE_CURVE('',#10565,#10565,#8844,.T.);
#13456=EDGE_CURVE('',#10565,#10566,#6474,.T.);
#13457=EDGE_CURVE('',#10566,#10566,#8845,.T.);
#13458=EDGE_CURVE('',#10555,#10567,#6475,.T.);
#13459=EDGE_CURVE('',#10567,#10567,#8846,.T.);
#13460=EDGE_CURVE('',#10567,#10568,#6476,.T.);
#13461=EDGE_CURVE('',#10568,#10568,#8847,.T.);
#13462=EDGE_CURVE('',#10557,#10569,#6477,.T.);
#13463=EDGE_CURVE('',#10569,#10569,#8848,.T.);
#13464=EDGE_CURVE('',#10569,#10570,#6478,.T.);
#13465=EDGE_CURVE('',#10570,#10570,#8849,.T.);
#13466=EDGE_CURVE('',#10570,#10571,#6479,.T.);
#13467=EDGE_CURVE('',#10568,#10572,#6480,.T.);
#13468=EDGE_CURVE('',#10566,#10573,#6481,.T.);
#13469=EDGE_CURVE('',#10564,#10574,#6482,.T.);
#13470=EDGE_CURVE('',#10562,#10575,#6483,.T.);
#13471=EDGE_CURVE('',#10560,#10576,#6484,.T.);
#13472=EDGE_CURVE('',#10556,#10577,#6485,.T.);
#13473=EDGE_CURVE('',#10577,#10578,#8850,.T.);
#13474=EDGE_CURVE('',#10578,#10577,#8851,.T.);
#13475=EDGE_CURVE('',#10579,#10579,#8852,.T.);
#13476=EDGE_CURVE('',#10579,#10578,#6486,.T.);
#13477=EDGE_CURVE('',#10549,#10553,#6487,.T.);
#13478=EDGE_CURVE('',#10580,#10580,#8853,.T.);
#13479=EDGE_CURVE('',#10580,#10581,#6488,.T.);
#13480=EDGE_CURVE('',#10581,#10581,#8854,.T.);
#17030=ORIENTED_EDGE('',*,*,#12519,.F.);
#17031=ORIENTED_EDGE('',*,*,#12520,.T.);
#17032=ORIENTED_EDGE('',*,*,#12521,.T.);
#17033=ORIENTED_EDGE('',*,*,#12522,.F.);
#17034=ORIENTED_EDGE('',*,*,#12523,.F.);
#17035=ORIENTED_EDGE('',*,*,#12524,.T.);
#17036=ORIENTED_EDGE('',*,*,#12525,.T.);
#17037=ORIENTED_EDGE('',*,*,#12520,.F.);
#17038=ORIENTED_EDGE('',*,*,#12526,.F.);
#17039=ORIENTED_EDGE('',*,*,#12527,.T.);
#17040=ORIENTED_EDGE('',*,*,#12528,.T.);
#17041=ORIENTED_EDGE('',*,*,#12524,.F.);
#17042=ORIENTED_EDGE('',*,*,#12529,.F.);
#17043=ORIENTED_EDGE('',*,*,#12530,.T.);
#17044=ORIENTED_EDGE('',*,*,#12531,.T.);
#17045=ORIENTED_EDGE('',*,*,#12527,.F.);
#17046=ORIENTED_EDGE('',*,*,#12532,.F.);
#17047=ORIENTED_EDGE('',*,*,#12533,.T.);
#17048=ORIENTED_EDGE('',*,*,#12534,.T.);
#17049=ORIENTED_EDGE('',*,*,#12530,.F.);
#17050=ORIENTED_EDGE('',*,*,#12535,.F.);
#17051=ORIENTED_EDGE('',*,*,#12536,.T.);
#17052=ORIENTED_EDGE('',*,*,#12537,.T.);
#17053=ORIENTED_EDGE('',*,*,#12533,.F.);
#17054=ORIENTED_EDGE('',*,*,#12538,.F.);
#17055=ORIENTED_EDGE('',*,*,#12539,.T.);
#17056=ORIENTED_EDGE('',*,*,#12540,.T.);
#17057=ORIENTED_EDGE('',*,*,#12536,.F.);
#17058=ORIENTED_EDGE('',*,*,#12541,.F.);
#17059=ORIENTED_EDGE('',*,*,#12542,.T.);
#17060=ORIENTED_EDGE('',*,*,#12543,.T.);
#17061=ORIENTED_EDGE('',*,*,#12539,.F.);
#17062=ORIENTED_EDGE('',*,*,#12544,.F.);
#17063=ORIENTED_EDGE('',*,*,#12545,.T.);
#17064=ORIENTED_EDGE('',*,*,#12546,.T.);
#17065=ORIENTED_EDGE('',*,*,#12542,.F.);
#17066=ORIENTED_EDGE('',*,*,#12547,.F.);
#17067=ORIENTED_EDGE('',*,*,#12522,.T.);
#17068=ORIENTED_EDGE('',*,*,#12548,.T.);
#17069=ORIENTED_EDGE('',*,*,#12545,.F.);
#17070=ORIENTED_EDGE('',*,*,#12549,.F.);
#17071=ORIENTED_EDGE('',*,*,#12550,.T.);
#17072=ORIENTED_EDGE('',*,*,#12551,.T.);
#17073=ORIENTED_EDGE('',*,*,#12552,.F.);
#17074=ORIENTED_EDGE('',*,*,#12553,.F.);
#17075=ORIENTED_EDGE('',*,*,#12554,.T.);
#17076=ORIENTED_EDGE('',*,*,#12555,.T.);
#17077=ORIENTED_EDGE('',*,*,#12550,.F.);
#17078=ORIENTED_EDGE('',*,*,#12556,.F.);
#17079=ORIENTED_EDGE('',*,*,#12557,.T.);
#17080=ORIENTED_EDGE('',*,*,#12558,.T.);
#17081=ORIENTED_EDGE('',*,*,#12554,.F.);
#17082=ORIENTED_EDGE('',*,*,#12559,.F.);
#17083=ORIENTED_EDGE('',*,*,#12560,.T.);
#17084=ORIENTED_EDGE('',*,*,#12561,.T.);
#17085=ORIENTED_EDGE('',*,*,#12557,.F.);
#17086=ORIENTED_EDGE('',*,*,#12562,.F.);
#17087=ORIENTED_EDGE('',*,*,#12563,.T.);
#17088=ORIENTED_EDGE('',*,*,#12564,.T.);
#17089=ORIENTED_EDGE('',*,*,#12560,.F.);
#17090=ORIENTED_EDGE('',*,*,#12565,.F.);
#17091=ORIENTED_EDGE('',*,*,#12566,.T.);
#17092=ORIENTED_EDGE('',*,*,#12567,.T.);
#17093=ORIENTED_EDGE('',*,*,#12563,.F.);
#17094=ORIENTED_EDGE('',*,*,#12568,.F.);
#17095=ORIENTED_EDGE('',*,*,#12569,.T.);
#17096=ORIENTED_EDGE('',*,*,#12570,.T.);
#17097=ORIENTED_EDGE('',*,*,#12566,.F.);
#17098=ORIENTED_EDGE('',*,*,#12571,.F.);
#17099=ORIENTED_EDGE('',*,*,#12572,.T.);
#17100=ORIENTED_EDGE('',*,*,#12573,.T.);
#17101=ORIENTED_EDGE('',*,*,#12569,.F.);
#17102=ORIENTED_EDGE('',*,*,#12574,.F.);
#17103=ORIENTED_EDGE('',*,*,#12575,.T.);
#17104=ORIENTED_EDGE('',*,*,#12576,.T.);
#17105=ORIENTED_EDGE('',*,*,#12572,.F.);
#17106=ORIENTED_EDGE('',*,*,#12577,.F.);
#17107=ORIENTED_EDGE('',*,*,#12578,.T.);
#17108=ORIENTED_EDGE('',*,*,#12579,.T.);
#17109=ORIENTED_EDGE('',*,*,#12575,.F.);
#17110=ORIENTED_EDGE('',*,*,#12580,.F.);
#17111=ORIENTED_EDGE('',*,*,#12581,.T.);
#17112=ORIENTED_EDGE('',*,*,#12582,.T.);
#17113=ORIENTED_EDGE('',*,*,#12578,.F.);
#17114=ORIENTED_EDGE('',*,*,#12583,.F.);
#17115=ORIENTED_EDGE('',*,*,#12584,.T.);
#17116=ORIENTED_EDGE('',*,*,#12585,.T.);
#17117=ORIENTED_EDGE('',*,*,#12581,.F.);
#17118=ORIENTED_EDGE('',*,*,#12586,.F.);
#17119=ORIENTED_EDGE('',*,*,#12587,.T.);
#17120=ORIENTED_EDGE('',*,*,#12588,.T.);
#17121=ORIENTED_EDGE('',*,*,#12584,.F.);
#17122=ORIENTED_EDGE('',*,*,#12589,.F.);
#17123=ORIENTED_EDGE('',*,*,#12590,.T.);
#17124=ORIENTED_EDGE('',*,*,#12591,.T.);
#17125=ORIENTED_EDGE('',*,*,#12587,.F.);
#17126=ORIENTED_EDGE('',*,*,#12592,.F.);
#17127=ORIENTED_EDGE('',*,*,#12593,.T.);
#17128=ORIENTED_EDGE('',*,*,#12594,.T.);
#17129=ORIENTED_EDGE('',*,*,#12590,.F.);
#17130=ORIENTED_EDGE('',*,*,#12595,.F.);
#17131=ORIENTED_EDGE('',*,*,#12596,.T.);
#17132=ORIENTED_EDGE('',*,*,#12597,.T.);
#17133=ORIENTED_EDGE('',*,*,#12593,.F.);
#17134=ORIENTED_EDGE('',*,*,#12598,.F.);
#17135=ORIENTED_EDGE('',*,*,#12599,.T.);
#17136=ORIENTED_EDGE('',*,*,#12600,.T.);
#17137=ORIENTED_EDGE('',*,*,#12596,.F.);
#17138=ORIENTED_EDGE('',*,*,#12601,.F.);
#17139=ORIENTED_EDGE('',*,*,#12602,.T.);
#17140=ORIENTED_EDGE('',*,*,#12603,.T.);
#17141=ORIENTED_EDGE('',*,*,#12599,.F.);
#17142=ORIENTED_EDGE('',*,*,#12604,.F.);
#17143=ORIENTED_EDGE('',*,*,#12605,.T.);
#17144=ORIENTED_EDGE('',*,*,#12606,.T.);
#17145=ORIENTED_EDGE('',*,*,#12602,.F.);
#17146=ORIENTED_EDGE('',*,*,#12607,.F.);
#17147=ORIENTED_EDGE('',*,*,#12608,.T.);
#17148=ORIENTED_EDGE('',*,*,#12609,.T.);
#17149=ORIENTED_EDGE('',*,*,#12605,.F.);
#17150=ORIENTED_EDGE('',*,*,#12610,.F.);
#17151=ORIENTED_EDGE('',*,*,#12611,.T.);
#17152=ORIENTED_EDGE('',*,*,#12612,.T.);
#17153=ORIENTED_EDGE('',*,*,#12608,.F.);
#17154=ORIENTED_EDGE('',*,*,#12613,.F.);
#17155=ORIENTED_EDGE('',*,*,#12614,.T.);
#17156=ORIENTED_EDGE('',*,*,#12615,.T.);
#17157=ORIENTED_EDGE('',*,*,#12611,.F.);
#17158=ORIENTED_EDGE('',*,*,#12616,.F.);
#17159=ORIENTED_EDGE('',*,*,#12617,.T.);
#17160=ORIENTED_EDGE('',*,*,#12618,.T.);
#17161=ORIENTED_EDGE('',*,*,#12614,.F.);
#17162=ORIENTED_EDGE('',*,*,#12619,.F.);
#17163=ORIENTED_EDGE('',*,*,#12620,.T.);
#17164=ORIENTED_EDGE('',*,*,#12621,.T.);
#17165=ORIENTED_EDGE('',*,*,#12617,.F.);
#17166=ORIENTED_EDGE('',*,*,#12622,.F.);
#17167=ORIENTED_EDGE('',*,*,#12623,.T.);
#17168=ORIENTED_EDGE('',*,*,#12624,.T.);
#17169=ORIENTED_EDGE('',*,*,#12620,.F.);
#17170=ORIENTED_EDGE('',*,*,#12625,.F.);
#17171=ORIENTED_EDGE('',*,*,#12626,.T.);
#17172=ORIENTED_EDGE('',*,*,#12627,.T.);
#17173=ORIENTED_EDGE('',*,*,#12623,.F.);
#17174=ORIENTED_EDGE('',*,*,#12628,.F.);
#17175=ORIENTED_EDGE('',*,*,#12552,.T.);
#17176=ORIENTED_EDGE('',*,*,#12629,.T.);
#17177=ORIENTED_EDGE('',*,*,#12626,.F.);
#17178=ORIENTED_EDGE('',*,*,#12629,.F.);
#17179=ORIENTED_EDGE('',*,*,#12551,.F.);
#17180=ORIENTED_EDGE('',*,*,#12555,.F.);
#17181=ORIENTED_EDGE('',*,*,#12558,.F.);
#17182=ORIENTED_EDGE('',*,*,#12561,.F.);
#17183=ORIENTED_EDGE('',*,*,#12564,.F.);
#17184=ORIENTED_EDGE('',*,*,#12567,.F.);
#17185=ORIENTED_EDGE('',*,*,#12570,.F.);
#17186=ORIENTED_EDGE('',*,*,#12573,.F.);
#17187=ORIENTED_EDGE('',*,*,#12576,.F.);
#17188=ORIENTED_EDGE('',*,*,#12579,.F.);
#17189=ORIENTED_EDGE('',*,*,#12582,.F.);
#17190=ORIENTED_EDGE('',*,*,#12585,.F.);
#17191=ORIENTED_EDGE('',*,*,#12588,.F.);
#17192=ORIENTED_EDGE('',*,*,#12591,.F.);
#17193=ORIENTED_EDGE('',*,*,#12594,.F.);
#17194=ORIENTED_EDGE('',*,*,#12597,.F.);
#17195=ORIENTED_EDGE('',*,*,#12600,.F.);
#17196=ORIENTED_EDGE('',*,*,#12603,.F.);
#17197=ORIENTED_EDGE('',*,*,#12606,.F.);
#17198=ORIENTED_EDGE('',*,*,#12609,.F.);
#17199=ORIENTED_EDGE('',*,*,#12612,.F.);
#17200=ORIENTED_EDGE('',*,*,#12615,.F.);
#17201=ORIENTED_EDGE('',*,*,#12618,.F.);
#17202=ORIENTED_EDGE('',*,*,#12621,.F.);
#17203=ORIENTED_EDGE('',*,*,#12624,.F.);
#17204=ORIENTED_EDGE('',*,*,#12627,.F.);
#17205=ORIENTED_EDGE('',*,*,#12548,.F.);
#17206=ORIENTED_EDGE('',*,*,#12521,.F.);
#17207=ORIENTED_EDGE('',*,*,#12525,.F.);
#17208=ORIENTED_EDGE('',*,*,#12528,.F.);
#17209=ORIENTED_EDGE('',*,*,#12531,.F.);
#17210=ORIENTED_EDGE('',*,*,#12534,.F.);
#17211=ORIENTED_EDGE('',*,*,#12537,.F.);
#17212=ORIENTED_EDGE('',*,*,#12540,.F.);
#17213=ORIENTED_EDGE('',*,*,#12543,.F.);
#17214=ORIENTED_EDGE('',*,*,#12546,.F.);
#17215=ORIENTED_EDGE('',*,*,#12630,.F.);
#17216=ORIENTED_EDGE('',*,*,#12631,.T.);
#17217=ORIENTED_EDGE('',*,*,#12632,.T.);
#17218=ORIENTED_EDGE('',*,*,#12633,.F.);
#17219=ORIENTED_EDGE('',*,*,#12634,.F.);
#17220=ORIENTED_EDGE('',*,*,#12635,.T.);
#17221=ORIENTED_EDGE('',*,*,#12636,.T.);
#17222=ORIENTED_EDGE('',*,*,#12631,.F.);
#17223=ORIENTED_EDGE('',*,*,#12637,.F.);
#17224=ORIENTED_EDGE('',*,*,#12638,.T.);
#17225=ORIENTED_EDGE('',*,*,#12639,.T.);
#17226=ORIENTED_EDGE('',*,*,#12635,.F.);
#17227=ORIENTED_EDGE('',*,*,#12640,.F.);
#17228=ORIENTED_EDGE('',*,*,#12641,.T.);
#17229=ORIENTED_EDGE('',*,*,#12642,.T.);
#17230=ORIENTED_EDGE('',*,*,#12638,.F.);
#17231=ORIENTED_EDGE('',*,*,#12643,.F.);
#17232=ORIENTED_EDGE('',*,*,#12644,.T.);
#17233=ORIENTED_EDGE('',*,*,#12645,.T.);
#17234=ORIENTED_EDGE('',*,*,#12641,.F.);
#17235=ORIENTED_EDGE('',*,*,#12646,.F.);
#17236=ORIENTED_EDGE('',*,*,#12647,.T.);
#17237=ORIENTED_EDGE('',*,*,#12648,.T.);
#17238=ORIENTED_EDGE('',*,*,#12644,.F.);
#17239=ORIENTED_EDGE('',*,*,#12649,.F.);
#17240=ORIENTED_EDGE('',*,*,#12650,.T.);
#17241=ORIENTED_EDGE('',*,*,#12651,.T.);
#17242=ORIENTED_EDGE('',*,*,#12647,.F.);
#17243=ORIENTED_EDGE('',*,*,#12652,.F.);
#17244=ORIENTED_EDGE('',*,*,#12633,.T.);
#17245=ORIENTED_EDGE('',*,*,#12653,.T.);
#17246=ORIENTED_EDGE('',*,*,#12650,.F.);
#17247=ORIENTED_EDGE('',*,*,#12654,.F.);
#17248=ORIENTED_EDGE('',*,*,#12655,.T.);
#17249=ORIENTED_EDGE('',*,*,#12656,.T.);
#17250=ORIENTED_EDGE('',*,*,#12657,.F.);
#17251=ORIENTED_EDGE('',*,*,#12658,.F.);
#17252=ORIENTED_EDGE('',*,*,#12659,.T.);
#17253=ORIENTED_EDGE('',*,*,#12660,.T.);
#17254=ORIENTED_EDGE('',*,*,#12655,.F.);
#17255=ORIENTED_EDGE('',*,*,#12661,.F.);
#17256=ORIENTED_EDGE('',*,*,#12662,.T.);
#17257=ORIENTED_EDGE('',*,*,#12663,.T.);
#17258=ORIENTED_EDGE('',*,*,#12659,.F.);
#17259=ORIENTED_EDGE('',*,*,#12664,.F.);
#17260=ORIENTED_EDGE('',*,*,#12665,.T.);
#17261=ORIENTED_EDGE('',*,*,#12666,.T.);
#17262=ORIENTED_EDGE('',*,*,#12662,.F.);
#17263=ORIENTED_EDGE('',*,*,#12667,.F.);
#17264=ORIENTED_EDGE('',*,*,#12668,.T.);
#17265=ORIENTED_EDGE('',*,*,#12669,.T.);
#17266=ORIENTED_EDGE('',*,*,#12665,.F.);
#17267=ORIENTED_EDGE('',*,*,#12670,.F.);
#17268=ORIENTED_EDGE('',*,*,#12671,.T.);
#17269=ORIENTED_EDGE('',*,*,#12672,.T.);
#17270=ORIENTED_EDGE('',*,*,#12668,.F.);
#17271=ORIENTED_EDGE('',*,*,#12673,.F.);
#17272=ORIENTED_EDGE('',*,*,#12674,.T.);
#17273=ORIENTED_EDGE('',*,*,#12675,.T.);
#17274=ORIENTED_EDGE('',*,*,#12671,.F.);
#17275=ORIENTED_EDGE('',*,*,#12676,.F.);
#17276=ORIENTED_EDGE('',*,*,#12677,.T.);
#17277=ORIENTED_EDGE('',*,*,#12678,.T.);
#17278=ORIENTED_EDGE('',*,*,#12674,.F.);
#17279=ORIENTED_EDGE('',*,*,#12679,.F.);
#17280=ORIENTED_EDGE('',*,*,#12680,.T.);
#17281=ORIENTED_EDGE('',*,*,#12681,.T.);
#17282=ORIENTED_EDGE('',*,*,#12677,.F.);
#17283=ORIENTED_EDGE('',*,*,#12682,.F.);
#17284=ORIENTED_EDGE('',*,*,#12683,.T.);
#17285=ORIENTED_EDGE('',*,*,#12684,.T.);
#17286=ORIENTED_EDGE('',*,*,#12680,.F.);
#17287=ORIENTED_EDGE('',*,*,#12685,.F.);
#17288=ORIENTED_EDGE('',*,*,#12686,.T.);
#17289=ORIENTED_EDGE('',*,*,#12687,.T.);
#17290=ORIENTED_EDGE('',*,*,#12683,.F.);
#17291=ORIENTED_EDGE('',*,*,#12688,.F.);
#17292=ORIENTED_EDGE('',*,*,#12657,.T.);
#17293=ORIENTED_EDGE('',*,*,#12689,.T.);
#17294=ORIENTED_EDGE('',*,*,#12686,.F.);
#17295=ORIENTED_EDGE('',*,*,#12689,.F.);
#17296=ORIENTED_EDGE('',*,*,#12656,.F.);
#17297=ORIENTED_EDGE('',*,*,#12660,.F.);
#17298=ORIENTED_EDGE('',*,*,#12663,.F.);
#17299=ORIENTED_EDGE('',*,*,#12666,.F.);
#17300=ORIENTED_EDGE('',*,*,#12669,.F.);
#17301=ORIENTED_EDGE('',*,*,#12672,.F.);
#17302=ORIENTED_EDGE('',*,*,#12675,.F.);
#17303=ORIENTED_EDGE('',*,*,#12678,.F.);
#17304=ORIENTED_EDGE('',*,*,#12681,.F.);
#17305=ORIENTED_EDGE('',*,*,#12684,.F.);
#17306=ORIENTED_EDGE('',*,*,#12687,.F.);
#17307=ORIENTED_EDGE('',*,*,#12653,.F.);
#17308=ORIENTED_EDGE('',*,*,#12632,.F.);
#17309=ORIENTED_EDGE('',*,*,#12636,.F.);
#17310=ORIENTED_EDGE('',*,*,#12639,.F.);
#17311=ORIENTED_EDGE('',*,*,#12642,.F.);
#17312=ORIENTED_EDGE('',*,*,#12645,.F.);
#17313=ORIENTED_EDGE('',*,*,#12648,.F.);
#17314=ORIENTED_EDGE('',*,*,#12651,.F.);
#17315=ORIENTED_EDGE('',*,*,#12690,.F.);
#17316=ORIENTED_EDGE('',*,*,#12691,.T.);
#17317=ORIENTED_EDGE('',*,*,#12692,.T.);
#17318=ORIENTED_EDGE('',*,*,#12693,.F.);
#17319=ORIENTED_EDGE('',*,*,#12694,.F.);
#17320=ORIENTED_EDGE('',*,*,#12695,.T.);
#17321=ORIENTED_EDGE('',*,*,#12696,.T.);
#17322=ORIENTED_EDGE('',*,*,#12691,.F.);
#17323=ORIENTED_EDGE('',*,*,#12697,.F.);
#17324=ORIENTED_EDGE('',*,*,#12698,.T.);
#17325=ORIENTED_EDGE('',*,*,#12699,.T.);
#17326=ORIENTED_EDGE('',*,*,#12695,.F.);
#17327=ORIENTED_EDGE('',*,*,#12700,.F.);
#17328=ORIENTED_EDGE('',*,*,#12701,.T.);
#17329=ORIENTED_EDGE('',*,*,#12702,.T.);
#17330=ORIENTED_EDGE('',*,*,#12698,.F.);
#17331=ORIENTED_EDGE('',*,*,#12703,.F.);
#17332=ORIENTED_EDGE('',*,*,#12704,.T.);
#17333=ORIENTED_EDGE('',*,*,#12705,.T.);
#17334=ORIENTED_EDGE('',*,*,#12701,.F.);
#17335=ORIENTED_EDGE('',*,*,#12706,.F.);
#17336=ORIENTED_EDGE('',*,*,#12707,.T.);
#17337=ORIENTED_EDGE('',*,*,#12708,.T.);
#17338=ORIENTED_EDGE('',*,*,#12704,.F.);
#17339=ORIENTED_EDGE('',*,*,#12709,.F.);
#17340=ORIENTED_EDGE('',*,*,#12710,.T.);
#17341=ORIENTED_EDGE('',*,*,#12711,.T.);
#17342=ORIENTED_EDGE('',*,*,#12707,.F.);
#17343=ORIENTED_EDGE('',*,*,#12712,.F.);
#17344=ORIENTED_EDGE('',*,*,#12713,.T.);
#17345=ORIENTED_EDGE('',*,*,#12714,.T.);
#17346=ORIENTED_EDGE('',*,*,#12710,.F.);
#17347=ORIENTED_EDGE('',*,*,#12715,.F.);
#17348=ORIENTED_EDGE('',*,*,#12693,.T.);
#17349=ORIENTED_EDGE('',*,*,#12716,.T.);
#17350=ORIENTED_EDGE('',*,*,#12713,.F.);
#17351=ORIENTED_EDGE('',*,*,#12716,.F.);
#17352=ORIENTED_EDGE('',*,*,#12692,.F.);
#17353=ORIENTED_EDGE('',*,*,#12696,.F.);
#17354=ORIENTED_EDGE('',*,*,#12699,.F.);
#17355=ORIENTED_EDGE('',*,*,#12702,.F.);
#17356=ORIENTED_EDGE('',*,*,#12705,.F.);
#17357=ORIENTED_EDGE('',*,*,#12708,.F.);
#17358=ORIENTED_EDGE('',*,*,#12711,.F.);
#17359=ORIENTED_EDGE('',*,*,#12714,.F.);
#17360=ORIENTED_EDGE('',*,*,#12717,.F.);
#17361=ORIENTED_EDGE('',*,*,#12718,.T.);
#17362=ORIENTED_EDGE('',*,*,#12719,.T.);
#17363=ORIENTED_EDGE('',*,*,#12720,.F.);
#17364=ORIENTED_EDGE('',*,*,#12721,.F.);
#17365=ORIENTED_EDGE('',*,*,#12722,.T.);
#17366=ORIENTED_EDGE('',*,*,#12723,.T.);
#17367=ORIENTED_EDGE('',*,*,#12718,.F.);
#17368=ORIENTED_EDGE('',*,*,#12724,.F.);
#17369=ORIENTED_EDGE('',*,*,#12725,.T.);
#17370=ORIENTED_EDGE('',*,*,#12726,.T.);
#17371=ORIENTED_EDGE('',*,*,#12722,.F.);
#17372=ORIENTED_EDGE('',*,*,#12727,.F.);
#17373=ORIENTED_EDGE('',*,*,#12728,.T.);
#17374=ORIENTED_EDGE('',*,*,#12729,.T.);
#17375=ORIENTED_EDGE('',*,*,#12725,.F.);
#17376=ORIENTED_EDGE('',*,*,#12730,.F.);
#17377=ORIENTED_EDGE('',*,*,#12731,.T.);
#17378=ORIENTED_EDGE('',*,*,#12732,.T.);
#17379=ORIENTED_EDGE('',*,*,#12728,.F.);
#17380=ORIENTED_EDGE('',*,*,#12733,.F.);
#17381=ORIENTED_EDGE('',*,*,#12734,.T.);
#17382=ORIENTED_EDGE('',*,*,#12735,.T.);
#17383=ORIENTED_EDGE('',*,*,#12731,.F.);
#17384=ORIENTED_EDGE('',*,*,#12736,.F.);
#17385=ORIENTED_EDGE('',*,*,#12737,.T.);
#17386=ORIENTED_EDGE('',*,*,#12738,.T.);
#17387=ORIENTED_EDGE('',*,*,#12734,.F.);
#17388=ORIENTED_EDGE('',*,*,#12739,.F.);
#17389=ORIENTED_EDGE('',*,*,#12740,.T.);
#17390=ORIENTED_EDGE('',*,*,#12741,.T.);
#17391=ORIENTED_EDGE('',*,*,#12737,.F.);
#17392=ORIENTED_EDGE('',*,*,#12742,.F.);
#17393=ORIENTED_EDGE('',*,*,#12743,.T.);
#17394=ORIENTED_EDGE('',*,*,#12744,.T.);
#17395=ORIENTED_EDGE('',*,*,#12740,.F.);
#17396=ORIENTED_EDGE('',*,*,#12745,.F.);
#17397=ORIENTED_EDGE('',*,*,#12746,.T.);
#17398=ORIENTED_EDGE('',*,*,#12747,.T.);
#17399=ORIENTED_EDGE('',*,*,#12743,.F.);
#17400=ORIENTED_EDGE('',*,*,#12748,.F.);
#17401=ORIENTED_EDGE('',*,*,#12749,.T.);
#17402=ORIENTED_EDGE('',*,*,#12750,.T.);
#17403=ORIENTED_EDGE('',*,*,#12746,.F.);
#17404=ORIENTED_EDGE('',*,*,#12751,.F.);
#17405=ORIENTED_EDGE('',*,*,#12752,.T.);
#17406=ORIENTED_EDGE('',*,*,#12753,.T.);
#17407=ORIENTED_EDGE('',*,*,#12749,.F.);
#17408=ORIENTED_EDGE('',*,*,#12754,.F.);
#17409=ORIENTED_EDGE('',*,*,#12755,.T.);
#17410=ORIENTED_EDGE('',*,*,#12756,.T.);
#17411=ORIENTED_EDGE('',*,*,#12752,.F.);
#17412=ORIENTED_EDGE('',*,*,#12757,.F.);
#17413=ORIENTED_EDGE('',*,*,#12758,.T.);
#17414=ORIENTED_EDGE('',*,*,#12759,.T.);
#17415=ORIENTED_EDGE('',*,*,#12755,.F.);
#17416=ORIENTED_EDGE('',*,*,#12760,.F.);
#17417=ORIENTED_EDGE('',*,*,#12720,.T.);
#17418=ORIENTED_EDGE('',*,*,#12761,.T.);
#17419=ORIENTED_EDGE('',*,*,#12758,.F.);
#17420=ORIENTED_EDGE('',*,*,#12761,.F.);
#17421=ORIENTED_EDGE('',*,*,#12719,.F.);
#17422=ORIENTED_EDGE('',*,*,#12723,.F.);
#17423=ORIENTED_EDGE('',*,*,#12726,.F.);
#17424=ORIENTED_EDGE('',*,*,#12729,.F.);
#17425=ORIENTED_EDGE('',*,*,#12732,.F.);
#17426=ORIENTED_EDGE('',*,*,#12735,.F.);
#17427=ORIENTED_EDGE('',*,*,#12738,.F.);
#17428=ORIENTED_EDGE('',*,*,#12741,.F.);
#17429=ORIENTED_EDGE('',*,*,#12744,.F.);
#17430=ORIENTED_EDGE('',*,*,#12747,.F.);
#17431=ORIENTED_EDGE('',*,*,#12750,.F.);
#17432=ORIENTED_EDGE('',*,*,#12753,.F.);
#17433=ORIENTED_EDGE('',*,*,#12756,.F.);
#17434=ORIENTED_EDGE('',*,*,#12759,.F.);
#17435=ORIENTED_EDGE('',*,*,#12762,.F.);
#17436=ORIENTED_EDGE('',*,*,#12763,.T.);
#17437=ORIENTED_EDGE('',*,*,#12764,.T.);
#17438=ORIENTED_EDGE('',*,*,#12765,.F.);
#17439=ORIENTED_EDGE('',*,*,#12766,.F.);
#17440=ORIENTED_EDGE('',*,*,#12767,.T.);
#17441=ORIENTED_EDGE('',*,*,#12768,.T.);
#17442=ORIENTED_EDGE('',*,*,#12763,.F.);
#17443=ORIENTED_EDGE('',*,*,#12769,.F.);
#17444=ORIENTED_EDGE('',*,*,#12770,.T.);
#17445=ORIENTED_EDGE('',*,*,#12771,.T.);
#17446=ORIENTED_EDGE('',*,*,#12767,.F.);
#17447=ORIENTED_EDGE('',*,*,#12772,.F.);
#17448=ORIENTED_EDGE('',*,*,#12773,.T.);
#17449=ORIENTED_EDGE('',*,*,#12774,.T.);
#17450=ORIENTED_EDGE('',*,*,#12770,.F.);
#17451=ORIENTED_EDGE('',*,*,#12775,.F.);
#17452=ORIENTED_EDGE('',*,*,#12776,.T.);
#17453=ORIENTED_EDGE('',*,*,#12777,.T.);
#17454=ORIENTED_EDGE('',*,*,#12773,.F.);
#17455=ORIENTED_EDGE('',*,*,#12778,.F.);
#17456=ORIENTED_EDGE('',*,*,#12779,.T.);
#17457=ORIENTED_EDGE('',*,*,#12780,.T.);
#17458=ORIENTED_EDGE('',*,*,#12776,.F.);
#17459=ORIENTED_EDGE('',*,*,#12781,.F.);
#17460=ORIENTED_EDGE('',*,*,#12782,.T.);
#17461=ORIENTED_EDGE('',*,*,#12783,.T.);
#17462=ORIENTED_EDGE('',*,*,#12779,.F.);
#17463=ORIENTED_EDGE('',*,*,#12784,.F.);
#17464=ORIENTED_EDGE('',*,*,#12785,.T.);
#17465=ORIENTED_EDGE('',*,*,#12786,.T.);
#17466=ORIENTED_EDGE('',*,*,#12782,.F.);
#17467=ORIENTED_EDGE('',*,*,#12787,.F.);
#17468=ORIENTED_EDGE('',*,*,#12788,.T.);
#17469=ORIENTED_EDGE('',*,*,#12789,.T.);
#17470=ORIENTED_EDGE('',*,*,#12785,.F.);
#17471=ORIENTED_EDGE('',*,*,#12790,.F.);
#17472=ORIENTED_EDGE('',*,*,#12791,.T.);
#17473=ORIENTED_EDGE('',*,*,#12792,.T.);
#17474=ORIENTED_EDGE('',*,*,#12788,.F.);
#17475=ORIENTED_EDGE('',*,*,#12793,.F.);
#17476=ORIENTED_EDGE('',*,*,#12794,.T.);
#17477=ORIENTED_EDGE('',*,*,#12795,.T.);
#17478=ORIENTED_EDGE('',*,*,#12791,.F.);
#17479=ORIENTED_EDGE('',*,*,#12796,.F.);
#17480=ORIENTED_EDGE('',*,*,#12797,.T.);
#17481=ORIENTED_EDGE('',*,*,#12798,.T.);
#17482=ORIENTED_EDGE('',*,*,#12794,.F.);
#17483=ORIENTED_EDGE('',*,*,#12799,.F.);
#17484=ORIENTED_EDGE('',*,*,#12800,.T.);
#17485=ORIENTED_EDGE('',*,*,#12801,.T.);
#17486=ORIENTED_EDGE('',*,*,#12797,.F.);
#17487=ORIENTED_EDGE('',*,*,#12802,.F.);
#17488=ORIENTED_EDGE('',*,*,#12803,.T.);
#17489=ORIENTED_EDGE('',*,*,#12804,.T.);
#17490=ORIENTED_EDGE('',*,*,#12800,.F.);
#17491=ORIENTED_EDGE('',*,*,#12805,.F.);
#17492=ORIENTED_EDGE('',*,*,#12806,.T.);
#17493=ORIENTED_EDGE('',*,*,#12807,.T.);
#17494=ORIENTED_EDGE('',*,*,#12803,.F.);
#17495=ORIENTED_EDGE('',*,*,#12808,.F.);
#17496=ORIENTED_EDGE('',*,*,#12809,.T.);
#17497=ORIENTED_EDGE('',*,*,#12810,.T.);
#17498=ORIENTED_EDGE('',*,*,#12806,.F.);
#17499=ORIENTED_EDGE('',*,*,#12811,.F.);
#17500=ORIENTED_EDGE('',*,*,#12812,.T.);
#17501=ORIENTED_EDGE('',*,*,#12813,.T.);
#17502=ORIENTED_EDGE('',*,*,#12809,.F.);
#17503=ORIENTED_EDGE('',*,*,#12814,.F.);
#17504=ORIENTED_EDGE('',*,*,#12815,.T.);
#17505=ORIENTED_EDGE('',*,*,#12816,.T.);
#17506=ORIENTED_EDGE('',*,*,#12812,.F.);
#17507=ORIENTED_EDGE('',*,*,#12817,.F.);
#17508=ORIENTED_EDGE('',*,*,#12818,.T.);
#17509=ORIENTED_EDGE('',*,*,#12819,.T.);
#17510=ORIENTED_EDGE('',*,*,#12815,.F.);
#17511=ORIENTED_EDGE('',*,*,#12820,.F.);
#17512=ORIENTED_EDGE('',*,*,#12821,.T.);
#17513=ORIENTED_EDGE('',*,*,#12822,.T.);
#17514=ORIENTED_EDGE('',*,*,#12818,.F.);
#17515=ORIENTED_EDGE('',*,*,#12823,.F.);
#17516=ORIENTED_EDGE('',*,*,#12824,.T.);
#17517=ORIENTED_EDGE('',*,*,#12825,.T.);
#17518=ORIENTED_EDGE('',*,*,#12821,.F.);
#17519=ORIENTED_EDGE('',*,*,#12826,.F.);
#17520=ORIENTED_EDGE('',*,*,#12827,.T.);
#17521=ORIENTED_EDGE('',*,*,#12828,.T.);
#17522=ORIENTED_EDGE('',*,*,#12824,.F.);
#17523=ORIENTED_EDGE('',*,*,#12829,.F.);
#17524=ORIENTED_EDGE('',*,*,#12830,.T.);
#17525=ORIENTED_EDGE('',*,*,#12831,.T.);
#17526=ORIENTED_EDGE('',*,*,#12827,.F.);
#17527=ORIENTED_EDGE('',*,*,#12832,.F.);
#17528=ORIENTED_EDGE('',*,*,#12833,.T.);
#17529=ORIENTED_EDGE('',*,*,#12834,.T.);
#17530=ORIENTED_EDGE('',*,*,#12830,.F.);
#17531=ORIENTED_EDGE('',*,*,#12835,.F.);
#17532=ORIENTED_EDGE('',*,*,#12836,.T.);
#17533=ORIENTED_EDGE('',*,*,#12837,.T.);
#17534=ORIENTED_EDGE('',*,*,#12833,.F.);
#17535=ORIENTED_EDGE('',*,*,#12838,.F.);
#17536=ORIENTED_EDGE('',*,*,#12839,.T.);
#17537=ORIENTED_EDGE('',*,*,#12840,.T.);
#17538=ORIENTED_EDGE('',*,*,#12836,.F.);
#17539=ORIENTED_EDGE('',*,*,#12841,.F.);
#17540=ORIENTED_EDGE('',*,*,#12842,.T.);
#17541=ORIENTED_EDGE('',*,*,#12843,.T.);
#17542=ORIENTED_EDGE('',*,*,#12839,.F.);
#17543=ORIENTED_EDGE('',*,*,#12844,.F.);
#17544=ORIENTED_EDGE('',*,*,#12845,.T.);
#17545=ORIENTED_EDGE('',*,*,#12846,.T.);
#17546=ORIENTED_EDGE('',*,*,#12842,.F.);
#17547=ORIENTED_EDGE('',*,*,#12847,.F.);
#17548=ORIENTED_EDGE('',*,*,#12848,.T.);
#17549=ORIENTED_EDGE('',*,*,#12849,.T.);
#17550=ORIENTED_EDGE('',*,*,#12845,.F.);
#17551=ORIENTED_EDGE('',*,*,#12850,.F.);
#17552=ORIENTED_EDGE('',*,*,#12765,.T.);
#17553=ORIENTED_EDGE('',*,*,#12851,.T.);
#17554=ORIENTED_EDGE('',*,*,#12848,.F.);
#17555=ORIENTED_EDGE('',*,*,#12851,.F.);
#17556=ORIENTED_EDGE('',*,*,#12764,.F.);
#17557=ORIENTED_EDGE('',*,*,#12768,.F.);
#17558=ORIENTED_EDGE('',*,*,#12771,.F.);
#17559=ORIENTED_EDGE('',*,*,#12774,.F.);
#17560=ORIENTED_EDGE('',*,*,#12777,.F.);
#17561=ORIENTED_EDGE('',*,*,#12780,.F.);
#17562=ORIENTED_EDGE('',*,*,#12783,.F.);
#17563=ORIENTED_EDGE('',*,*,#12786,.F.);
#17564=ORIENTED_EDGE('',*,*,#12789,.F.);
#17565=ORIENTED_EDGE('',*,*,#12792,.F.);
#17566=ORIENTED_EDGE('',*,*,#12795,.F.);
#17567=ORIENTED_EDGE('',*,*,#12798,.F.);
#17568=ORIENTED_EDGE('',*,*,#12801,.F.);
#17569=ORIENTED_EDGE('',*,*,#12804,.F.);
#17570=ORIENTED_EDGE('',*,*,#12807,.F.);
#17571=ORIENTED_EDGE('',*,*,#12810,.F.);
#17572=ORIENTED_EDGE('',*,*,#12813,.F.);
#17573=ORIENTED_EDGE('',*,*,#12816,.F.);
#17574=ORIENTED_EDGE('',*,*,#12819,.F.);
#17575=ORIENTED_EDGE('',*,*,#12822,.F.);
#17576=ORIENTED_EDGE('',*,*,#12825,.F.);
#17577=ORIENTED_EDGE('',*,*,#12828,.F.);
#17578=ORIENTED_EDGE('',*,*,#12831,.F.);
#17579=ORIENTED_EDGE('',*,*,#12834,.F.);
#17580=ORIENTED_EDGE('',*,*,#12837,.F.);
#17581=ORIENTED_EDGE('',*,*,#12840,.F.);
#17582=ORIENTED_EDGE('',*,*,#12843,.F.);
#17583=ORIENTED_EDGE('',*,*,#12846,.F.);
#17584=ORIENTED_EDGE('',*,*,#12849,.F.);
#17585=ORIENTED_EDGE('',*,*,#12852,.F.);
#17586=ORIENTED_EDGE('',*,*,#12853,.T.);
#17587=ORIENTED_EDGE('',*,*,#12854,.T.);
#17588=ORIENTED_EDGE('',*,*,#12855,.F.);
#17589=ORIENTED_EDGE('',*,*,#12856,.F.);
#17590=ORIENTED_EDGE('',*,*,#12857,.T.);
#17591=ORIENTED_EDGE('',*,*,#12858,.T.);
#17592=ORIENTED_EDGE('',*,*,#12853,.F.);
#17593=ORIENTED_EDGE('',*,*,#12859,.F.);
#17594=ORIENTED_EDGE('',*,*,#12860,.T.);
#17595=ORIENTED_EDGE('',*,*,#12861,.T.);
#17596=ORIENTED_EDGE('',*,*,#12857,.F.);
#17597=ORIENTED_EDGE('',*,*,#12862,.F.);
#17598=ORIENTED_EDGE('',*,*,#12855,.T.);
#17599=ORIENTED_EDGE('',*,*,#12863,.T.);
#17600=ORIENTED_EDGE('',*,*,#12860,.F.);
#17601=ORIENTED_EDGE('',*,*,#12863,.F.);
#17602=ORIENTED_EDGE('',*,*,#12854,.F.);
#17603=ORIENTED_EDGE('',*,*,#12858,.F.);
#17604=ORIENTED_EDGE('',*,*,#12861,.F.);
#17605=ORIENTED_EDGE('',*,*,#12864,.F.);
#17606=ORIENTED_EDGE('',*,*,#12865,.T.);
#17607=ORIENTED_EDGE('',*,*,#12866,.T.);
#17608=ORIENTED_EDGE('',*,*,#12867,.F.);
#17609=ORIENTED_EDGE('',*,*,#12868,.F.);
#17610=ORIENTED_EDGE('',*,*,#12869,.T.);
#17611=ORIENTED_EDGE('',*,*,#12870,.T.);
#17612=ORIENTED_EDGE('',*,*,#12865,.F.);
#17613=ORIENTED_EDGE('',*,*,#12871,.F.);
#17614=ORIENTED_EDGE('',*,*,#12872,.T.);
#17615=ORIENTED_EDGE('',*,*,#12873,.T.);
#17616=ORIENTED_EDGE('',*,*,#12869,.F.);
#17617=ORIENTED_EDGE('',*,*,#12874,.F.);
#17618=ORIENTED_EDGE('',*,*,#12875,.T.);
#17619=ORIENTED_EDGE('',*,*,#12876,.T.);
#17620=ORIENTED_EDGE('',*,*,#12872,.F.);
#17621=ORIENTED_EDGE('',*,*,#12877,.F.);
#17622=ORIENTED_EDGE('',*,*,#12867,.T.);
#17623=ORIENTED_EDGE('',*,*,#12878,.T.);
#17624=ORIENTED_EDGE('',*,*,#12875,.F.);
#17625=ORIENTED_EDGE('',*,*,#12879,.F.);
#17626=ORIENTED_EDGE('',*,*,#12880,.T.);
#17627=ORIENTED_EDGE('',*,*,#12881,.T.);
#17628=ORIENTED_EDGE('',*,*,#12882,.F.);
#17629=ORIENTED_EDGE('',*,*,#12883,.F.);
#17630=ORIENTED_EDGE('',*,*,#12884,.T.);
#17631=ORIENTED_EDGE('',*,*,#12885,.T.);
#17632=ORIENTED_EDGE('',*,*,#12880,.F.);
#17633=ORIENTED_EDGE('',*,*,#12886,.F.);
#17634=ORIENTED_EDGE('',*,*,#12887,.T.);
#17635=ORIENTED_EDGE('',*,*,#12888,.T.);
#17636=ORIENTED_EDGE('',*,*,#12884,.F.);
#17637=ORIENTED_EDGE('',*,*,#12889,.F.);
#17638=ORIENTED_EDGE('',*,*,#12890,.T.);
#17639=ORIENTED_EDGE('',*,*,#12891,.T.);
#17640=ORIENTED_EDGE('',*,*,#12887,.F.);
#17641=ORIENTED_EDGE('',*,*,#12892,.F.);
#17642=ORIENTED_EDGE('',*,*,#12893,.T.);
#17643=ORIENTED_EDGE('',*,*,#12894,.T.);
#17644=ORIENTED_EDGE('',*,*,#12890,.F.);
#17645=ORIENTED_EDGE('',*,*,#12895,.F.);
#17646=ORIENTED_EDGE('',*,*,#12896,.T.);
#17647=ORIENTED_EDGE('',*,*,#12897,.T.);
#17648=ORIENTED_EDGE('',*,*,#12893,.F.);
#17649=ORIENTED_EDGE('',*,*,#12898,.F.);
#17650=ORIENTED_EDGE('',*,*,#12899,.T.);
#17651=ORIENTED_EDGE('',*,*,#12900,.T.);
#17652=ORIENTED_EDGE('',*,*,#12896,.F.);
#17653=ORIENTED_EDGE('',*,*,#12901,.F.);
#17654=ORIENTED_EDGE('',*,*,#12882,.T.);
#17655=ORIENTED_EDGE('',*,*,#12902,.T.);
#17656=ORIENTED_EDGE('',*,*,#12899,.F.);
#17657=ORIENTED_EDGE('',*,*,#12902,.F.);
#17658=ORIENTED_EDGE('',*,*,#12881,.F.);
#17659=ORIENTED_EDGE('',*,*,#12885,.F.);
#17660=ORIENTED_EDGE('',*,*,#12888,.F.);
#17661=ORIENTED_EDGE('',*,*,#12891,.F.);
#17662=ORIENTED_EDGE('',*,*,#12894,.F.);
#17663=ORIENTED_EDGE('',*,*,#12897,.F.);
#17664=ORIENTED_EDGE('',*,*,#12900,.F.);
#17665=ORIENTED_EDGE('',*,*,#12878,.F.);
#17666=ORIENTED_EDGE('',*,*,#12866,.F.);
#17667=ORIENTED_EDGE('',*,*,#12870,.F.);
#17668=ORIENTED_EDGE('',*,*,#12873,.F.);
#17669=ORIENTED_EDGE('',*,*,#12876,.F.);
#17670=ORIENTED_EDGE('',*,*,#12903,.F.);
#17671=ORIENTED_EDGE('',*,*,#12904,.T.);
#17672=ORIENTED_EDGE('',*,*,#12905,.T.);
#17673=ORIENTED_EDGE('',*,*,#12906,.F.);
#17674=ORIENTED_EDGE('',*,*,#12907,.F.);
#17675=ORIENTED_EDGE('',*,*,#12908,.T.);
#17676=ORIENTED_EDGE('',*,*,#12909,.T.);
#17677=ORIENTED_EDGE('',*,*,#12904,.F.);
#17678=ORIENTED_EDGE('',*,*,#12910,.F.);
#17679=ORIENTED_EDGE('',*,*,#12911,.T.);
#17680=ORIENTED_EDGE('',*,*,#12912,.T.);
#17681=ORIENTED_EDGE('',*,*,#12908,.F.);
#17682=ORIENTED_EDGE('',*,*,#12913,.F.);
#17683=ORIENTED_EDGE('',*,*,#12914,.T.);
#17684=ORIENTED_EDGE('',*,*,#12915,.T.);
#17685=ORIENTED_EDGE('',*,*,#12911,.F.);
#17686=ORIENTED_EDGE('',*,*,#12916,.F.);
#17687=ORIENTED_EDGE('',*,*,#12917,.T.);
#17688=ORIENTED_EDGE('',*,*,#12918,.T.);
#17689=ORIENTED_EDGE('',*,*,#12914,.F.);
#17690=ORIENTED_EDGE('',*,*,#12919,.F.);
#17691=ORIENTED_EDGE('',*,*,#12920,.T.);
#17692=ORIENTED_EDGE('',*,*,#12921,.T.);
#17693=ORIENTED_EDGE('',*,*,#12917,.F.);
#17694=ORIENTED_EDGE('',*,*,#12922,.F.);
#17695=ORIENTED_EDGE('',*,*,#12923,.T.);
#17696=ORIENTED_EDGE('',*,*,#12924,.T.);
#17697=ORIENTED_EDGE('',*,*,#12920,.F.);
#17698=ORIENTED_EDGE('',*,*,#12925,.F.);
#17699=ORIENTED_EDGE('',*,*,#12926,.T.);
#17700=ORIENTED_EDGE('',*,*,#12927,.T.);
#17701=ORIENTED_EDGE('',*,*,#12923,.F.);
#17702=ORIENTED_EDGE('',*,*,#12928,.F.);
#17703=ORIENTED_EDGE('',*,*,#12929,.T.);
#17704=ORIENTED_EDGE('',*,*,#12930,.T.);
#17705=ORIENTED_EDGE('',*,*,#12926,.F.);
#17706=ORIENTED_EDGE('',*,*,#12931,.F.);
#17707=ORIENTED_EDGE('',*,*,#12932,.T.);
#17708=ORIENTED_EDGE('',*,*,#12933,.T.);
#17709=ORIENTED_EDGE('',*,*,#12929,.F.);
#17710=ORIENTED_EDGE('',*,*,#12934,.F.);
#17711=ORIENTED_EDGE('',*,*,#12935,.T.);
#17712=ORIENTED_EDGE('',*,*,#12936,.T.);
#17713=ORIENTED_EDGE('',*,*,#12932,.F.);
#17714=ORIENTED_EDGE('',*,*,#12937,.F.);
#17715=ORIENTED_EDGE('',*,*,#12938,.T.);
#17716=ORIENTED_EDGE('',*,*,#12939,.T.);
#17717=ORIENTED_EDGE('',*,*,#12935,.F.);
#17718=ORIENTED_EDGE('',*,*,#12940,.F.);
#17719=ORIENTED_EDGE('',*,*,#12941,.T.);
#17720=ORIENTED_EDGE('',*,*,#12942,.T.);
#17721=ORIENTED_EDGE('',*,*,#12938,.F.);
#17722=ORIENTED_EDGE('',*,*,#12943,.F.);
#17723=ORIENTED_EDGE('',*,*,#12944,.T.);
#17724=ORIENTED_EDGE('',*,*,#12945,.T.);
#17725=ORIENTED_EDGE('',*,*,#12941,.F.);
#17726=ORIENTED_EDGE('',*,*,#12946,.F.);
#17727=ORIENTED_EDGE('',*,*,#12947,.T.);
#17728=ORIENTED_EDGE('',*,*,#12948,.T.);
#17729=ORIENTED_EDGE('',*,*,#12944,.F.);
#17730=ORIENTED_EDGE('',*,*,#12949,.F.);
#17731=ORIENTED_EDGE('',*,*,#12950,.T.);
#17732=ORIENTED_EDGE('',*,*,#12951,.T.);
#17733=ORIENTED_EDGE('',*,*,#12947,.F.);
#17734=ORIENTED_EDGE('',*,*,#12952,.F.);
#17735=ORIENTED_EDGE('',*,*,#12953,.T.);
#17736=ORIENTED_EDGE('',*,*,#12954,.T.);
#17737=ORIENTED_EDGE('',*,*,#12950,.F.);
#17738=ORIENTED_EDGE('',*,*,#12955,.F.);
#17739=ORIENTED_EDGE('',*,*,#12956,.T.);
#17740=ORIENTED_EDGE('',*,*,#12957,.T.);
#17741=ORIENTED_EDGE('',*,*,#12953,.F.);
#17742=ORIENTED_EDGE('',*,*,#12958,.F.);
#17743=ORIENTED_EDGE('',*,*,#12959,.T.);
#17744=ORIENTED_EDGE('',*,*,#12960,.T.);
#17745=ORIENTED_EDGE('',*,*,#12956,.F.);
#17746=ORIENTED_EDGE('',*,*,#12961,.F.);
#17747=ORIENTED_EDGE('',*,*,#12962,.T.);
#17748=ORIENTED_EDGE('',*,*,#12963,.T.);
#17749=ORIENTED_EDGE('',*,*,#12959,.F.);
#17750=ORIENTED_EDGE('',*,*,#12964,.F.);
#17751=ORIENTED_EDGE('',*,*,#12965,.T.);
#17752=ORIENTED_EDGE('',*,*,#12966,.T.);
#17753=ORIENTED_EDGE('',*,*,#12962,.F.);
#17754=ORIENTED_EDGE('',*,*,#12967,.F.);
#17755=ORIENTED_EDGE('',*,*,#12968,.T.);
#17756=ORIENTED_EDGE('',*,*,#12969,.T.);
#17757=ORIENTED_EDGE('',*,*,#12965,.F.);
#17758=ORIENTED_EDGE('',*,*,#12970,.F.);
#17759=ORIENTED_EDGE('',*,*,#12971,.T.);
#17760=ORIENTED_EDGE('',*,*,#12972,.T.);
#17761=ORIENTED_EDGE('',*,*,#12968,.F.);
#17762=ORIENTED_EDGE('',*,*,#12973,.F.);
#17763=ORIENTED_EDGE('',*,*,#12974,.T.);
#17764=ORIENTED_EDGE('',*,*,#12975,.T.);
#17765=ORIENTED_EDGE('',*,*,#12971,.F.);
#17766=ORIENTED_EDGE('',*,*,#12976,.F.);
#17767=ORIENTED_EDGE('',*,*,#12977,.T.);
#17768=ORIENTED_EDGE('',*,*,#12978,.T.);
#17769=ORIENTED_EDGE('',*,*,#12974,.F.);
#17770=ORIENTED_EDGE('',*,*,#12979,.F.);
#17771=ORIENTED_EDGE('',*,*,#12980,.T.);
#17772=ORIENTED_EDGE('',*,*,#12981,.T.);
#17773=ORIENTED_EDGE('',*,*,#12977,.F.);
#17774=ORIENTED_EDGE('',*,*,#12982,.F.);
#17775=ORIENTED_EDGE('',*,*,#12983,.T.);
#17776=ORIENTED_EDGE('',*,*,#12984,.T.);
#17777=ORIENTED_EDGE('',*,*,#12980,.F.);
#17778=ORIENTED_EDGE('',*,*,#12985,.F.);
#17779=ORIENTED_EDGE('',*,*,#12986,.T.);
#17780=ORIENTED_EDGE('',*,*,#12987,.T.);
#17781=ORIENTED_EDGE('',*,*,#12983,.F.);
#17782=ORIENTED_EDGE('',*,*,#12988,.F.);
#17783=ORIENTED_EDGE('',*,*,#12989,.T.);
#17784=ORIENTED_EDGE('',*,*,#12990,.T.);
#17785=ORIENTED_EDGE('',*,*,#12986,.F.);
#17786=ORIENTED_EDGE('',*,*,#12991,.F.);
#17787=ORIENTED_EDGE('',*,*,#12992,.T.);
#17788=ORIENTED_EDGE('',*,*,#12993,.T.);
#17789=ORIENTED_EDGE('',*,*,#12989,.F.);
#17790=ORIENTED_EDGE('',*,*,#12994,.F.);
#17791=ORIENTED_EDGE('',*,*,#12995,.T.);
#17792=ORIENTED_EDGE('',*,*,#12996,.T.);
#17793=ORIENTED_EDGE('',*,*,#12992,.F.);
#17794=ORIENTED_EDGE('',*,*,#12997,.F.);
#17795=ORIENTED_EDGE('',*,*,#12998,.T.);
#17796=ORIENTED_EDGE('',*,*,#12999,.T.);
#17797=ORIENTED_EDGE('',*,*,#12995,.F.);
#17798=ORIENTED_EDGE('',*,*,#13000,.F.);
#17799=ORIENTED_EDGE('',*,*,#13001,.T.);
#17800=ORIENTED_EDGE('',*,*,#13002,.T.);
#17801=ORIENTED_EDGE('',*,*,#12998,.F.);
#17802=ORIENTED_EDGE('',*,*,#13003,.F.);
#17803=ORIENTED_EDGE('',*,*,#13004,.T.);
#17804=ORIENTED_EDGE('',*,*,#13005,.T.);
#17805=ORIENTED_EDGE('',*,*,#13001,.F.);
#17806=ORIENTED_EDGE('',*,*,#13006,.F.);
#17807=ORIENTED_EDGE('',*,*,#12906,.T.);
#17808=ORIENTED_EDGE('',*,*,#13007,.T.);
#17809=ORIENTED_EDGE('',*,*,#13004,.F.);
#17810=ORIENTED_EDGE('',*,*,#13007,.F.);
#17811=ORIENTED_EDGE('',*,*,#12905,.F.);
#17812=ORIENTED_EDGE('',*,*,#12909,.F.);
#17813=ORIENTED_EDGE('',*,*,#12912,.F.);
#17814=ORIENTED_EDGE('',*,*,#12915,.F.);
#17815=ORIENTED_EDGE('',*,*,#12918,.F.);
#17816=ORIENTED_EDGE('',*,*,#12921,.F.);
#17817=ORIENTED_EDGE('',*,*,#12924,.F.);
#17818=ORIENTED_EDGE('',*,*,#12927,.F.);
#17819=ORIENTED_EDGE('',*,*,#12930,.F.);
#17820=ORIENTED_EDGE('',*,*,#12933,.F.);
#17821=ORIENTED_EDGE('',*,*,#12936,.F.);
#17822=ORIENTED_EDGE('',*,*,#12939,.F.);
#17823=ORIENTED_EDGE('',*,*,#12942,.F.);
#17824=ORIENTED_EDGE('',*,*,#12945,.F.);
#17825=ORIENTED_EDGE('',*,*,#12948,.F.);
#17826=ORIENTED_EDGE('',*,*,#12951,.F.);
#17827=ORIENTED_EDGE('',*,*,#12954,.F.);
#17828=ORIENTED_EDGE('',*,*,#12957,.F.);
#17829=ORIENTED_EDGE('',*,*,#12960,.F.);
#17830=ORIENTED_EDGE('',*,*,#12963,.F.);
#17831=ORIENTED_EDGE('',*,*,#12966,.F.);
#17832=ORIENTED_EDGE('',*,*,#12969,.F.);
#17833=ORIENTED_EDGE('',*,*,#12972,.F.);
#17834=ORIENTED_EDGE('',*,*,#12975,.F.);
#17835=ORIENTED_EDGE('',*,*,#12978,.F.);
#17836=ORIENTED_EDGE('',*,*,#12981,.F.);
#17837=ORIENTED_EDGE('',*,*,#12984,.F.);
#17838=ORIENTED_EDGE('',*,*,#12987,.F.);
#17839=ORIENTED_EDGE('',*,*,#12990,.F.);
#17840=ORIENTED_EDGE('',*,*,#12993,.F.);
#17841=ORIENTED_EDGE('',*,*,#12996,.F.);
#17842=ORIENTED_EDGE('',*,*,#12999,.F.);
#17843=ORIENTED_EDGE('',*,*,#13002,.F.);
#17844=ORIENTED_EDGE('',*,*,#13005,.F.);
#17845=ORIENTED_EDGE('',*,*,#13008,.F.);
#17846=ORIENTED_EDGE('',*,*,#13009,.T.);
#17847=ORIENTED_EDGE('',*,*,#13010,.T.);
#17848=ORIENTED_EDGE('',*,*,#13011,.F.);
#17849=ORIENTED_EDGE('',*,*,#13012,.F.);
#17850=ORIENTED_EDGE('',*,*,#13013,.T.);
#17851=ORIENTED_EDGE('',*,*,#13014,.T.);
#17852=ORIENTED_EDGE('',*,*,#13009,.F.);
#17853=ORIENTED_EDGE('',*,*,#13015,.F.);
#17854=ORIENTED_EDGE('',*,*,#13016,.T.);
#17855=ORIENTED_EDGE('',*,*,#13017,.T.);
#17856=ORIENTED_EDGE('',*,*,#13013,.F.);
#17857=ORIENTED_EDGE('',*,*,#13018,.F.);
#17858=ORIENTED_EDGE('',*,*,#13019,.T.);
#17859=ORIENTED_EDGE('',*,*,#13020,.T.);
#17860=ORIENTED_EDGE('',*,*,#13016,.F.);
#17861=ORIENTED_EDGE('',*,*,#13021,.F.);
#17862=ORIENTED_EDGE('',*,*,#13022,.T.);
#17863=ORIENTED_EDGE('',*,*,#13023,.T.);
#17864=ORIENTED_EDGE('',*,*,#13019,.F.);
#17865=ORIENTED_EDGE('',*,*,#13024,.F.);
#17866=ORIENTED_EDGE('',*,*,#13025,.T.);
#17867=ORIENTED_EDGE('',*,*,#13026,.T.);
#17868=ORIENTED_EDGE('',*,*,#13022,.F.);
#17869=ORIENTED_EDGE('',*,*,#13027,.F.);
#17870=ORIENTED_EDGE('',*,*,#13028,.T.);
#17871=ORIENTED_EDGE('',*,*,#13029,.T.);
#17872=ORIENTED_EDGE('',*,*,#13025,.F.);
#17873=ORIENTED_EDGE('',*,*,#13030,.F.);
#17874=ORIENTED_EDGE('',*,*,#13031,.T.);
#17875=ORIENTED_EDGE('',*,*,#13032,.T.);
#17876=ORIENTED_EDGE('',*,*,#13028,.F.);
#17877=ORIENTED_EDGE('',*,*,#13033,.F.);
#17878=ORIENTED_EDGE('',*,*,#13034,.T.);
#17879=ORIENTED_EDGE('',*,*,#13035,.T.);
#17880=ORIENTED_EDGE('',*,*,#13031,.F.);
#17881=ORIENTED_EDGE('',*,*,#13036,.F.);
#17882=ORIENTED_EDGE('',*,*,#13037,.T.);
#17883=ORIENTED_EDGE('',*,*,#13038,.T.);
#17884=ORIENTED_EDGE('',*,*,#13034,.F.);
#17885=ORIENTED_EDGE('',*,*,#13039,.F.);
#17886=ORIENTED_EDGE('',*,*,#13040,.T.);
#17887=ORIENTED_EDGE('',*,*,#13041,.T.);
#17888=ORIENTED_EDGE('',*,*,#13037,.F.);
#17889=ORIENTED_EDGE('',*,*,#13042,.F.);
#17890=ORIENTED_EDGE('',*,*,#13043,.T.);
#17891=ORIENTED_EDGE('',*,*,#13044,.T.);
#17892=ORIENTED_EDGE('',*,*,#13040,.F.);
#17893=ORIENTED_EDGE('',*,*,#13045,.F.);
#17894=ORIENTED_EDGE('',*,*,#13046,.T.);
#17895=ORIENTED_EDGE('',*,*,#13047,.T.);
#17896=ORIENTED_EDGE('',*,*,#13043,.F.);
#17897=ORIENTED_EDGE('',*,*,#13048,.F.);
#17898=ORIENTED_EDGE('',*,*,#13049,.T.);
#17899=ORIENTED_EDGE('',*,*,#13050,.T.);
#17900=ORIENTED_EDGE('',*,*,#13046,.F.);
#17901=ORIENTED_EDGE('',*,*,#13051,.F.);
#17902=ORIENTED_EDGE('',*,*,#13052,.T.);
#17903=ORIENTED_EDGE('',*,*,#13053,.T.);
#17904=ORIENTED_EDGE('',*,*,#13049,.F.);
#17905=ORIENTED_EDGE('',*,*,#13054,.F.);
#17906=ORIENTED_EDGE('',*,*,#13055,.T.);
#17907=ORIENTED_EDGE('',*,*,#13056,.T.);
#17908=ORIENTED_EDGE('',*,*,#13052,.F.);
#17909=ORIENTED_EDGE('',*,*,#13057,.F.);
#17910=ORIENTED_EDGE('',*,*,#13058,.T.);
#17911=ORIENTED_EDGE('',*,*,#13059,.T.);
#17912=ORIENTED_EDGE('',*,*,#13055,.F.);
#17913=ORIENTED_EDGE('',*,*,#13060,.F.);
#17914=ORIENTED_EDGE('',*,*,#13061,.T.);
#17915=ORIENTED_EDGE('',*,*,#13062,.T.);
#17916=ORIENTED_EDGE('',*,*,#13058,.F.);
#17917=ORIENTED_EDGE('',*,*,#13063,.F.);
#17918=ORIENTED_EDGE('',*,*,#13064,.T.);
#17919=ORIENTED_EDGE('',*,*,#13065,.T.);
#17920=ORIENTED_EDGE('',*,*,#13061,.F.);
#17921=ORIENTED_EDGE('',*,*,#13066,.F.);
#17922=ORIENTED_EDGE('',*,*,#13067,.T.);
#17923=ORIENTED_EDGE('',*,*,#13068,.T.);
#17924=ORIENTED_EDGE('',*,*,#13064,.F.);
#17925=ORIENTED_EDGE('',*,*,#13069,.F.);
#17926=ORIENTED_EDGE('',*,*,#13070,.T.);
#17927=ORIENTED_EDGE('',*,*,#13071,.T.);
#17928=ORIENTED_EDGE('',*,*,#13067,.F.);
#17929=ORIENTED_EDGE('',*,*,#13072,.F.);
#17930=ORIENTED_EDGE('',*,*,#13073,.T.);
#17931=ORIENTED_EDGE('',*,*,#13074,.T.);
#17932=ORIENTED_EDGE('',*,*,#13070,.F.);
#17933=ORIENTED_EDGE('',*,*,#13075,.F.);
#17934=ORIENTED_EDGE('',*,*,#13076,.T.);
#17935=ORIENTED_EDGE('',*,*,#13077,.T.);
#17936=ORIENTED_EDGE('',*,*,#13073,.F.);
#17937=ORIENTED_EDGE('',*,*,#13078,.F.);
#17938=ORIENTED_EDGE('',*,*,#13079,.T.);
#17939=ORIENTED_EDGE('',*,*,#13080,.T.);
#17940=ORIENTED_EDGE('',*,*,#13076,.F.);
#17941=ORIENTED_EDGE('',*,*,#13081,.F.);
#17942=ORIENTED_EDGE('',*,*,#13082,.T.);
#17943=ORIENTED_EDGE('',*,*,#13083,.T.);
#17944=ORIENTED_EDGE('',*,*,#13079,.F.);
#17945=ORIENTED_EDGE('',*,*,#13084,.F.);
#17946=ORIENTED_EDGE('',*,*,#13085,.T.);
#17947=ORIENTED_EDGE('',*,*,#13086,.T.);
#17948=ORIENTED_EDGE('',*,*,#13082,.F.);
#17949=ORIENTED_EDGE('',*,*,#13087,.F.);
#17950=ORIENTED_EDGE('',*,*,#13088,.T.);
#17951=ORIENTED_EDGE('',*,*,#13089,.T.);
#17952=ORIENTED_EDGE('',*,*,#13085,.F.);
#17953=ORIENTED_EDGE('',*,*,#13090,.F.);
#17954=ORIENTED_EDGE('',*,*,#13091,.T.);
#17955=ORIENTED_EDGE('',*,*,#13092,.T.);
#17956=ORIENTED_EDGE('',*,*,#13088,.F.);
#17957=ORIENTED_EDGE('',*,*,#13093,.F.);
#17958=ORIENTED_EDGE('',*,*,#13094,.T.);
#17959=ORIENTED_EDGE('',*,*,#13095,.T.);
#17960=ORIENTED_EDGE('',*,*,#13091,.F.);
#17961=ORIENTED_EDGE('',*,*,#13096,.F.);
#17962=ORIENTED_EDGE('',*,*,#13011,.T.);
#17963=ORIENTED_EDGE('',*,*,#13097,.T.);
#17964=ORIENTED_EDGE('',*,*,#13094,.F.);
#17965=ORIENTED_EDGE('',*,*,#13097,.F.);
#17966=ORIENTED_EDGE('',*,*,#13010,.F.);
#17967=ORIENTED_EDGE('',*,*,#13014,.F.);
#17968=ORIENTED_EDGE('',*,*,#13017,.F.);
#17969=ORIENTED_EDGE('',*,*,#13020,.F.);
#17970=ORIENTED_EDGE('',*,*,#13023,.F.);
#17971=ORIENTED_EDGE('',*,*,#13026,.F.);
#17972=ORIENTED_EDGE('',*,*,#13029,.F.);
#17973=ORIENTED_EDGE('',*,*,#13032,.F.);
#17974=ORIENTED_EDGE('',*,*,#13035,.F.);
#17975=ORIENTED_EDGE('',*,*,#13038,.F.);
#17976=ORIENTED_EDGE('',*,*,#13041,.F.);
#17977=ORIENTED_EDGE('',*,*,#13044,.F.);
#17978=ORIENTED_EDGE('',*,*,#13047,.F.);
#17979=ORIENTED_EDGE('',*,*,#13050,.F.);
#17980=ORIENTED_EDGE('',*,*,#13053,.F.);
#17981=ORIENTED_EDGE('',*,*,#13056,.F.);
#17982=ORIENTED_EDGE('',*,*,#13059,.F.);
#17983=ORIENTED_EDGE('',*,*,#13062,.F.);
#17984=ORIENTED_EDGE('',*,*,#13065,.F.);
#17985=ORIENTED_EDGE('',*,*,#13068,.F.);
#17986=ORIENTED_EDGE('',*,*,#13071,.F.);
#17987=ORIENTED_EDGE('',*,*,#13074,.F.);
#17988=ORIENTED_EDGE('',*,*,#13077,.F.);
#17989=ORIENTED_EDGE('',*,*,#13080,.F.);
#17990=ORIENTED_EDGE('',*,*,#13083,.F.);
#17991=ORIENTED_EDGE('',*,*,#13086,.F.);
#17992=ORIENTED_EDGE('',*,*,#13089,.F.);
#17993=ORIENTED_EDGE('',*,*,#13092,.F.);
#17994=ORIENTED_EDGE('',*,*,#13095,.F.);
#17995=ORIENTED_EDGE('',*,*,#13098,.F.);
#17996=ORIENTED_EDGE('',*,*,#13099,.T.);
#17997=ORIENTED_EDGE('',*,*,#13100,.T.);
#17998=ORIENTED_EDGE('',*,*,#13101,.F.);
#17999=ORIENTED_EDGE('',*,*,#13102,.F.);
#18000=ORIENTED_EDGE('',*,*,#13103,.T.);
#18001=ORIENTED_EDGE('',*,*,#13104,.T.);
#18002=ORIENTED_EDGE('',*,*,#13099,.F.);
#18003=ORIENTED_EDGE('',*,*,#13105,.F.);
#18004=ORIENTED_EDGE('',*,*,#13106,.T.);
#18005=ORIENTED_EDGE('',*,*,#13107,.T.);
#18006=ORIENTED_EDGE('',*,*,#13103,.F.);
#18007=ORIENTED_EDGE('',*,*,#13108,.F.);
#18008=ORIENTED_EDGE('',*,*,#13109,.T.);
#18009=ORIENTED_EDGE('',*,*,#13110,.T.);
#18010=ORIENTED_EDGE('',*,*,#13106,.F.);
#18011=ORIENTED_EDGE('',*,*,#13111,.F.);
#18012=ORIENTED_EDGE('',*,*,#13112,.T.);
#18013=ORIENTED_EDGE('',*,*,#13113,.T.);
#18014=ORIENTED_EDGE('',*,*,#13109,.F.);
#18015=ORIENTED_EDGE('',*,*,#13114,.F.);
#18016=ORIENTED_EDGE('',*,*,#13115,.T.);
#18017=ORIENTED_EDGE('',*,*,#13116,.T.);
#18018=ORIENTED_EDGE('',*,*,#13112,.F.);
#18019=ORIENTED_EDGE('',*,*,#13117,.F.);
#18020=ORIENTED_EDGE('',*,*,#13118,.T.);
#18021=ORIENTED_EDGE('',*,*,#13119,.T.);
#18022=ORIENTED_EDGE('',*,*,#13115,.F.);
#18023=ORIENTED_EDGE('',*,*,#13120,.F.);
#18024=ORIENTED_EDGE('',*,*,#13121,.T.);
#18025=ORIENTED_EDGE('',*,*,#13122,.T.);
#18026=ORIENTED_EDGE('',*,*,#13118,.F.);
#18027=ORIENTED_EDGE('',*,*,#13123,.F.);
#18028=ORIENTED_EDGE('',*,*,#13124,.T.);
#18029=ORIENTED_EDGE('',*,*,#13125,.T.);
#18030=ORIENTED_EDGE('',*,*,#13121,.F.);
#18031=ORIENTED_EDGE('',*,*,#13126,.F.);
#18032=ORIENTED_EDGE('',*,*,#13127,.T.);
#18033=ORIENTED_EDGE('',*,*,#13128,.T.);
#18034=ORIENTED_EDGE('',*,*,#13124,.F.);
#18035=ORIENTED_EDGE('',*,*,#13129,.F.);
#18036=ORIENTED_EDGE('',*,*,#13130,.T.);
#18037=ORIENTED_EDGE('',*,*,#13131,.T.);
#18038=ORIENTED_EDGE('',*,*,#13127,.F.);
#18039=ORIENTED_EDGE('',*,*,#13132,.F.);
#18040=ORIENTED_EDGE('',*,*,#13133,.T.);
#18041=ORIENTED_EDGE('',*,*,#13134,.T.);
#18042=ORIENTED_EDGE('',*,*,#13130,.F.);
#18043=ORIENTED_EDGE('',*,*,#13135,.F.);
#18044=ORIENTED_EDGE('',*,*,#13136,.T.);
#18045=ORIENTED_EDGE('',*,*,#13137,.T.);
#18046=ORIENTED_EDGE('',*,*,#13133,.F.);
#18047=ORIENTED_EDGE('',*,*,#13138,.F.);
#18048=ORIENTED_EDGE('',*,*,#13139,.T.);
#18049=ORIENTED_EDGE('',*,*,#13140,.T.);
#18050=ORIENTED_EDGE('',*,*,#13136,.F.);
#18051=ORIENTED_EDGE('',*,*,#13141,.F.);
#18052=ORIENTED_EDGE('',*,*,#13142,.T.);
#18053=ORIENTED_EDGE('',*,*,#13143,.T.);
#18054=ORIENTED_EDGE('',*,*,#13139,.F.);
#18055=ORIENTED_EDGE('',*,*,#13144,.F.);
#18056=ORIENTED_EDGE('',*,*,#13145,.T.);
#18057=ORIENTED_EDGE('',*,*,#13146,.T.);
#18058=ORIENTED_EDGE('',*,*,#13142,.F.);
#18059=ORIENTED_EDGE('',*,*,#13147,.F.);
#18060=ORIENTED_EDGE('',*,*,#13148,.T.);
#18061=ORIENTED_EDGE('',*,*,#13149,.T.);
#18062=ORIENTED_EDGE('',*,*,#13145,.F.);
#18063=ORIENTED_EDGE('',*,*,#13150,.F.);
#18064=ORIENTED_EDGE('',*,*,#13151,.T.);
#18065=ORIENTED_EDGE('',*,*,#13152,.T.);
#18066=ORIENTED_EDGE('',*,*,#13148,.F.);
#18067=ORIENTED_EDGE('',*,*,#13153,.F.);
#18068=ORIENTED_EDGE('',*,*,#13154,.T.);
#18069=ORIENTED_EDGE('',*,*,#13155,.T.);
#18070=ORIENTED_EDGE('',*,*,#13151,.F.);
#18071=ORIENTED_EDGE('',*,*,#13156,.F.);
#18072=ORIENTED_EDGE('',*,*,#13157,.T.);
#18073=ORIENTED_EDGE('',*,*,#13158,.T.);
#18074=ORIENTED_EDGE('',*,*,#13154,.F.);
#18075=ORIENTED_EDGE('',*,*,#13159,.F.);
#18076=ORIENTED_EDGE('',*,*,#13160,.T.);
#18077=ORIENTED_EDGE('',*,*,#13161,.T.);
#18078=ORIENTED_EDGE('',*,*,#13157,.F.);
#18079=ORIENTED_EDGE('',*,*,#13162,.F.);
#18080=ORIENTED_EDGE('',*,*,#13101,.T.);
#18081=ORIENTED_EDGE('',*,*,#13163,.T.);
#18082=ORIENTED_EDGE('',*,*,#13160,.F.);
#18083=ORIENTED_EDGE('',*,*,#13163,.F.);
#18084=ORIENTED_EDGE('',*,*,#13100,.F.);
#18085=ORIENTED_EDGE('',*,*,#13104,.F.);
#18086=ORIENTED_EDGE('',*,*,#13107,.F.);
#18087=ORIENTED_EDGE('',*,*,#13110,.F.);
#18088=ORIENTED_EDGE('',*,*,#13113,.F.);
#18089=ORIENTED_EDGE('',*,*,#13116,.F.);
#18090=ORIENTED_EDGE('',*,*,#13119,.F.);
#18091=ORIENTED_EDGE('',*,*,#13122,.F.);
#18092=ORIENTED_EDGE('',*,*,#13125,.F.);
#18093=ORIENTED_EDGE('',*,*,#13128,.F.);
#18094=ORIENTED_EDGE('',*,*,#13131,.F.);
#18095=ORIENTED_EDGE('',*,*,#13134,.F.);
#18096=ORIENTED_EDGE('',*,*,#13137,.F.);
#18097=ORIENTED_EDGE('',*,*,#13140,.F.);
#18098=ORIENTED_EDGE('',*,*,#13143,.F.);
#18099=ORIENTED_EDGE('',*,*,#13146,.F.);
#18100=ORIENTED_EDGE('',*,*,#13149,.F.);
#18101=ORIENTED_EDGE('',*,*,#13152,.F.);
#18102=ORIENTED_EDGE('',*,*,#13155,.F.);
#18103=ORIENTED_EDGE('',*,*,#13158,.F.);
#18104=ORIENTED_EDGE('',*,*,#13161,.F.);
#18105=ORIENTED_EDGE('',*,*,#13164,.F.);
#18106=ORIENTED_EDGE('',*,*,#13165,.T.);
#18107=ORIENTED_EDGE('',*,*,#13166,.T.);
#18108=ORIENTED_EDGE('',*,*,#13167,.F.);
#18109=ORIENTED_EDGE('',*,*,#13168,.F.);
#18110=ORIENTED_EDGE('',*,*,#13169,.T.);
#18111=ORIENTED_EDGE('',*,*,#13170,.T.);
#18112=ORIENTED_EDGE('',*,*,#13165,.F.);
#18113=ORIENTED_EDGE('',*,*,#13171,.F.);
#18114=ORIENTED_EDGE('',*,*,#13172,.T.);
#18115=ORIENTED_EDGE('',*,*,#13173,.T.);
#18116=ORIENTED_EDGE('',*,*,#13169,.F.);
#18117=ORIENTED_EDGE('',*,*,#13174,.F.);
#18118=ORIENTED_EDGE('',*,*,#13175,.T.);
#18119=ORIENTED_EDGE('',*,*,#13176,.T.);
#18120=ORIENTED_EDGE('',*,*,#13172,.F.);
#18121=ORIENTED_EDGE('',*,*,#13177,.F.);
#18122=ORIENTED_EDGE('',*,*,#13178,.T.);
#18123=ORIENTED_EDGE('',*,*,#13179,.T.);
#18124=ORIENTED_EDGE('',*,*,#13175,.F.);
#18125=ORIENTED_EDGE('',*,*,#13180,.F.);
#18126=ORIENTED_EDGE('',*,*,#13181,.T.);
#18127=ORIENTED_EDGE('',*,*,#13182,.T.);
#18128=ORIENTED_EDGE('',*,*,#13178,.F.);
#18129=ORIENTED_EDGE('',*,*,#13183,.F.);
#18130=ORIENTED_EDGE('',*,*,#13184,.T.);
#18131=ORIENTED_EDGE('',*,*,#13185,.T.);
#18132=ORIENTED_EDGE('',*,*,#13181,.F.);
#18133=ORIENTED_EDGE('',*,*,#13186,.F.);
#18134=ORIENTED_EDGE('',*,*,#13167,.T.);
#18135=ORIENTED_EDGE('',*,*,#13187,.T.);
#18136=ORIENTED_EDGE('',*,*,#13184,.F.);
#18137=ORIENTED_EDGE('',*,*,#13188,.F.);
#18138=ORIENTED_EDGE('',*,*,#13189,.T.);
#18139=ORIENTED_EDGE('',*,*,#13190,.T.);
#18140=ORIENTED_EDGE('',*,*,#13191,.F.);
#18141=ORIENTED_EDGE('',*,*,#13192,.F.);
#18142=ORIENTED_EDGE('',*,*,#13193,.T.);
#18143=ORIENTED_EDGE('',*,*,#13194,.T.);
#18144=ORIENTED_EDGE('',*,*,#13189,.F.);
#18145=ORIENTED_EDGE('',*,*,#13195,.F.);
#18146=ORIENTED_EDGE('',*,*,#13196,.T.);
#18147=ORIENTED_EDGE('',*,*,#13197,.T.);
#18148=ORIENTED_EDGE('',*,*,#13193,.F.);
#18149=ORIENTED_EDGE('',*,*,#13198,.F.);
#18150=ORIENTED_EDGE('',*,*,#13199,.T.);
#18151=ORIENTED_EDGE('',*,*,#13200,.T.);
#18152=ORIENTED_EDGE('',*,*,#13196,.F.);
#18153=ORIENTED_EDGE('',*,*,#13201,.F.);
#18154=ORIENTED_EDGE('',*,*,#13202,.T.);
#18155=ORIENTED_EDGE('',*,*,#13203,.T.);
#18156=ORIENTED_EDGE('',*,*,#13199,.F.);
#18157=ORIENTED_EDGE('',*,*,#13204,.F.);
#18158=ORIENTED_EDGE('',*,*,#13205,.T.);
#18159=ORIENTED_EDGE('',*,*,#13206,.T.);
#18160=ORIENTED_EDGE('',*,*,#13202,.F.);
#18161=ORIENTED_EDGE('',*,*,#13207,.F.);
#18162=ORIENTED_EDGE('',*,*,#13208,.T.);
#18163=ORIENTED_EDGE('',*,*,#13209,.T.);
#18164=ORIENTED_EDGE('',*,*,#13205,.F.);
#18165=ORIENTED_EDGE('',*,*,#13210,.F.);
#18166=ORIENTED_EDGE('',*,*,#13211,.T.);
#18167=ORIENTED_EDGE('',*,*,#13212,.T.);
#18168=ORIENTED_EDGE('',*,*,#13208,.F.);
#18169=ORIENTED_EDGE('',*,*,#13213,.F.);
#18170=ORIENTED_EDGE('',*,*,#13214,.T.);
#18171=ORIENTED_EDGE('',*,*,#13215,.T.);
#18172=ORIENTED_EDGE('',*,*,#13211,.F.);
#18173=ORIENTED_EDGE('',*,*,#13216,.F.);
#18174=ORIENTED_EDGE('',*,*,#13217,.T.);
#18175=ORIENTED_EDGE('',*,*,#13218,.T.);
#18176=ORIENTED_EDGE('',*,*,#13214,.F.);
#18177=ORIENTED_EDGE('',*,*,#13219,.F.);
#18178=ORIENTED_EDGE('',*,*,#13191,.T.);
#18179=ORIENTED_EDGE('',*,*,#13220,.T.);
#18180=ORIENTED_EDGE('',*,*,#13217,.F.);
#18181=ORIENTED_EDGE('',*,*,#13220,.F.);
#18182=ORIENTED_EDGE('',*,*,#13190,.F.);
#18183=ORIENTED_EDGE('',*,*,#13194,.F.);
#18184=ORIENTED_EDGE('',*,*,#13197,.F.);
#18185=ORIENTED_EDGE('',*,*,#13200,.F.);
#18186=ORIENTED_EDGE('',*,*,#13203,.F.);
#18187=ORIENTED_EDGE('',*,*,#13206,.F.);
#18188=ORIENTED_EDGE('',*,*,#13209,.F.);
#18189=ORIENTED_EDGE('',*,*,#13212,.F.);
#18190=ORIENTED_EDGE('',*,*,#13215,.F.);
#18191=ORIENTED_EDGE('',*,*,#13218,.F.);
#18192=ORIENTED_EDGE('',*,*,#13187,.F.);
#18193=ORIENTED_EDGE('',*,*,#13166,.F.);
#18194=ORIENTED_EDGE('',*,*,#13170,.F.);
#18195=ORIENTED_EDGE('',*,*,#13173,.F.);
#18196=ORIENTED_EDGE('',*,*,#13176,.F.);
#18197=ORIENTED_EDGE('',*,*,#13179,.F.);
#18198=ORIENTED_EDGE('',*,*,#13182,.F.);
#18199=ORIENTED_EDGE('',*,*,#13185,.F.);
#18200=ORIENTED_EDGE('',*,*,#13221,.F.);
#18201=ORIENTED_EDGE('',*,*,#13222,.T.);
#18202=ORIENTED_EDGE('',*,*,#13223,.T.);
#18203=ORIENTED_EDGE('',*,*,#13224,.F.);
#18204=ORIENTED_EDGE('',*,*,#13225,.F.);
#18205=ORIENTED_EDGE('',*,*,#13226,.T.);
#18206=ORIENTED_EDGE('',*,*,#13227,.T.);
#18207=ORIENTED_EDGE('',*,*,#13222,.F.);
#18208=ORIENTED_EDGE('',*,*,#13228,.F.);
#18209=ORIENTED_EDGE('',*,*,#13229,.T.);
#18210=ORIENTED_EDGE('',*,*,#13230,.T.);
#18211=ORIENTED_EDGE('',*,*,#13226,.F.);
#18212=ORIENTED_EDGE('',*,*,#13231,.F.);
#18213=ORIENTED_EDGE('',*,*,#13232,.T.);
#18214=ORIENTED_EDGE('',*,*,#13233,.T.);
#18215=ORIENTED_EDGE('',*,*,#13229,.F.);
#18216=ORIENTED_EDGE('',*,*,#13234,.F.);
#18217=ORIENTED_EDGE('',*,*,#13235,.T.);
#18218=ORIENTED_EDGE('',*,*,#13236,.T.);
#18219=ORIENTED_EDGE('',*,*,#13232,.F.);
#18220=ORIENTED_EDGE('',*,*,#13237,.F.);
#18221=ORIENTED_EDGE('',*,*,#13238,.T.);
#18222=ORIENTED_EDGE('',*,*,#13239,.T.);
#18223=ORIENTED_EDGE('',*,*,#13235,.F.);
#18224=ORIENTED_EDGE('',*,*,#13240,.F.);
#18225=ORIENTED_EDGE('',*,*,#13241,.T.);
#18226=ORIENTED_EDGE('',*,*,#13242,.T.);
#18227=ORIENTED_EDGE('',*,*,#13238,.F.);
#18228=ORIENTED_EDGE('',*,*,#13243,.F.);
#18229=ORIENTED_EDGE('',*,*,#13244,.T.);
#18230=ORIENTED_EDGE('',*,*,#13245,.T.);
#18231=ORIENTED_EDGE('',*,*,#13241,.F.);
#18232=ORIENTED_EDGE('',*,*,#13246,.F.);
#18233=ORIENTED_EDGE('',*,*,#13224,.T.);
#18234=ORIENTED_EDGE('',*,*,#13247,.T.);
#18235=ORIENTED_EDGE('',*,*,#13244,.F.);
#18236=ORIENTED_EDGE('',*,*,#13248,.F.);
#18237=ORIENTED_EDGE('',*,*,#13249,.T.);
#18238=ORIENTED_EDGE('',*,*,#13250,.T.);
#18239=ORIENTED_EDGE('',*,*,#13251,.F.);
#18240=ORIENTED_EDGE('',*,*,#13252,.F.);
#18241=ORIENTED_EDGE('',*,*,#13253,.T.);
#18242=ORIENTED_EDGE('',*,*,#13254,.T.);
#18243=ORIENTED_EDGE('',*,*,#13249,.F.);
#18244=ORIENTED_EDGE('',*,*,#13255,.F.);
#18245=ORIENTED_EDGE('',*,*,#13256,.T.);
#18246=ORIENTED_EDGE('',*,*,#13257,.T.);
#18247=ORIENTED_EDGE('',*,*,#13253,.F.);
#18248=ORIENTED_EDGE('',*,*,#13258,.F.);
#18249=ORIENTED_EDGE('',*,*,#13259,.T.);
#18250=ORIENTED_EDGE('',*,*,#13260,.T.);
#18251=ORIENTED_EDGE('',*,*,#13256,.F.);
#18252=ORIENTED_EDGE('',*,*,#13261,.F.);
#18253=ORIENTED_EDGE('',*,*,#13262,.T.);
#18254=ORIENTED_EDGE('',*,*,#13263,.T.);
#18255=ORIENTED_EDGE('',*,*,#13259,.F.);
#18256=ORIENTED_EDGE('',*,*,#13264,.F.);
#18257=ORIENTED_EDGE('',*,*,#13265,.T.);
#18258=ORIENTED_EDGE('',*,*,#13266,.T.);
#18259=ORIENTED_EDGE('',*,*,#13262,.F.);
#18260=ORIENTED_EDGE('',*,*,#13267,.F.);
#18261=ORIENTED_EDGE('',*,*,#13268,.T.);
#18262=ORIENTED_EDGE('',*,*,#13269,.T.);
#18263=ORIENTED_EDGE('',*,*,#13265,.F.);
#18264=ORIENTED_EDGE('',*,*,#13270,.F.);
#18265=ORIENTED_EDGE('',*,*,#13271,.T.);
#18266=ORIENTED_EDGE('',*,*,#13272,.T.);
#18267=ORIENTED_EDGE('',*,*,#13268,.F.);
#18268=ORIENTED_EDGE('',*,*,#13273,.F.);
#18269=ORIENTED_EDGE('',*,*,#13274,.T.);
#18270=ORIENTED_EDGE('',*,*,#13275,.T.);
#18271=ORIENTED_EDGE('',*,*,#13271,.F.);
#18272=ORIENTED_EDGE('',*,*,#13276,.F.);
#18273=ORIENTED_EDGE('',*,*,#13277,.T.);
#18274=ORIENTED_EDGE('',*,*,#13278,.T.);
#18275=ORIENTED_EDGE('',*,*,#13274,.F.);
#18276=ORIENTED_EDGE('',*,*,#13279,.F.);
#18277=ORIENTED_EDGE('',*,*,#13280,.T.);
#18278=ORIENTED_EDGE('',*,*,#13281,.T.);
#18279=ORIENTED_EDGE('',*,*,#13277,.F.);
#18280=ORIENTED_EDGE('',*,*,#13282,.F.);
#18281=ORIENTED_EDGE('',*,*,#13283,.T.);
#18282=ORIENTED_EDGE('',*,*,#13284,.T.);
#18283=ORIENTED_EDGE('',*,*,#13280,.F.);
#18284=ORIENTED_EDGE('',*,*,#13285,.F.);
#18285=ORIENTED_EDGE('',*,*,#13286,.T.);
#18286=ORIENTED_EDGE('',*,*,#13287,.T.);
#18287=ORIENTED_EDGE('',*,*,#13283,.F.);
#18288=ORIENTED_EDGE('',*,*,#13288,.F.);
#18289=ORIENTED_EDGE('',*,*,#13289,.T.);
#18290=ORIENTED_EDGE('',*,*,#13290,.T.);
#18291=ORIENTED_EDGE('',*,*,#13286,.F.);
#18292=ORIENTED_EDGE('',*,*,#13291,.F.);
#18293=ORIENTED_EDGE('',*,*,#13292,.T.);
#18294=ORIENTED_EDGE('',*,*,#13293,.T.);
#18295=ORIENTED_EDGE('',*,*,#13289,.F.);
#18296=ORIENTED_EDGE('',*,*,#13294,.F.);
#18297=ORIENTED_EDGE('',*,*,#13295,.T.);
#18298=ORIENTED_EDGE('',*,*,#13296,.T.);
#18299=ORIENTED_EDGE('',*,*,#13292,.F.);
#18300=ORIENTED_EDGE('',*,*,#13297,.F.);
#18301=ORIENTED_EDGE('',*,*,#13298,.T.);
#18302=ORIENTED_EDGE('',*,*,#13299,.T.);
#18303=ORIENTED_EDGE('',*,*,#13295,.F.);
#18304=ORIENTED_EDGE('',*,*,#13300,.F.);
#18305=ORIENTED_EDGE('',*,*,#13301,.T.);
#18306=ORIENTED_EDGE('',*,*,#13302,.T.);
#18307=ORIENTED_EDGE('',*,*,#13298,.F.);
#18308=ORIENTED_EDGE('',*,*,#13303,.F.);
#18309=ORIENTED_EDGE('',*,*,#13251,.T.);
#18310=ORIENTED_EDGE('',*,*,#13304,.T.);
#18311=ORIENTED_EDGE('',*,*,#13301,.F.);
#18312=ORIENTED_EDGE('',*,*,#13304,.F.);
#18313=ORIENTED_EDGE('',*,*,#13250,.F.);
#18314=ORIENTED_EDGE('',*,*,#13254,.F.);
#18315=ORIENTED_EDGE('',*,*,#13257,.F.);
#18316=ORIENTED_EDGE('',*,*,#13260,.F.);
#18317=ORIENTED_EDGE('',*,*,#13263,.F.);
#18318=ORIENTED_EDGE('',*,*,#13266,.F.);
#18319=ORIENTED_EDGE('',*,*,#13269,.F.);
#18320=ORIENTED_EDGE('',*,*,#13272,.F.);
#18321=ORIENTED_EDGE('',*,*,#13275,.F.);
#18322=ORIENTED_EDGE('',*,*,#13278,.F.);
#18323=ORIENTED_EDGE('',*,*,#13281,.F.);
#18324=ORIENTED_EDGE('',*,*,#13284,.F.);
#18325=ORIENTED_EDGE('',*,*,#13287,.F.);
#18326=ORIENTED_EDGE('',*,*,#13290,.F.);
#18327=ORIENTED_EDGE('',*,*,#13293,.F.);
#18328=ORIENTED_EDGE('',*,*,#13296,.F.);
#18329=ORIENTED_EDGE('',*,*,#13299,.F.);
#18330=ORIENTED_EDGE('',*,*,#13302,.F.);
#18331=ORIENTED_EDGE('',*,*,#13247,.F.);
#18332=ORIENTED_EDGE('',*,*,#13223,.F.);
#18333=ORIENTED_EDGE('',*,*,#13227,.F.);
#18334=ORIENTED_EDGE('',*,*,#13230,.F.);
#18335=ORIENTED_EDGE('',*,*,#13233,.F.);
#18336=ORIENTED_EDGE('',*,*,#13236,.F.);
#18337=ORIENTED_EDGE('',*,*,#13239,.F.);
#18338=ORIENTED_EDGE('',*,*,#13242,.F.);
#18339=ORIENTED_EDGE('',*,*,#13245,.F.);
#18340=ORIENTED_EDGE('',*,*,#13305,.F.);
#18341=ORIENTED_EDGE('',*,*,#13306,.T.);
#18342=ORIENTED_EDGE('',*,*,#13307,.T.);
#18343=ORIENTED_EDGE('',*,*,#13308,.F.);
#18344=ORIENTED_EDGE('',*,*,#13309,.F.);
#18345=ORIENTED_EDGE('',*,*,#13310,.T.);
#18346=ORIENTED_EDGE('',*,*,#13311,.T.);
#18347=ORIENTED_EDGE('',*,*,#13306,.F.);
#18348=ORIENTED_EDGE('',*,*,#13312,.F.);
#18349=ORIENTED_EDGE('',*,*,#13313,.T.);
#18350=ORIENTED_EDGE('',*,*,#13314,.T.);
#18351=ORIENTED_EDGE('',*,*,#13310,.F.);
#18352=ORIENTED_EDGE('',*,*,#13315,.F.);
#18353=ORIENTED_EDGE('',*,*,#13316,.T.);
#18354=ORIENTED_EDGE('',*,*,#13317,.T.);
#18355=ORIENTED_EDGE('',*,*,#13313,.F.);
#18356=ORIENTED_EDGE('',*,*,#13318,.F.);
#18357=ORIENTED_EDGE('',*,*,#13319,.T.);
#18358=ORIENTED_EDGE('',*,*,#13320,.T.);
#18359=ORIENTED_EDGE('',*,*,#13316,.F.);
#18360=ORIENTED_EDGE('',*,*,#13321,.F.);
#18361=ORIENTED_EDGE('',*,*,#13322,.T.);
#18362=ORIENTED_EDGE('',*,*,#13323,.T.);
#18363=ORIENTED_EDGE('',*,*,#13319,.F.);
#18364=ORIENTED_EDGE('',*,*,#13324,.F.);
#18365=ORIENTED_EDGE('',*,*,#13325,.T.);
#18366=ORIENTED_EDGE('',*,*,#13326,.T.);
#18367=ORIENTED_EDGE('',*,*,#13322,.F.);
#18368=ORIENTED_EDGE('',*,*,#13327,.F.);
#18369=ORIENTED_EDGE('',*,*,#13308,.T.);
#18370=ORIENTED_EDGE('',*,*,#13328,.T.);
#18371=ORIENTED_EDGE('',*,*,#13325,.F.);
#18372=ORIENTED_EDGE('',*,*,#13329,.F.);
#18373=ORIENTED_EDGE('',*,*,#13330,.T.);
#18374=ORIENTED_EDGE('',*,*,#13331,.T.);
#18375=ORIENTED_EDGE('',*,*,#13332,.F.);
#18376=ORIENTED_EDGE('',*,*,#13333,.F.);
#18377=ORIENTED_EDGE('',*,*,#13334,.T.);
#18378=ORIENTED_EDGE('',*,*,#13335,.T.);
#18379=ORIENTED_EDGE('',*,*,#13330,.F.);
#18380=ORIENTED_EDGE('',*,*,#13336,.F.);
#18381=ORIENTED_EDGE('',*,*,#13337,.T.);
#18382=ORIENTED_EDGE('',*,*,#13338,.T.);
#18383=ORIENTED_EDGE('',*,*,#13334,.F.);
#18384=ORIENTED_EDGE('',*,*,#13339,.F.);
#18385=ORIENTED_EDGE('',*,*,#13340,.T.);
#18386=ORIENTED_EDGE('',*,*,#13341,.T.);
#18387=ORIENTED_EDGE('',*,*,#13337,.F.);
#18388=ORIENTED_EDGE('',*,*,#13342,.F.);
#18389=ORIENTED_EDGE('',*,*,#13343,.T.);
#18390=ORIENTED_EDGE('',*,*,#13344,.T.);
#18391=ORIENTED_EDGE('',*,*,#13340,.F.);
#18392=ORIENTED_EDGE('',*,*,#13345,.F.);
#18393=ORIENTED_EDGE('',*,*,#13346,.T.);
#18394=ORIENTED_EDGE('',*,*,#13347,.T.);
#18395=ORIENTED_EDGE('',*,*,#13343,.F.);
#18396=ORIENTED_EDGE('',*,*,#13348,.F.);
#18397=ORIENTED_EDGE('',*,*,#13349,.T.);
#18398=ORIENTED_EDGE('',*,*,#13350,.T.);
#18399=ORIENTED_EDGE('',*,*,#13346,.F.);
#18400=ORIENTED_EDGE('',*,*,#13351,.F.);
#18401=ORIENTED_EDGE('',*,*,#13352,.T.);
#18402=ORIENTED_EDGE('',*,*,#13353,.T.);
#18403=ORIENTED_EDGE('',*,*,#13349,.F.);
#18404=ORIENTED_EDGE('',*,*,#13354,.F.);
#18405=ORIENTED_EDGE('',*,*,#13355,.T.);
#18406=ORIENTED_EDGE('',*,*,#13356,.T.);
#18407=ORIENTED_EDGE('',*,*,#13352,.F.);
#18408=ORIENTED_EDGE('',*,*,#13357,.F.);
#18409=ORIENTED_EDGE('',*,*,#13358,.T.);
#18410=ORIENTED_EDGE('',*,*,#13359,.T.);
#18411=ORIENTED_EDGE('',*,*,#13355,.F.);
#18412=ORIENTED_EDGE('',*,*,#13360,.F.);
#18413=ORIENTED_EDGE('',*,*,#13361,.T.);
#18414=ORIENTED_EDGE('',*,*,#13362,.T.);
#18415=ORIENTED_EDGE('',*,*,#13358,.F.);
#18416=ORIENTED_EDGE('',*,*,#13363,.F.);
#18417=ORIENTED_EDGE('',*,*,#13364,.T.);
#18418=ORIENTED_EDGE('',*,*,#13365,.T.);
#18419=ORIENTED_EDGE('',*,*,#13361,.F.);
#18420=ORIENTED_EDGE('',*,*,#13366,.F.);
#18421=ORIENTED_EDGE('',*,*,#13332,.T.);
#18422=ORIENTED_EDGE('',*,*,#13367,.T.);
#18423=ORIENTED_EDGE('',*,*,#13364,.F.);
#18424=ORIENTED_EDGE('',*,*,#13367,.F.);
#18425=ORIENTED_EDGE('',*,*,#13331,.F.);
#18426=ORIENTED_EDGE('',*,*,#13335,.F.);
#18427=ORIENTED_EDGE('',*,*,#13338,.F.);
#18428=ORIENTED_EDGE('',*,*,#13341,.F.);
#18429=ORIENTED_EDGE('',*,*,#13344,.F.);
#18430=ORIENTED_EDGE('',*,*,#13347,.F.);
#18431=ORIENTED_EDGE('',*,*,#13350,.F.);
#18432=ORIENTED_EDGE('',*,*,#13353,.F.);
#18433=ORIENTED_EDGE('',*,*,#13356,.F.);
#18434=ORIENTED_EDGE('',*,*,#13359,.F.);
#18435=ORIENTED_EDGE('',*,*,#13362,.F.);
#18436=ORIENTED_EDGE('',*,*,#13365,.F.);
#18437=ORIENTED_EDGE('',*,*,#13328,.F.);
#18438=ORIENTED_EDGE('',*,*,#13307,.F.);
#18439=ORIENTED_EDGE('',*,*,#13311,.F.);
#18440=ORIENTED_EDGE('',*,*,#13314,.F.);
#18441=ORIENTED_EDGE('',*,*,#13317,.F.);
#18442=ORIENTED_EDGE('',*,*,#13320,.F.);
#18443=ORIENTED_EDGE('',*,*,#13323,.F.);
#18444=ORIENTED_EDGE('',*,*,#13326,.F.);
#18445=ORIENTED_EDGE('',*,*,#13368,.F.);
#18446=ORIENTED_EDGE('',*,*,#13369,.T.);
#18447=ORIENTED_EDGE('',*,*,#13370,.T.);
#18448=ORIENTED_EDGE('',*,*,#13371,.F.);
#18449=ORIENTED_EDGE('',*,*,#13372,.F.);
#18450=ORIENTED_EDGE('',*,*,#13373,.T.);
#18451=ORIENTED_EDGE('',*,*,#13374,.T.);
#18452=ORIENTED_EDGE('',*,*,#13369,.F.);
#18453=ORIENTED_EDGE('',*,*,#13375,.F.);
#18454=ORIENTED_EDGE('',*,*,#13376,.T.);
#18455=ORIENTED_EDGE('',*,*,#13377,.T.);
#18456=ORIENTED_EDGE('',*,*,#13373,.F.);
#18457=ORIENTED_EDGE('',*,*,#13378,.F.);
#18458=ORIENTED_EDGE('',*,*,#13379,.T.);
#18459=ORIENTED_EDGE('',*,*,#13380,.T.);
#18460=ORIENTED_EDGE('',*,*,#13376,.F.);
#18461=ORIENTED_EDGE('',*,*,#13381,.F.);
#18462=ORIENTED_EDGE('',*,*,#13382,.T.);
#18463=ORIENTED_EDGE('',*,*,#13383,.T.);
#18464=ORIENTED_EDGE('',*,*,#13379,.F.);
#18465=ORIENTED_EDGE('',*,*,#13384,.F.);
#18466=ORIENTED_EDGE('',*,*,#13385,.T.);
#18467=ORIENTED_EDGE('',*,*,#13386,.T.);
#18468=ORIENTED_EDGE('',*,*,#13382,.F.);
#18469=ORIENTED_EDGE('',*,*,#13387,.F.);
#18470=ORIENTED_EDGE('',*,*,#13388,.T.);
#18471=ORIENTED_EDGE('',*,*,#13389,.T.);
#18472=ORIENTED_EDGE('',*,*,#13385,.F.);
#18473=ORIENTED_EDGE('',*,*,#13390,.F.);
#18474=ORIENTED_EDGE('',*,*,#13391,.T.);
#18475=ORIENTED_EDGE('',*,*,#13392,.T.);
#18476=ORIENTED_EDGE('',*,*,#13388,.F.);
#18477=ORIENTED_EDGE('',*,*,#13393,.F.);
#18478=ORIENTED_EDGE('',*,*,#13394,.T.);
#18479=ORIENTED_EDGE('',*,*,#13395,.T.);
#18480=ORIENTED_EDGE('',*,*,#13391,.F.);
#18481=ORIENTED_EDGE('',*,*,#13396,.F.);
#18482=ORIENTED_EDGE('',*,*,#13397,.T.);
#18483=ORIENTED_EDGE('',*,*,#13398,.T.);
#18484=ORIENTED_EDGE('',*,*,#13394,.F.);
#18485=ORIENTED_EDGE('',*,*,#13399,.F.);
#18486=ORIENTED_EDGE('',*,*,#13400,.T.);
#18487=ORIENTED_EDGE('',*,*,#13401,.T.);
#18488=ORIENTED_EDGE('',*,*,#13397,.F.);
#18489=ORIENTED_EDGE('',*,*,#13402,.F.);
#18490=ORIENTED_EDGE('',*,*,#13403,.T.);
#18491=ORIENTED_EDGE('',*,*,#13404,.T.);
#18492=ORIENTED_EDGE('',*,*,#13400,.F.);
#18493=ORIENTED_EDGE('',*,*,#13405,.F.);
#18494=ORIENTED_EDGE('',*,*,#13371,.T.);
#18495=ORIENTED_EDGE('',*,*,#13406,.T.);
#18496=ORIENTED_EDGE('',*,*,#13403,.F.);
#18497=ORIENTED_EDGE('',*,*,#13406,.F.);
#18498=ORIENTED_EDGE('',*,*,#13370,.F.);
#18499=ORIENTED_EDGE('',*,*,#13374,.F.);
#18500=ORIENTED_EDGE('',*,*,#13377,.F.);
#18501=ORIENTED_EDGE('',*,*,#13380,.F.);
#18502=ORIENTED_EDGE('',*,*,#13383,.F.);
#18503=ORIENTED_EDGE('',*,*,#13386,.F.);
#18504=ORIENTED_EDGE('',*,*,#13389,.F.);
#18505=ORIENTED_EDGE('',*,*,#13392,.F.);
#18506=ORIENTED_EDGE('',*,*,#13395,.F.);
#18507=ORIENTED_EDGE('',*,*,#13398,.F.);
#18508=ORIENTED_EDGE('',*,*,#13401,.F.);
#18509=ORIENTED_EDGE('',*,*,#13404,.F.);
#18510=ORIENTED_EDGE('',*,*,#13305,.T.);
#18511=ORIENTED_EDGE('',*,*,#13327,.T.);
#18512=ORIENTED_EDGE('',*,*,#13324,.T.);
#18513=ORIENTED_EDGE('',*,*,#13321,.T.);
#18514=ORIENTED_EDGE('',*,*,#13318,.T.);
#18515=ORIENTED_EDGE('',*,*,#13315,.T.);
#18516=ORIENTED_EDGE('',*,*,#13312,.T.);
#18517=ORIENTED_EDGE('',*,*,#13309,.T.);
#18518=ORIENTED_EDGE('',*,*,#13221,.T.);
#18519=ORIENTED_EDGE('',*,*,#13246,.T.);
#18520=ORIENTED_EDGE('',*,*,#13243,.T.);
#18521=ORIENTED_EDGE('',*,*,#13240,.T.);
#18522=ORIENTED_EDGE('',*,*,#13237,.T.);
#18523=ORIENTED_EDGE('',*,*,#13234,.T.);
#18524=ORIENTED_EDGE('',*,*,#13231,.T.);
#18525=ORIENTED_EDGE('',*,*,#13228,.T.);
#18526=ORIENTED_EDGE('',*,*,#13225,.T.);
#18527=ORIENTED_EDGE('',*,*,#13164,.T.);
#18528=ORIENTED_EDGE('',*,*,#13186,.T.);
#18529=ORIENTED_EDGE('',*,*,#13183,.T.);
#18530=ORIENTED_EDGE('',*,*,#13180,.T.);
#18531=ORIENTED_EDGE('',*,*,#13177,.T.);
#18532=ORIENTED_EDGE('',*,*,#13174,.T.);
#18533=ORIENTED_EDGE('',*,*,#13171,.T.);
#18534=ORIENTED_EDGE('',*,*,#13168,.T.);
#18535=ORIENTED_EDGE('',*,*,#12864,.T.);
#18536=ORIENTED_EDGE('',*,*,#12877,.T.);
#18537=ORIENTED_EDGE('',*,*,#12874,.T.);
#18538=ORIENTED_EDGE('',*,*,#12871,.T.);
#18539=ORIENTED_EDGE('',*,*,#12868,.T.);
#18540=ORIENTED_EDGE('',*,*,#12630,.T.);
#18541=ORIENTED_EDGE('',*,*,#12652,.T.);
#18542=ORIENTED_EDGE('',*,*,#12649,.T.);
#18543=ORIENTED_EDGE('',*,*,#12646,.T.);
#18544=ORIENTED_EDGE('',*,*,#12643,.T.);
#18545=ORIENTED_EDGE('',*,*,#12640,.T.);
#18546=ORIENTED_EDGE('',*,*,#12637,.T.);
#18547=ORIENTED_EDGE('',*,*,#12634,.T.);
#18548=ORIENTED_EDGE('',*,*,#12519,.T.);
#18549=ORIENTED_EDGE('',*,*,#12547,.T.);
#18550=ORIENTED_EDGE('',*,*,#12544,.T.);
#18551=ORIENTED_EDGE('',*,*,#12541,.T.);
#18552=ORIENTED_EDGE('',*,*,#12538,.T.);
#18553=ORIENTED_EDGE('',*,*,#12535,.T.);
#18554=ORIENTED_EDGE('',*,*,#12532,.T.);
#18555=ORIENTED_EDGE('',*,*,#12529,.T.);
#18556=ORIENTED_EDGE('',*,*,#12526,.T.);
#18557=ORIENTED_EDGE('',*,*,#12523,.T.);
#18558=ORIENTED_EDGE('',*,*,#13407,.F.);
#18559=ORIENTED_EDGE('',*,*,#13408,.T.);
#18560=ORIENTED_EDGE('',*,*,#13409,.F.);
#18561=ORIENTED_EDGE('',*,*,#13410,.F.);
#18562=ORIENTED_EDGE('',*,*,#13411,.F.);
#18563=ORIENTED_EDGE('',*,*,#13412,.F.);
#18564=ORIENTED_EDGE('',*,*,#13408,.F.);
#18565=ORIENTED_EDGE('',*,*,#13413,.T.);
#18566=ORIENTED_EDGE('',*,*,#13414,.T.);
#18567=ORIENTED_EDGE('',*,*,#13415,.T.);
#18568=ORIENTED_EDGE('',*,*,#13414,.F.);
#18569=ORIENTED_EDGE('',*,*,#13416,.F.);
#18570=ORIENTED_EDGE('',*,*,#13417,.T.);
#18571=ORIENTED_EDGE('',*,*,#13415,.F.);
#18572=ORIENTED_EDGE('',*,*,#13417,.F.);
#18573=ORIENTED_EDGE('',*,*,#13418,.F.);
#18574=ORIENTED_EDGE('',*,*,#13419,.F.);
#18575=ORIENTED_EDGE('',*,*,#13420,.F.);
#18576=ORIENTED_EDGE('',*,*,#13421,.F.);
#18577=ORIENTED_EDGE('',*,*,#13413,.F.);
#18578=ORIENTED_EDGE('',*,*,#13422,.T.);
#18579=ORIENTED_EDGE('',*,*,#13423,.T.);
#18580=ORIENTED_EDGE('',*,*,#13422,.F.);
#18581=ORIENTED_EDGE('',*,*,#13423,.F.);
#18582=ORIENTED_EDGE('',*,*,#13424,.T.);
#18583=ORIENTED_EDGE('',*,*,#13409,.T.);
#18584=ORIENTED_EDGE('',*,*,#13412,.T.);
#18585=ORIENTED_EDGE('',*,*,#13425,.T.);
#18586=ORIENTED_EDGE('',*,*,#13426,.T.);
#18587=ORIENTED_EDGE('',*,*,#13425,.F.);
#18588=ORIENTED_EDGE('',*,*,#13411,.T.);
#18589=ORIENTED_EDGE('',*,*,#13410,.T.);
#18590=ORIENTED_EDGE('',*,*,#13424,.F.);
#18591=ORIENTED_EDGE('',*,*,#13416,.T.);
#18592=ORIENTED_EDGE('',*,*,#13426,.F.);
#18593=ORIENTED_EDGE('',*,*,#13427,.F.);
#18594=ORIENTED_EDGE('',*,*,#13421,.T.);
#18595=ORIENTED_EDGE('',*,*,#13418,.T.);
#18596=ORIENTED_EDGE('',*,*,#13427,.T.);
#18597=ORIENTED_EDGE('',*,*,#13420,.T.);
#18598=ORIENTED_EDGE('',*,*,#13428,.F.);
#18599=ORIENTED_EDGE('',*,*,#13429,.T.);
#18600=ORIENTED_EDGE('',*,*,#13430,.T.);
#18601=ORIENTED_EDGE('',*,*,#13429,.F.);
#18602=ORIENTED_EDGE('',*,*,#13431,.F.);
#18603=ORIENTED_EDGE('',*,*,#13432,.T.);
#18604=ORIENTED_EDGE('',*,*,#13433,.T.);
#18605=ORIENTED_EDGE('',*,*,#13428,.T.);
#18606=ORIENTED_EDGE('',*,*,#13419,.T.);
#18607=ORIENTED_EDGE('',*,*,#13431,.T.);
#18608=ORIENTED_EDGE('',*,*,#13433,.F.);
#18609=ORIENTED_EDGE('',*,*,#13434,.T.);
#18610=ORIENTED_EDGE('',*,*,#13435,.T.);
#18611=ORIENTED_EDGE('',*,*,#13436,.T.);
#18612=ORIENTED_EDGE('',*,*,#13435,.F.);
#18613=ORIENTED_EDGE('',*,*,#13437,.F.);
#18614=ORIENTED_EDGE('',*,*,#13434,.F.);
#18615=ORIENTED_EDGE('',*,*,#13438,.F.);
#18616=ORIENTED_EDGE('',*,*,#13439,.F.);
#18617=ORIENTED_EDGE('',*,*,#13440,.F.);
#18618=ORIENTED_EDGE('',*,*,#13441,.F.);
#18619=ORIENTED_EDGE('',*,*,#13442,.F.);
#18620=ORIENTED_EDGE('',*,*,#13443,.F.);
#18621=ORIENTED_EDGE('',*,*,#13407,.T.);
#18622=ORIENTED_EDGE('',*,*,#13436,.F.);
#18623=ORIENTED_EDGE('',*,*,#13444,.T.);
#18624=ORIENTED_EDGE('',*,*,#13445,.T.);
#18625=ORIENTED_EDGE('',*,*,#13444,.F.);
#18626=ORIENTED_EDGE('',*,*,#13443,.T.);
#18627=ORIENTED_EDGE('',*,*,#13446,.T.);
#18628=ORIENTED_EDGE('',*,*,#13447,.T.);
#18629=ORIENTED_EDGE('',*,*,#13446,.F.);
#18630=ORIENTED_EDGE('',*,*,#13447,.F.);
#18631=ORIENTED_EDGE('',*,*,#13448,.T.);
#18632=ORIENTED_EDGE('',*,*,#13449,.T.);
#18633=ORIENTED_EDGE('',*,*,#13448,.F.);
#18634=ORIENTED_EDGE('',*,*,#13438,.T.);
#18635=ORIENTED_EDGE('',*,*,#13450,.T.);
#18636=ORIENTED_EDGE('',*,*,#13451,.T.);
#18637=ORIENTED_EDGE('',*,*,#13450,.F.);
#18638=ORIENTED_EDGE('',*,*,#13451,.F.);
#18639=ORIENTED_EDGE('',*,*,#13452,.T.);
#18640=ORIENTED_EDGE('',*,*,#13453,.T.);
#18641=ORIENTED_EDGE('',*,*,#13452,.F.);
#18642=ORIENTED_EDGE('',*,*,#13442,.T.);
#18643=ORIENTED_EDGE('',*,*,#13454,.T.);
#18644=ORIENTED_EDGE('',*,*,#13455,.T.);
#18645=ORIENTED_EDGE('',*,*,#13454,.F.);
#18646=ORIENTED_EDGE('',*,*,#13455,.F.);
#18647=ORIENTED_EDGE('',*,*,#13456,.T.);
#18648=ORIENTED_EDGE('',*,*,#13457,.T.);
#18649=ORIENTED_EDGE('',*,*,#13456,.F.);
#18650=ORIENTED_EDGE('',*,*,#13439,.T.);
#18651=ORIENTED_EDGE('',*,*,#13458,.T.);
#18652=ORIENTED_EDGE('',*,*,#13459,.T.);
#18653=ORIENTED_EDGE('',*,*,#13458,.F.);
#18654=ORIENTED_EDGE('',*,*,#13459,.F.);
#18655=ORIENTED_EDGE('',*,*,#13460,.T.);
#18656=ORIENTED_EDGE('',*,*,#13461,.T.);
#18657=ORIENTED_EDGE('',*,*,#13460,.F.);
#18658=ORIENTED_EDGE('',*,*,#13441,.T.);
#18659=ORIENTED_EDGE('',*,*,#13462,.T.);
#18660=ORIENTED_EDGE('',*,*,#13463,.T.);
#18661=ORIENTED_EDGE('',*,*,#13462,.F.);
#18662=ORIENTED_EDGE('',*,*,#13463,.F.);
#18663=ORIENTED_EDGE('',*,*,#13464,.T.);
#18664=ORIENTED_EDGE('',*,*,#13465,.T.);
#18665=ORIENTED_EDGE('',*,*,#13464,.F.);
#18666=ORIENTED_EDGE('',*,*,#13465,.F.);
#18667=ORIENTED_EDGE('',*,*,#13466,.T.);
#18668=ORIENTED_EDGE('',*,*,#13466,.F.);
#18669=ORIENTED_EDGE('',*,*,#13461,.F.);
#18670=ORIENTED_EDGE('',*,*,#13467,.T.);
#18671=ORIENTED_EDGE('',*,*,#13467,.F.);
#18672=ORIENTED_EDGE('',*,*,#13457,.F.);
#18673=ORIENTED_EDGE('',*,*,#13468,.T.);
#18674=ORIENTED_EDGE('',*,*,#13468,.F.);
#18675=ORIENTED_EDGE('',*,*,#13453,.F.);
#18676=ORIENTED_EDGE('',*,*,#13469,.T.);
#18677=ORIENTED_EDGE('',*,*,#13469,.F.);
#18678=ORIENTED_EDGE('',*,*,#13449,.F.);
#18679=ORIENTED_EDGE('',*,*,#13470,.T.);
#18680=ORIENTED_EDGE('',*,*,#13470,.F.);
#18681=ORIENTED_EDGE('',*,*,#13445,.F.);
#18682=ORIENTED_EDGE('',*,*,#13471,.T.);
#18683=ORIENTED_EDGE('',*,*,#13471,.F.);
#18684=ORIENTED_EDGE('',*,*,#13440,.T.);
#18685=ORIENTED_EDGE('',*,*,#13472,.T.);
#18686=ORIENTED_EDGE('',*,*,#13473,.T.);
#18687=ORIENTED_EDGE('',*,*,#13474,.T.);
#18688=ORIENTED_EDGE('',*,*,#13472,.F.);
#18689=ORIENTED_EDGE('',*,*,#13475,.T.);
#18690=ORIENTED_EDGE('',*,*,#13476,.T.);
#18691=ORIENTED_EDGE('',*,*,#13473,.F.);
#18692=ORIENTED_EDGE('',*,*,#13474,.F.);
#18693=ORIENTED_EDGE('',*,*,#13476,.F.);
#18694=ORIENTED_EDGE('',*,*,#13432,.F.);
#18695=ORIENTED_EDGE('',*,*,#13368,.T.);
#18696=ORIENTED_EDGE('',*,*,#13405,.T.);
#18697=ORIENTED_EDGE('',*,*,#13402,.T.);
#18698=ORIENTED_EDGE('',*,*,#13399,.T.);
#18699=ORIENTED_EDGE('',*,*,#13396,.T.);
#18700=ORIENTED_EDGE('',*,*,#13393,.T.);
#18701=ORIENTED_EDGE('',*,*,#13390,.T.);
#18702=ORIENTED_EDGE('',*,*,#13387,.T.);
#18703=ORIENTED_EDGE('',*,*,#13384,.T.);
#18704=ORIENTED_EDGE('',*,*,#13381,.T.);
#18705=ORIENTED_EDGE('',*,*,#13378,.T.);
#18706=ORIENTED_EDGE('',*,*,#13375,.T.);
#18707=ORIENTED_EDGE('',*,*,#13372,.T.);
#18708=ORIENTED_EDGE('',*,*,#13329,.T.);
#18709=ORIENTED_EDGE('',*,*,#13366,.T.);
#18710=ORIENTED_EDGE('',*,*,#13363,.T.);
#18711=ORIENTED_EDGE('',*,*,#13360,.T.);
#18712=ORIENTED_EDGE('',*,*,#13357,.T.);
#18713=ORIENTED_EDGE('',*,*,#13354,.T.);
#18714=ORIENTED_EDGE('',*,*,#13351,.T.);
#18715=ORIENTED_EDGE('',*,*,#13348,.T.);
#18716=ORIENTED_EDGE('',*,*,#13345,.T.);
#18717=ORIENTED_EDGE('',*,*,#13342,.T.);
#18718=ORIENTED_EDGE('',*,*,#13339,.T.);
#18719=ORIENTED_EDGE('',*,*,#13336,.T.);
#18720=ORIENTED_EDGE('',*,*,#13333,.T.);
#18721=ORIENTED_EDGE('',*,*,#13248,.T.);
#18722=ORIENTED_EDGE('',*,*,#13303,.T.);
#18723=ORIENTED_EDGE('',*,*,#13300,.T.);
#18724=ORIENTED_EDGE('',*,*,#13297,.T.);
#18725=ORIENTED_EDGE('',*,*,#13294,.T.);
#18726=ORIENTED_EDGE('',*,*,#13291,.T.);
#18727=ORIENTED_EDGE('',*,*,#13288,.T.);
#18728=ORIENTED_EDGE('',*,*,#13285,.T.);
#18729=ORIENTED_EDGE('',*,*,#13282,.T.);
#18730=ORIENTED_EDGE('',*,*,#13279,.T.);
#18731=ORIENTED_EDGE('',*,*,#13276,.T.);
#18732=ORIENTED_EDGE('',*,*,#13273,.T.);
#18733=ORIENTED_EDGE('',*,*,#13270,.T.);
#18734=ORIENTED_EDGE('',*,*,#13267,.T.);
#18735=ORIENTED_EDGE('',*,*,#13264,.T.);
#18736=ORIENTED_EDGE('',*,*,#13261,.T.);
#18737=ORIENTED_EDGE('',*,*,#13258,.T.);
#18738=ORIENTED_EDGE('',*,*,#13255,.T.);
#18739=ORIENTED_EDGE('',*,*,#13252,.T.);
#18740=ORIENTED_EDGE('',*,*,#13188,.T.);
#18741=ORIENTED_EDGE('',*,*,#13219,.T.);
#18742=ORIENTED_EDGE('',*,*,#13216,.T.);
#18743=ORIENTED_EDGE('',*,*,#13213,.T.);
#18744=ORIENTED_EDGE('',*,*,#13210,.T.);
#18745=ORIENTED_EDGE('',*,*,#13207,.T.);
#18746=ORIENTED_EDGE('',*,*,#13204,.T.);
#18747=ORIENTED_EDGE('',*,*,#13201,.T.);
#18748=ORIENTED_EDGE('',*,*,#13198,.T.);
#18749=ORIENTED_EDGE('',*,*,#13195,.T.);
#18750=ORIENTED_EDGE('',*,*,#13192,.T.);
#18751=ORIENTED_EDGE('',*,*,#13098,.T.);
#18752=ORIENTED_EDGE('',*,*,#13162,.T.);
#18753=ORIENTED_EDGE('',*,*,#13159,.T.);
#18754=ORIENTED_EDGE('',*,*,#13156,.T.);
#18755=ORIENTED_EDGE('',*,*,#13153,.T.);
#18756=ORIENTED_EDGE('',*,*,#13150,.T.);
#18757=ORIENTED_EDGE('',*,*,#13147,.T.);
#18758=ORIENTED_EDGE('',*,*,#13144,.T.);
#18759=ORIENTED_EDGE('',*,*,#13141,.T.);
#18760=ORIENTED_EDGE('',*,*,#13138,.T.);
#18761=ORIENTED_EDGE('',*,*,#13135,.T.);
#18762=ORIENTED_EDGE('',*,*,#13132,.T.);
#18763=ORIENTED_EDGE('',*,*,#13129,.T.);
#18764=ORIENTED_EDGE('',*,*,#13126,.T.);
#18765=ORIENTED_EDGE('',*,*,#13123,.T.);
#18766=ORIENTED_EDGE('',*,*,#13120,.T.);
#18767=ORIENTED_EDGE('',*,*,#13117,.T.);
#18768=ORIENTED_EDGE('',*,*,#13114,.T.);
#18769=ORIENTED_EDGE('',*,*,#13111,.T.);
#18770=ORIENTED_EDGE('',*,*,#13108,.T.);
#18771=ORIENTED_EDGE('',*,*,#13105,.T.);
#18772=ORIENTED_EDGE('',*,*,#13102,.T.);
#18773=ORIENTED_EDGE('',*,*,#13008,.T.);
#18774=ORIENTED_EDGE('',*,*,#13096,.T.);
#18775=ORIENTED_EDGE('',*,*,#13093,.T.);
#18776=ORIENTED_EDGE('',*,*,#13090,.T.);
#18777=ORIENTED_EDGE('',*,*,#13087,.T.);
#18778=ORIENTED_EDGE('',*,*,#13084,.T.);
#18779=ORIENTED_EDGE('',*,*,#13081,.T.);
#18780=ORIENTED_EDGE('',*,*,#13078,.T.);
#18781=ORIENTED_EDGE('',*,*,#13075,.T.);
#18782=ORIENTED_EDGE('',*,*,#13072,.T.);
#18783=ORIENTED_EDGE('',*,*,#13069,.T.);
#18784=ORIENTED_EDGE('',*,*,#13066,.T.);
#18785=ORIENTED_EDGE('',*,*,#13063,.T.);
#18786=ORIENTED_EDGE('',*,*,#13060,.T.);
#18787=ORIENTED_EDGE('',*,*,#13057,.T.);
#18788=ORIENTED_EDGE('',*,*,#13054,.T.);
#18789=ORIENTED_EDGE('',*,*,#13051,.T.);
#18790=ORIENTED_EDGE('',*,*,#13048,.T.);
#18791=ORIENTED_EDGE('',*,*,#13045,.T.);
#18792=ORIENTED_EDGE('',*,*,#13042,.T.);
#18793=ORIENTED_EDGE('',*,*,#13039,.T.);
#18794=ORIENTED_EDGE('',*,*,#13036,.T.);
#18795=ORIENTED_EDGE('',*,*,#13033,.T.);
#18796=ORIENTED_EDGE('',*,*,#13030,.T.);
#18797=ORIENTED_EDGE('',*,*,#13027,.T.);
#18798=ORIENTED_EDGE('',*,*,#13024,.T.);
#18799=ORIENTED_EDGE('',*,*,#13021,.T.);
#18800=ORIENTED_EDGE('',*,*,#13018,.T.);
#18801=ORIENTED_EDGE('',*,*,#13015,.T.);
#18802=ORIENTED_EDGE('',*,*,#13012,.T.);
#18803=ORIENTED_EDGE('',*,*,#12903,.T.);
#18804=ORIENTED_EDGE('',*,*,#13006,.T.);
#18805=ORIENTED_EDGE('',*,*,#13003,.T.);
#18806=ORIENTED_EDGE('',*,*,#13000,.T.);
#18807=ORIENTED_EDGE('',*,*,#12997,.T.);
#18808=ORIENTED_EDGE('',*,*,#12994,.T.);
#18809=ORIENTED_EDGE('',*,*,#12991,.T.);
#18810=ORIENTED_EDGE('',*,*,#12988,.T.);
#18811=ORIENTED_EDGE('',*,*,#12985,.T.);
#18812=ORIENTED_EDGE('',*,*,#12982,.T.);
#18813=ORIENTED_EDGE('',*,*,#12979,.T.);
#18814=ORIENTED_EDGE('',*,*,#12976,.T.);
#18815=ORIENTED_EDGE('',*,*,#12973,.T.);
#18816=ORIENTED_EDGE('',*,*,#12970,.T.);
#18817=ORIENTED_EDGE('',*,*,#12967,.T.);
#18818=ORIENTED_EDGE('',*,*,#12964,.T.);
#18819=ORIENTED_EDGE('',*,*,#12961,.T.);
#18820=ORIENTED_EDGE('',*,*,#12958,.T.);
#18821=ORIENTED_EDGE('',*,*,#12955,.T.);
#18822=ORIENTED_EDGE('',*,*,#12952,.T.);
#18823=ORIENTED_EDGE('',*,*,#12949,.T.);
#18824=ORIENTED_EDGE('',*,*,#12946,.T.);
#18825=ORIENTED_EDGE('',*,*,#12943,.T.);
#18826=ORIENTED_EDGE('',*,*,#12940,.T.);
#18827=ORIENTED_EDGE('',*,*,#12937,.T.);
#18828=ORIENTED_EDGE('',*,*,#12934,.T.);
#18829=ORIENTED_EDGE('',*,*,#12931,.T.);
#18830=ORIENTED_EDGE('',*,*,#12928,.T.);
#18831=ORIENTED_EDGE('',*,*,#12925,.T.);
#18832=ORIENTED_EDGE('',*,*,#12922,.T.);
#18833=ORIENTED_EDGE('',*,*,#12919,.T.);
#18834=ORIENTED_EDGE('',*,*,#12916,.T.);
#18835=ORIENTED_EDGE('',*,*,#12913,.T.);
#18836=ORIENTED_EDGE('',*,*,#12910,.T.);
#18837=ORIENTED_EDGE('',*,*,#12907,.T.);
#18838=ORIENTED_EDGE('',*,*,#12879,.T.);
#18839=ORIENTED_EDGE('',*,*,#12901,.T.);
#18840=ORIENTED_EDGE('',*,*,#12898,.T.);
#18841=ORIENTED_EDGE('',*,*,#12895,.T.);
#18842=ORIENTED_EDGE('',*,*,#12892,.T.);
#18843=ORIENTED_EDGE('',*,*,#12889,.T.);
#18844=ORIENTED_EDGE('',*,*,#12886,.T.);
#18845=ORIENTED_EDGE('',*,*,#12883,.T.);
#18846=ORIENTED_EDGE('',*,*,#12852,.T.);
#18847=ORIENTED_EDGE('',*,*,#12862,.T.);
#18848=ORIENTED_EDGE('',*,*,#12859,.T.);
#18849=ORIENTED_EDGE('',*,*,#12856,.T.);
#18850=ORIENTED_EDGE('',*,*,#12762,.T.);
#18851=ORIENTED_EDGE('',*,*,#12850,.T.);
#18852=ORIENTED_EDGE('',*,*,#12847,.T.);
#18853=ORIENTED_EDGE('',*,*,#12844,.T.);
#18854=ORIENTED_EDGE('',*,*,#12841,.T.);
#18855=ORIENTED_EDGE('',*,*,#12838,.T.);
#18856=ORIENTED_EDGE('',*,*,#12835,.T.);
#18857=ORIENTED_EDGE('',*,*,#12832,.T.);
#18858=ORIENTED_EDGE('',*,*,#12829,.T.);
#18859=ORIENTED_EDGE('',*,*,#12826,.T.);
#18860=ORIENTED_EDGE('',*,*,#12823,.T.);
#18861=ORIENTED_EDGE('',*,*,#12820,.T.);
#18862=ORIENTED_EDGE('',*,*,#12817,.T.);
#18863=ORIENTED_EDGE('',*,*,#12814,.T.);
#18864=ORIENTED_EDGE('',*,*,#12811,.T.);
#18865=ORIENTED_EDGE('',*,*,#12808,.T.);
#18866=ORIENTED_EDGE('',*,*,#12805,.T.);
#18867=ORIENTED_EDGE('',*,*,#12802,.T.);
#18868=ORIENTED_EDGE('',*,*,#12799,.T.);
#18869=ORIENTED_EDGE('',*,*,#12796,.T.);
#18870=ORIENTED_EDGE('',*,*,#12793,.T.);
#18871=ORIENTED_EDGE('',*,*,#12790,.T.);
#18872=ORIENTED_EDGE('',*,*,#12787,.T.);
#18873=ORIENTED_EDGE('',*,*,#12784,.T.);
#18874=ORIENTED_EDGE('',*,*,#12781,.T.);
#18875=ORIENTED_EDGE('',*,*,#12778,.T.);
#18876=ORIENTED_EDGE('',*,*,#12775,.T.);
#18877=ORIENTED_EDGE('',*,*,#12772,.T.);
#18878=ORIENTED_EDGE('',*,*,#12769,.T.);
#18879=ORIENTED_EDGE('',*,*,#12766,.T.);
#18880=ORIENTED_EDGE('',*,*,#12717,.T.);
#18881=ORIENTED_EDGE('',*,*,#12760,.T.);
#18882=ORIENTED_EDGE('',*,*,#12757,.T.);
#18883=ORIENTED_EDGE('',*,*,#12754,.T.);
#18884=ORIENTED_EDGE('',*,*,#12751,.T.);
#18885=ORIENTED_EDGE('',*,*,#12748,.T.);
#18886=ORIENTED_EDGE('',*,*,#12745,.T.);
#18887=ORIENTED_EDGE('',*,*,#12742,.T.);
#18888=ORIENTED_EDGE('',*,*,#12739,.T.);
#18889=ORIENTED_EDGE('',*,*,#12736,.T.);
#18890=ORIENTED_EDGE('',*,*,#12733,.T.);
#18891=ORIENTED_EDGE('',*,*,#12730,.T.);
#18892=ORIENTED_EDGE('',*,*,#12727,.T.);
#18893=ORIENTED_EDGE('',*,*,#12724,.T.);
#18894=ORIENTED_EDGE('',*,*,#12721,.T.);
#18895=ORIENTED_EDGE('',*,*,#12690,.T.);
#18896=ORIENTED_EDGE('',*,*,#12715,.T.);
#18897=ORIENTED_EDGE('',*,*,#12712,.T.);
#18898=ORIENTED_EDGE('',*,*,#12709,.T.);
#18899=ORIENTED_EDGE('',*,*,#12706,.T.);
#18900=ORIENTED_EDGE('',*,*,#12703,.T.);
#18901=ORIENTED_EDGE('',*,*,#12700,.T.);
#18902=ORIENTED_EDGE('',*,*,#12697,.T.);
#18903=ORIENTED_EDGE('',*,*,#12694,.T.);
#18904=ORIENTED_EDGE('',*,*,#12654,.T.);
#18905=ORIENTED_EDGE('',*,*,#12688,.T.);
#18906=ORIENTED_EDGE('',*,*,#12685,.T.);
#18907=ORIENTED_EDGE('',*,*,#12682,.T.);
#18908=ORIENTED_EDGE('',*,*,#12679,.T.);
#18909=ORIENTED_EDGE('',*,*,#12676,.T.);
#18910=ORIENTED_EDGE('',*,*,#12673,.T.);
#18911=ORIENTED_EDGE('',*,*,#12670,.T.);
#18912=ORIENTED_EDGE('',*,*,#12667,.T.);
#18913=ORIENTED_EDGE('',*,*,#12664,.T.);
#18914=ORIENTED_EDGE('',*,*,#12661,.T.);
#18915=ORIENTED_EDGE('',*,*,#12658,.T.);
#18916=ORIENTED_EDGE('',*,*,#12549,.T.);
#18917=ORIENTED_EDGE('',*,*,#12628,.T.);
#18918=ORIENTED_EDGE('',*,*,#12625,.T.);
#18919=ORIENTED_EDGE('',*,*,#12622,.T.);
#18920=ORIENTED_EDGE('',*,*,#12619,.T.);
#18921=ORIENTED_EDGE('',*,*,#12616,.T.);
#18922=ORIENTED_EDGE('',*,*,#12613,.T.);
#18923=ORIENTED_EDGE('',*,*,#12610,.T.);
#18924=ORIENTED_EDGE('',*,*,#12607,.T.);
#18925=ORIENTED_EDGE('',*,*,#12604,.T.);
#18926=ORIENTED_EDGE('',*,*,#12601,.T.);
#18927=ORIENTED_EDGE('',*,*,#12598,.T.);
#18928=ORIENTED_EDGE('',*,*,#12595,.T.);
#18929=ORIENTED_EDGE('',*,*,#12592,.T.);
#18930=ORIENTED_EDGE('',*,*,#12589,.T.);
#18931=ORIENTED_EDGE('',*,*,#12586,.T.);
#18932=ORIENTED_EDGE('',*,*,#12583,.T.);
#18933=ORIENTED_EDGE('',*,*,#12580,.T.);
#18934=ORIENTED_EDGE('',*,*,#12577,.T.);
#18935=ORIENTED_EDGE('',*,*,#12574,.T.);
#18936=ORIENTED_EDGE('',*,*,#12571,.T.);
#18937=ORIENTED_EDGE('',*,*,#12568,.T.);
#18938=ORIENTED_EDGE('',*,*,#12565,.T.);
#18939=ORIENTED_EDGE('',*,*,#12562,.T.);
#18940=ORIENTED_EDGE('',*,*,#12559,.T.);
#18941=ORIENTED_EDGE('',*,*,#12556,.T.);
#18942=ORIENTED_EDGE('',*,*,#12553,.T.);
#18943=ORIENTED_EDGE('',*,*,#13430,.F.);
#18944=ORIENTED_EDGE('',*,*,#13477,.T.);
#18945=ORIENTED_EDGE('',*,*,#13437,.T.);
#18946=ORIENTED_EDGE('',*,*,#13477,.F.);
#18947=ORIENTED_EDGE('',*,*,#13478,.F.);
#18948=ORIENTED_EDGE('',*,*,#13478,.T.);
#18949=ORIENTED_EDGE('',*,*,#13479,.T.);
#18950=ORIENTED_EDGE('',*,*,#13480,.F.);
#18951=ORIENTED_EDGE('',*,*,#13479,.F.);
#18952=ORIENTED_EDGE('',*,*,#13475,.F.);
#18953=ORIENTED_EDGE('',*,*,#13480,.T.);
#21403=CONICAL_SURFACE('',#24088,0.8781,0.785398163397448);
#21404=CONICAL_SURFACE('',#24094,0.25,1.02974425867665);
#21405=CONICAL_SURFACE('',#24108,0.429999999999999,0.785398163397448);
#21406=CONICAL_SURFACE('',#24121,0.429999999999999,0.785398163397448);
#21407=CONICAL_SURFACE('',#24125,0.43,0.785398163397448);
#21408=CONICAL_SURFACE('',#24129,0.429999999999999,0.785398163397448);
#21409=CONICAL_SURFACE('',#24133,0.43,0.785398163397448);
#21410=CONICAL_SURFACE('',#24137,0.429999999999999,0.785398163397448);
#21411=CONICAL_SURFACE('',#24141,0.404999999999999,1.02974425867665);
#21412=CONICAL_SURFACE('',#24142,0.405,1.02974425867665);
#21413=CONICAL_SURFACE('',#24143,0.404999999999999,1.02974425867665);
#21414=CONICAL_SURFACE('',#24144,0.405,1.02974425867666);
#21415=CONICAL_SURFACE('',#24145,0.404999999999999,1.02974425867665);
#21416=CONICAL_SURFACE('',#24146,0.404999999999999,1.02974425867665);
#21417=CONICAL_SURFACE('',#24147,2.63,0.785398163397448);
#21418=CONICAL_SURFACE('',#24153,6.975,0.785398163397444);
#21993=ADVANCED_FACE('',(#3163),#332,.F.);
#21994=ADVANCED_FACE('',(#3164),#333,.F.);
#21995=ADVANCED_FACE('',(#3165),#334,.F.);
#21996=ADVANCED_FACE('',(#3166),#335,.F.);
#21997=ADVANCED_FACE('',(#3167),#336,.F.);
#21998=ADVANCED_FACE('',(#3168),#337,.F.);
#21999=ADVANCED_FACE('',(#3169),#338,.F.);
#22000=ADVANCED_FACE('',(#3170),#339,.F.);
#22001=ADVANCED_FACE('',(#3171),#340,.F.);
#22002=ADVANCED_FACE('',(#3172),#2051,.F.);
#22003=ADVANCED_FACE('',(#3173),#341,.F.);
#22004=ADVANCED_FACE('',(#3174),#342,.F.);
#22005=ADVANCED_FACE('',(#3175),#2052,.F.);
#22006=ADVANCED_FACE('',(#3176),#343,.F.);
#22007=ADVANCED_FACE('',(#3177),#344,.F.);
#22008=ADVANCED_FACE('',(#3178),#345,.F.);
#22009=ADVANCED_FACE('',(#3179),#346,.F.);
#22010=ADVANCED_FACE('',(#3180),#347,.F.);
#22011=ADVANCED_FACE('',(#3181),#348,.F.);
#22012=ADVANCED_FACE('',(#3182),#349,.F.);
#22013=ADVANCED_FACE('',(#3183),#2053,.F.);
#22014=ADVANCED_FACE('',(#3184),#350,.F.);
#22015=ADVANCED_FACE('',(#3185),#351,.F.);
#22016=ADVANCED_FACE('',(#3186),#352,.F.);
#22017=ADVANCED_FACE('',(#3187),#353,.F.);
#22018=ADVANCED_FACE('',(#3188),#354,.F.);
#22019=ADVANCED_FACE('',(#3189),#355,.F.);
#22020=ADVANCED_FACE('',(#3190),#356,.F.);
#22021=ADVANCED_FACE('',(#3191),#357,.F.);
#22022=ADVANCED_FACE('',(#3192),#358,.F.);
#22023=ADVANCED_FACE('',(#3193),#359,.F.);
#22024=ADVANCED_FACE('',(#3194),#360,.F.);
#22025=ADVANCED_FACE('',(#3195),#361,.F.);
#22026=ADVANCED_FACE('',(#3196),#362,.F.);
#22027=ADVANCED_FACE('',(#3197),#363,.F.);
#22028=ADVANCED_FACE('',(#3198),#364,.F.);
#22029=ADVANCED_FACE('',(#3199),#2054,.F.);
#22030=ADVANCED_FACE('',(#3200,#1716),#2055,.T.);
#22031=ADVANCED_FACE('',(#3201),#365,.F.);
#22032=ADVANCED_FACE('',(#3202),#366,.F.);
#22033=ADVANCED_FACE('',(#3203),#367,.F.);
#22034=ADVANCED_FACE('',(#3204),#368,.F.);
#22035=ADVANCED_FACE('',(#3205),#369,.F.);
#22036=ADVANCED_FACE('',(#3206),#370,.F.);
#22037=ADVANCED_FACE('',(#3207),#371,.F.);
#22038=ADVANCED_FACE('',(#3208),#372,.F.);
#22039=ADVANCED_FACE('',(#3209),#373,.F.);
#22040=ADVANCED_FACE('',(#3210),#374,.F.);
#22041=ADVANCED_FACE('',(#3211),#375,.F.);
#22042=ADVANCED_FACE('',(#3212),#376,.F.);
#22043=ADVANCED_FACE('',(#3213),#377,.F.);
#22044=ADVANCED_FACE('',(#3214),#378,.F.);
#22045=ADVANCED_FACE('',(#3215),#379,.F.);
#22046=ADVANCED_FACE('',(#3216),#380,.F.);
#22047=ADVANCED_FACE('',(#3217),#381,.F.);
#22048=ADVANCED_FACE('',(#3218),#382,.F.);
#22049=ADVANCED_FACE('',(#3219),#383,.F.);
#22050=ADVANCED_FACE('',(#3220),#384,.F.);
#22051=ADVANCED_FACE('',(#3221,#1717),#2056,.T.);
#22052=ADVANCED_FACE('',(#3222),#385,.F.);
#22053=ADVANCED_FACE('',(#3223),#386,.F.);
#22054=ADVANCED_FACE('',(#3224),#2057,.F.);
#22055=ADVANCED_FACE('',(#3225),#387,.F.);
#22056=ADVANCED_FACE('',(#3226),#388,.F.);
#22057=ADVANCED_FACE('',(#3227),#2058,.F.);
#22058=ADVANCED_FACE('',(#3228),#2059,.F.);
#22059=ADVANCED_FACE('',(#3229),#2060,.F.);
#22060=ADVANCED_FACE('',(#3230),#2061,.F.);
#22061=ADVANCED_FACE('',(#3231),#2062,.T.);
#22062=ADVANCED_FACE('',(#3232),#2063,.F.);
#22063=ADVANCED_FACE('',(#3233),#2064,.F.);
#22064=ADVANCED_FACE('',(#3234),#2065,.F.);
#22065=ADVANCED_FACE('',(#3235),#2066,.F.);
#22066=ADVANCED_FACE('',(#3236),#2067,.F.);
#22067=ADVANCED_FACE('',(#3237),#2068,.F.);
#22068=ADVANCED_FACE('',(#3238),#2069,.F.);
#22069=ADVANCED_FACE('',(#3239),#2070,.F.);
#22070=ADVANCED_FACE('',(#3240),#389,.F.);
#22071=ADVANCED_FACE('',(#3241),#390,.F.);
#22072=ADVANCED_FACE('',(#3242),#2071,.F.);
#22073=ADVANCED_FACE('',(#3243),#2072,.F.);
#22074=ADVANCED_FACE('',(#3244),#2073,.F.);
#22075=ADVANCED_FACE('',(#3245),#2074,.F.);
#22076=ADVANCED_FACE('',(#3246),#2075,.F.);
#22077=ADVANCED_FACE('',(#3247),#2076,.T.);
#22078=ADVANCED_FACE('',(#3248),#391,.F.);
#22079=ADVANCED_FACE('',(#3249),#392,.F.);
#22080=ADVANCED_FACE('',(#3250),#393,.F.);
#22081=ADVANCED_FACE('',(#3251),#394,.F.);
#22082=ADVANCED_FACE('',(#3252),#395,.F.);
#22083=ADVANCED_FACE('',(#3253),#396,.F.);
#22084=ADVANCED_FACE('',(#3254),#397,.F.);
#22085=ADVANCED_FACE('',(#3255),#398,.F.);
#22086=ADVANCED_FACE('',(#3256),#399,.F.);
#22087=ADVANCED_FACE('',(#3257),#400,.F.);
#22088=ADVANCED_FACE('',(#3258),#401,.F.);
#22089=ADVANCED_FACE('',(#3259),#2077,.F.);
#22090=ADVANCED_FACE('',(#3260),#402,.F.);
#22091=ADVANCED_FACE('',(#3261),#403,.F.);
#22092=ADVANCED_FACE('',(#3262),#404,.F.);
#22093=ADVANCED_FACE('',(#3263),#405,.F.);
#22094=ADVANCED_FACE('',(#3264),#406,.F.);
#22095=ADVANCED_FACE('',(#3265),#407,.F.);
#22096=ADVANCED_FACE('',(#3266),#408,.F.);
#22097=ADVANCED_FACE('',(#3267),#2078,.F.);
#22098=ADVANCED_FACE('',(#3268),#409,.F.);
#22099=ADVANCED_FACE('',(#3269),#410,.F.);
#22100=ADVANCED_FACE('',(#3270),#411,.F.);
#22101=ADVANCED_FACE('',(#3271),#412,.F.);
#22102=ADVANCED_FACE('',(#3272),#413,.F.);
#22103=ADVANCED_FACE('',(#3273),#414,.F.);
#22104=ADVANCED_FACE('',(#3274),#415,.F.);
#22105=ADVANCED_FACE('',(#3275),#2079,.F.);
#22106=ADVANCED_FACE('',(#3276),#416,.F.);
#22107=ADVANCED_FACE('',(#3277),#417,.F.);
#22108=ADVANCED_FACE('',(#3278),#2080,.T.);
#22109=ADVANCED_FACE('',(#3279),#2081,.F.);
#22110=ADVANCED_FACE('',(#3280),#2082,.F.);
#22111=ADVANCED_FACE('',(#3281),#2083,.F.);
#22112=ADVANCED_FACE('',(#3282),#2084,.F.);
#22113=ADVANCED_FACE('',(#3283),#2085,.F.);
#22114=ADVANCED_FACE('',(#3284),#418,.F.);
#22115=ADVANCED_FACE('',(#3285),#419,.F.);
#22116=ADVANCED_FACE('',(#3286),#2086,.F.);
#22117=ADVANCED_FACE('',(#3287),#2087,.F.);
#22118=ADVANCED_FACE('',(#3288),#2088,.F.);
#22119=ADVANCED_FACE('',(#3289),#2089,.F.);
#22120=ADVANCED_FACE('',(#3290),#2090,.F.);
#22121=ADVANCED_FACE('',(#3291),#2091,.F.);
#22122=ADVANCED_FACE('',(#3292),#2092,.F.);
#22123=ADVANCED_FACE('',(#3293),#2093,.F.);
#22124=ADVANCED_FACE('',(#3294),#2094,.F.);
#22125=ADVANCED_FACE('',(#3295),#2095,.F.);
#22126=ADVANCED_FACE('',(#3296),#2096,.F.);
#22127=ADVANCED_FACE('',(#3297,#1718),#2097,.T.);
#22128=ADVANCED_FACE('',(#3298),#420,.F.);
#22129=ADVANCED_FACE('',(#3299),#421,.F.);
#22130=ADVANCED_FACE('',(#3300),#422,.F.);
#22131=ADVANCED_FACE('',(#3301),#423,.F.);
#22132=ADVANCED_FACE('',(#3302),#424,.F.);
#22133=ADVANCED_FACE('',(#3303),#425,.F.);
#22134=ADVANCED_FACE('',(#3304),#426,.F.);
#22135=ADVANCED_FACE('',(#3305),#427,.F.);
#22136=ADVANCED_FACE('',(#3306),#428,.F.);
#22137=ADVANCED_FACE('',(#3307),#429,.F.);
#22138=ADVANCED_FACE('',(#3308),#430,.F.);
#22139=ADVANCED_FACE('',(#3309),#431,.F.);
#22140=ADVANCED_FACE('',(#3310),#432,.F.);
#22141=ADVANCED_FACE('',(#3311),#2098,.F.);
#22142=ADVANCED_FACE('',(#3312),#433,.F.);
#22143=ADVANCED_FACE('',(#3313),#434,.F.);
#22144=ADVANCED_FACE('',(#3314),#435,.F.);
#22145=ADVANCED_FACE('',(#3315),#436,.F.);
#22146=ADVANCED_FACE('',(#3316),#437,.F.);
#22147=ADVANCED_FACE('',(#3317),#438,.F.);
#22148=ADVANCED_FACE('',(#3318),#439,.F.);
#22149=ADVANCED_FACE('',(#3319),#440,.F.);
#22150=ADVANCED_FACE('',(#3320),#441,.F.);
#22151=ADVANCED_FACE('',(#3321),#442,.F.);
#22152=ADVANCED_FACE('',(#3322),#443,.F.);
#22153=ADVANCED_FACE('',(#3323),#444,.F.);
#22154=ADVANCED_FACE('',(#3324),#445,.F.);
#22155=ADVANCED_FACE('',(#3325),#446,.F.);
#22156=ADVANCED_FACE('',(#3326),#447,.F.);
#22157=ADVANCED_FACE('',(#3327),#448,.F.);
#22158=ADVANCED_FACE('',(#3328),#449,.F.);
#22159=ADVANCED_FACE('',(#3329),#450,.F.);
#22160=ADVANCED_FACE('',(#3330),#2099,.F.);
#22161=ADVANCED_FACE('',(#3331),#451,.F.);
#22162=ADVANCED_FACE('',(#3332),#452,.F.);
#22163=ADVANCED_FACE('',(#3333),#2100,.T.);
#22164=ADVANCED_FACE('',(#3334),#453,.F.);
#22165=ADVANCED_FACE('',(#3335),#454,.F.);
#22166=ADVANCED_FACE('',(#3336),#455,.F.);
#22167=ADVANCED_FACE('',(#3337),#456,.F.);
#22168=ADVANCED_FACE('',(#3338),#457,.F.);
#22169=ADVANCED_FACE('',(#3339),#458,.F.);
#22170=ADVANCED_FACE('',(#3340),#459,.F.);
#22171=ADVANCED_FACE('',(#3341),#460,.F.);
#22172=ADVANCED_FACE('',(#3342),#461,.F.);
#22173=ADVANCED_FACE('',(#3343),#462,.F.);
#22174=ADVANCED_FACE('',(#3344),#463,.F.);
#22175=ADVANCED_FACE('',(#3345),#2101,.F.);
#22176=ADVANCED_FACE('',(#3346),#464,.F.);
#22177=ADVANCED_FACE('',(#3347),#465,.F.);
#22178=ADVANCED_FACE('',(#3348),#466,.F.);
#22179=ADVANCED_FACE('',(#3349),#467,.F.);
#22180=ADVANCED_FACE('',(#3350),#468,.F.);
#22181=ADVANCED_FACE('',(#3351),#469,.F.);
#22182=ADVANCED_FACE('',(#3352),#470,.F.);
#22183=ADVANCED_FACE('',(#3353),#2102,.F.);
#22184=ADVANCED_FACE('',(#3354),#471,.F.);
#22185=ADVANCED_FACE('',(#3355),#472,.F.);
#22186=ADVANCED_FACE('',(#3356),#473,.F.);
#22187=ADVANCED_FACE('',(#3357),#474,.F.);
#22188=ADVANCED_FACE('',(#3358),#475,.F.);
#22189=ADVANCED_FACE('',(#3359),#476,.F.);
#22190=ADVANCED_FACE('',(#3360),#477,.F.);
#22191=ADVANCED_FACE('',(#3361),#2103,.F.);
#22192=ADVANCED_FACE('',(#3362),#478,.F.);
#22193=ADVANCED_FACE('',(#3363),#479,.F.);
#22194=ADVANCED_FACE('',(#3364),#2104,.T.);
#22195=ADVANCED_FACE('',(#3365),#480,.F.);
#22196=ADVANCED_FACE('',(#3366),#481,.F.);
#22197=ADVANCED_FACE('',(#3367),#482,.F.);
#22198=ADVANCED_FACE('',(#3368),#483,.F.);
#22199=ADVANCED_FACE('',(#3369),#484,.F.);
#22200=ADVANCED_FACE('',(#3370),#485,.F.);
#22201=ADVANCED_FACE('',(#3371),#486,.F.);
#22202=ADVANCED_FACE('',(#3372),#487,.F.);
#22203=ADVANCED_FACE('',(#3373),#2105,.F.);
#22204=ADVANCED_FACE('',(#3374),#488,.F.);
#22205=ADVANCED_FACE('',(#3375),#489,.F.);
#22206=ADVANCED_FACE('',(#3376),#490,.F.);
#22207=ADVANCED_FACE('',(#3377),#491,.F.);
#22208=ADVANCED_FACE('',(#3378),#492,.F.);
#22209=ADVANCED_FACE('',(#3379),#493,.F.);
#22210=ADVANCED_FACE('',(#3380),#494,.F.);
#22211=ADVANCED_FACE('',(#3381),#495,.F.);
#22212=ADVANCED_FACE('',(#3382),#496,.F.);
#22213=ADVANCED_FACE('',(#3383),#2106,.F.);
#22214=ADVANCED_FACE('',(#3384),#2107,.F.);
#22215=ADVANCED_FACE('',(#3385),#2108,.F.);
#22216=ADVANCED_FACE('',(#3386),#497,.F.);
#22217=ADVANCED_FACE('',(#3387),#2109,.T.);
#22218=ADVANCED_FACE('',(#3388),#2110,.F.);
#22219=ADVANCED_FACE('',(#3389),#498,.F.);
#22220=ADVANCED_FACE('',(#3390),#499,.F.);
#22221=ADVANCED_FACE('',(#3391),#500,.F.);
#22222=ADVANCED_FACE('',(#3392),#501,.F.);
#22223=ADVANCED_FACE('',(#3393),#502,.F.);
#22224=ADVANCED_FACE('',(#3394),#2111,.F.);
#22225=ADVANCED_FACE('',(#3395),#2112,.F.);
#22226=ADVANCED_FACE('',(#3396),#2113,.F.);
#22227=ADVANCED_FACE('',(#3397),#503,.F.);
#22228=ADVANCED_FACE('',(#3398),#504,.F.);
#22229=ADVANCED_FACE('',(#3399),#505,.F.);
#22230=ADVANCED_FACE('',(#3400),#506,.F.);
#22231=ADVANCED_FACE('',(#3401),#507,.F.);
#22232=ADVANCED_FACE('',(#3402),#508,.F.);
#22233=ADVANCED_FACE('',(#3403),#2114,.F.);
#22234=ADVANCED_FACE('',(#3404),#2115,.F.);
#22235=ADVANCED_FACE('',(#3405),#2116,.F.);
#22236=ADVANCED_FACE('',(#3406),#2117,.F.);
#22237=ADVANCED_FACE('',(#3407,#1719),#2118,.T.);
#22238=ADVANCED_FACE('',(#3408),#509,.F.);
#22239=ADVANCED_FACE('',(#3409),#510,.F.);
#22240=ADVANCED_FACE('',(#3410),#511,.F.);
#22241=ADVANCED_FACE('',(#3411),#512,.F.);
#22242=ADVANCED_FACE('',(#3412),#513,.F.);
#22243=ADVANCED_FACE('',(#3413),#514,.F.);
#22244=ADVANCED_FACE('',(#3414),#515,.F.);
#22245=ADVANCED_FACE('',(#3415),#516,.F.);
#22246=ADVANCED_FACE('',(#3416),#517,.F.);
#22247=ADVANCED_FACE('',(#3417),#518,.F.);
#22248=ADVANCED_FACE('',(#3418),#519,.F.);
#22249=ADVANCED_FACE('',(#3419),#520,.F.);
#22250=ADVANCED_FACE('',(#3420),#521,.F.);
#22251=ADVANCED_FACE('',(#3421),#522,.F.);
#22252=ADVANCED_FACE('',(#3422),#523,.F.);
#22253=ADVANCED_FACE('',(#3423),#524,.F.);
#22254=ADVANCED_FACE('',(#3424),#525,.F.);
#22255=ADVANCED_FACE('',(#3425),#526,.F.);
#22256=ADVANCED_FACE('',(#3426),#527,.F.);
#22257=ADVANCED_FACE('',(#3427),#528,.F.);
#22258=ADVANCED_FACE('',(#3428),#529,.F.);
#22259=ADVANCED_FACE('',(#3429),#530,.F.);
#22260=ADVANCED_FACE('',(#3430),#531,.F.);
#22261=ADVANCED_FACE('',(#3431),#532,.F.);
#22262=ADVANCED_FACE('',(#3432),#533,.F.);
#22263=ADVANCED_FACE('',(#3433),#2119,.F.);
#22264=ADVANCED_FACE('',(#3434),#534,.F.);
#22265=ADVANCED_FACE('',(#3435),#535,.F.);
#22266=ADVANCED_FACE('',(#3436,#1720),#2120,.T.);
#22267=ADVANCED_FACE('',(#3437),#536,.F.);
#22268=ADVANCED_FACE('',(#3438),#537,.F.);
#22269=ADVANCED_FACE('',(#3439),#538,.F.);
#22270=ADVANCED_FACE('',(#3440),#539,.F.);
#22271=ADVANCED_FACE('',(#3441),#540,.F.);
#22272=ADVANCED_FACE('',(#3442),#541,.F.);
#22273=ADVANCED_FACE('',(#3443),#542,.F.);
#22274=ADVANCED_FACE('',(#3444),#543,.F.);
#22275=ADVANCED_FACE('',(#3445),#544,.F.);
#22276=ADVANCED_FACE('',(#3446),#545,.F.);
#22277=ADVANCED_FACE('',(#3447),#546,.F.);
#22278=ADVANCED_FACE('',(#3448),#547,.F.);
#22279=ADVANCED_FACE('',(#3449),#548,.F.);
#22280=ADVANCED_FACE('',(#3450),#549,.F.);
#22281=ADVANCED_FACE('',(#3451),#550,.F.);
#22282=ADVANCED_FACE('',(#3452),#2121,.F.);
#22283=ADVANCED_FACE('',(#3453),#2122,.F.);
#22284=ADVANCED_FACE('',(#3454),#2123,.F.);
#22285=ADVANCED_FACE('',(#3455),#2124,.F.);
#22286=ADVANCED_FACE('',(#3456),#2125,.F.);
#22287=ADVANCED_FACE('',(#3457),#551,.F.);
#22288=ADVANCED_FACE('',(#3458,#1721),#2126,.T.);
#22289=ADVANCED_FACE('',(#3459),#552,.F.);
#22290=ADVANCED_FACE('',(#3460),#553,.F.);
#22291=ADVANCED_FACE('',(#3461),#554,.F.);
#22292=ADVANCED_FACE('',(#3462),#555,.F.);
#22293=ADVANCED_FACE('',(#3463),#2127,.F.);
#22294=ADVANCED_FACE('',(#3464),#556,.F.);
#22295=ADVANCED_FACE('',(#3465),#557,.F.);
#22296=ADVANCED_FACE('',(#3466),#558,.F.);
#22297=ADVANCED_FACE('',(#3467),#2128,.F.);
#22298=ADVANCED_FACE('',(#3468),#2129,.F.);
#22299=ADVANCED_FACE('',(#3469),#2130,.F.);
#22300=ADVANCED_FACE('',(#3470),#2131,.F.);
#22301=ADVANCED_FACE('',(#3471),#2132,.F.);
#22302=ADVANCED_FACE('',(#3472),#2133,.T.);
#22303=ADVANCED_FACE('',(#3473),#2134,.T.);
#22304=ADVANCED_FACE('',(#3474),#2135,.T.);
#22305=ADVANCED_FACE('',(#3475),#2136,.T.);
#22306=ADVANCED_FACE('',(#3476),#2137,.T.);
#22307=ADVANCED_FACE('',(#3477),#2138,.T.);
#22308=ADVANCED_FACE('',(#3478),#2139,.T.);
#22309=ADVANCED_FACE('',(#3479),#2553,.F.);
#22310=ADVANCED_FACE('',(#3480),#21403,.F.);
#22311=ADVANCED_FACE('',(#3481),#2554,.F.);
#22312=ADVANCED_FACE('',(#3482,#1722),#2140,.T.);
#22313=ADVANCED_FACE('',(#3483),#21404,.F.);
#22314=ADVANCED_FACE('',(#3484),#2555,.F.);
#22315=ADVANCED_FACE('',(#3485,#1723),#2141,.F.);
#22316=ADVANCED_FACE('',(#3486),#2142,.F.);
#22317=ADVANCED_FACE('',(#3487),#2556,.T.);
#22318=ADVANCED_FACE('',(#3488),#312,.T.);
#22319=ADVANCED_FACE('',(#3489),#21405,.F.);
#22320=ADVANCED_FACE('',(#3490,#1724,#1725,#1726,#1727,#1728,#1729,#1730,
#1731),#2143,.T.);
#22321=ADVANCED_FACE('',(#3491),#2557,.F.);
#22322=ADVANCED_FACE('',(#3492),#21406,.F.);
#22323=ADVANCED_FACE('',(#3493),#2558,.F.);
#22324=ADVANCED_FACE('',(#3494),#21407,.F.);
#22325=ADVANCED_FACE('',(#3495),#2559,.F.);
#22326=ADVANCED_FACE('',(#3496),#21408,.F.);
#22327=ADVANCED_FACE('',(#3497),#2560,.F.);
#22328=ADVANCED_FACE('',(#3498),#21409,.F.);
#22329=ADVANCED_FACE('',(#3499),#2561,.F.);
#22330=ADVANCED_FACE('',(#3500),#21410,.F.);
#22331=ADVANCED_FACE('',(#3501),#2562,.F.);
#22332=ADVANCED_FACE('',(#3502),#21411,.F.);
#22333=ADVANCED_FACE('',(#3503),#21412,.F.);
#22334=ADVANCED_FACE('',(#3504),#21413,.F.);
#22335=ADVANCED_FACE('',(#3505),#21414,.F.);
#22336=ADVANCED_FACE('',(#3506),#21415,.F.);
#22337=ADVANCED_FACE('',(#3507),#21416,.F.);
#22338=ADVANCED_FACE('',(#3508),#21417,.F.);
#22339=ADVANCED_FACE('',(#3509),#2563,.F.);
#22340=ADVANCED_FACE('',(#3510,#1732,#1733,#1734,#1735,#1736,#1737,#1738,
#1739,#1740,#1741,#1742,#1743,#1744,#1745),#2144,.T.);
#22341=ADVANCED_FACE('',(#3511),#21418,.T.);
#22342=ADVANCED_FACE('',(#3512),#2145,.T.);
#22343=ADVANCED_FACE('',(#3513),#2564,.F.);
#22344=ADVANCED_FACE('',(#3514,#1746),#2146,.T.);
#22816=CLOSED_SHELL('',(#21993,#21994,#21995,#21996,#21997,#21998,#21999,
#22000,#22001,#22002,#22003,#22004,#22005,#22006,#22007,#22008,#22009,#22010,
#22011,#22012,#22013,#22014,#22015,#22016,#22017,#22018,#22019,#22020,#22021,
#22022,#22023,#22024,#22025,#22026,#22027,#22028,#22029,#22030,#22031,#22032,
#22033,#22034,#22035,#22036,#22037,#22038,#22039,#22040,#22041,#22042,#22043,
#22044,#22045,#22046,#22047,#22048,#22049,#22050,#22051,#22052,#22053,#22054,
#22055,#22056,#22057,#22058,#22059,#22060,#22061,#22062,#22063,#22064,#22065,
#22066,#22067,#22068,#22069,#22070,#22071,#22072,#22073,#22074,#22075,#22076,
#22077,#22078,#22079,#22080,#22081,#22082,#22083,#22084,#22085,#22086,#22087,
#22088,#22089,#22090,#22091,#22092,#22093,#22094,#22095,#22096,#22097,#22098,
#22099,#22100,#22101,#22102,#22103,#22104,#22105,#22106,#22107,#22108,#22109,
#22110,#22111,#22112,#22113,#22114,#22115,#22116,#22117,#22118,#22119,#22120,
#22121,#22122,#22123,#22124,#22125,#22126,#22127,#22128,#22129,#22130,#22131,
#22132,#22133,#22134,#22135,#22136,#22137,#22138,#22139,#22140,#22141,#22142,
#22143,#22144,#22145,#22146,#22147,#22148,#22149,#22150,#22151,#22152,#22153,
#22154,#22155,#22156,#22157,#22158,#22159,#22160,#22161,#22162,#22163,#22164,
#22165,#22166,#22167,#22168,#22169,#22170,#22171,#22172,#22173,#22174,#22175,
#22176,#22177,#22178,#22179,#22180,#22181,#22182,#22183,#22184,#22185,#22186,
#22187,#22188,#22189,#22190,#22191,#22192,#22193,#22194,#22195,#22196,#22197,
#22198,#22199,#22200,#22201,#22202,#22203,#22204,#22205,#22206,#22207,#22208,
#22209,#22210,#22211,#22212,#22213,#22214,#22215,#22216,#22217,#22218,#22219,
#22220,#22221,#22222,#22223,#22224,#22225,#22226,#22227,#22228,#22229,#22230,
#22231,#22232,#22233,#22234,#22235,#22236,#22237,#22238,#22239,#22240,#22241,
#22242,#22243,#22244,#22245,#22246,#22247,#22248,#22249,#22250,#22251,#22252,
#22253,#22254,#22255,#22256,#22257,#22258,#22259,#22260,#22261,#22262,#22263,
#22264,#22265,#22266,#22267,#22268,#22269,#22270,#22271,#22272,#22273,#22274,
#22275,#22276,#22277,#22278,#22279,#22280,#22281,#22282,#22283,#22284,#22285,
#22286,#22287,#22288,#22289,#22290,#22291,#22292,#22293,#22294,#22295,#22296,
#22297,#22298,#22299,#22300,#22301,#22302,#22303,#22304,#22305,#22306,#22307,
#22308,#22309,#22310,#22311,#22312,#22313,#22314,#22315,#22316,#22317,#22318,
#22319,#22320,#22321,#22322,#22323,#22324,#22325,#22326,#22327,#22328,#22329,
#22330,#22331,#22332,#22333,#22334,#22335,#22336,#22337,#22338,#22339,#22340,
#22341,#22342,#22343,#22344));
#23996=AXIS2_PLACEMENT_3D('',#43215,#27551,#27552);
#23997=AXIS2_PLACEMENT_3D('',#43354,#27563,#27564);
#23998=AXIS2_PLACEMENT_3D('',#43390,#27570,#27571);
#23999=AXIS2_PLACEMENT_3D('',#43501,#27582,#27583);
#24000=AXIS2_PLACEMENT_3D('',#43732,#27602,#27603);
#24001=AXIS2_PLACEMENT_3D('',#43735,#27606,#27607);
#24002=AXIS2_PLACEMENT_3D('',#44036,#27628,#27629);
#24003=AXIS2_PLACEMENT_3D('',#44070,#27633,#27634);
#24004=AXIS2_PLACEMENT_3D('',#44106,#27640,#27641);
#24005=AXIS2_PLACEMENT_3D('',#44112,#27645,#27646);
#24006=AXIS2_PLACEMENT_3D('',#44118,#27650,#27651);
#24007=AXIS2_PLACEMENT_3D('',#44124,#27655,#27656);
#24008=AXIS2_PLACEMENT_3D('',#44127,#27659,#27660);
#24009=AXIS2_PLACEMENT_3D('',#44128,#27661,#27662);
#24010=AXIS2_PLACEMENT_3D('',#44137,#27667,#27668);
#24011=AXIS2_PLACEMENT_3D('',#44143,#27672,#27673);
#24012=AXIS2_PLACEMENT_3D('',#44149,#27677,#27678);
#24013=AXIS2_PLACEMENT_3D('',#44155,#27682,#27683);
#24014=AXIS2_PLACEMENT_3D('',#44161,#27687,#27688);
#24015=AXIS2_PLACEMENT_3D('',#44167,#27692,#27693);
#24016=AXIS2_PLACEMENT_3D('',#44173,#27697,#27698);
#24017=AXIS2_PLACEMENT_3D('',#44209,#27704,#27705);
#24018=AXIS2_PLACEMENT_3D('',#44215,#27709,#27710);
#24019=AXIS2_PLACEMENT_3D('',#44221,#27714,#27715);
#24020=AXIS2_PLACEMENT_3D('',#44227,#27719,#27720);
#24021=AXIS2_PLACEMENT_3D('',#44233,#27724,#27725);
#24022=AXIS2_PLACEMENT_3D('',#44236,#27728,#27729);
#24023=AXIS2_PLACEMENT_3D('',#44405,#27742,#27743);
#24024=AXIS2_PLACEMENT_3D('',#44516,#27754,#27755);
#24025=AXIS2_PLACEMENT_3D('',#44627,#27766,#27767);
#24026=AXIS2_PLACEMENT_3D('',#44660,#27772,#27773);
#24027=AXIS2_PLACEMENT_3D('',#44661,#27774,#27775);
#24028=AXIS2_PLACEMENT_3D('',#44670,#27780,#27781);
#24029=AXIS2_PLACEMENT_3D('',#44676,#27785,#27786);
#24030=AXIS2_PLACEMENT_3D('',#44682,#27790,#27791);
#24031=AXIS2_PLACEMENT_3D('',#44685,#27794,#27795);
#24032=AXIS2_PLACEMENT_3D('',#44719,#27799,#27800);
#24033=AXIS2_PLACEMENT_3D('',#44725,#27804,#27805);
#24034=AXIS2_PLACEMENT_3D('',#44731,#27809,#27810);
#24035=AXIS2_PLACEMENT_3D('',#44734,#27813,#27814);
#24036=AXIS2_PLACEMENT_3D('',#44743,#27819,#27820);
#24037=AXIS2_PLACEMENT_3D('',#44749,#27824,#27825);
#24038=AXIS2_PLACEMENT_3D('',#44755,#27829,#27830);
#24039=AXIS2_PLACEMENT_3D('',#44761,#27834,#27835);
#24040=AXIS2_PLACEMENT_3D('',#44767,#27839,#27840);
#24041=AXIS2_PLACEMENT_3D('',#44773,#27844,#27845);
#24042=AXIS2_PLACEMENT_3D('',#44779,#27849,#27850);
#24043=AXIS2_PLACEMENT_3D('',#44782,#27853,#27854);
#24044=AXIS2_PLACEMENT_3D('',#44981,#27869,#27870);
#24045=AXIS2_PLACEMENT_3D('',#45257,#27892,#27893);
#24046=AXIS2_PLACEMENT_3D('',#45290,#27898,#27899);
#24047=AXIS2_PLACEMENT_3D('',#45459,#27912,#27913);
#24048=AXIS2_PLACEMENT_3D('',#45570,#27924,#27925);
#24049=AXIS2_PLACEMENT_3D('',#45681,#27936,#27937);
#24050=AXIS2_PLACEMENT_3D('',#45714,#27942,#27943);
#24051=AXIS2_PLACEMENT_3D('',#45838,#27953,#27954);
#24052=AXIS2_PLACEMENT_3D('',#45979,#27967,#27968);
#24053=AXIS2_PLACEMENT_3D('',#45985,#27972,#27973);
#24054=AXIS2_PLACEMENT_3D('',#45991,#27977,#27978);
#24055=AXIS2_PLACEMENT_3D('',#46009,#27982,#27983);
#24056=AXIS2_PLACEMENT_3D('',#46010,#27984,#27985);
#24057=AXIS2_PLACEMENT_3D('',#46094,#27995,#27996);
#24058=AXIS2_PLACEMENT_3D('',#46100,#28000,#28001);
#24059=AXIS2_PLACEMENT_3D('',#46103,#28004,#28005);
#24060=AXIS2_PLACEMENT_3D('',#46202,#28016,#28017);
#24061=AXIS2_PLACEMENT_3D('',#46208,#28021,#28022);
#24062=AXIS2_PLACEMENT_3D('',#46214,#28026,#28027);
#24063=AXIS2_PLACEMENT_3D('',#46220,#28031,#28032);
#24064=AXIS2_PLACEMENT_3D('',#46223,#28035,#28036);
#24065=AXIS2_PLACEMENT_3D('',#46602,#28063,#28064);
#24066=AXIS2_PLACEMENT_3D('',#46635,#28069,#28070);
#24067=AXIS2_PLACEMENT_3D('',#46864,#28087,#28088);
#24068=AXIS2_PLACEMENT_3D('',#46870,#28092,#28093);
#24069=AXIS2_PLACEMENT_3D('',#46876,#28097,#28098);
#24070=AXIS2_PLACEMENT_3D('',#46882,#28102,#28103);
#24071=AXIS2_PLACEMENT_3D('',#46888,#28107,#28108);
#24072=AXIS2_PLACEMENT_3D('',#46906,#28112,#28113);
#24073=AXIS2_PLACEMENT_3D('',#46970,#28119,#28120);
#24074=AXIS2_PLACEMENT_3D('',#47021,#28127,#28128);
#24075=AXIS2_PLACEMENT_3D('',#47027,#28132,#28133);
#24076=AXIS2_PLACEMENT_3D('',#47033,#28137,#28138);
#24077=AXIS2_PLACEMENT_3D('',#47039,#28142,#28143);
#24078=AXIS2_PLACEMENT_3D('',#47045,#28147,#28148);
#24079=AXIS2_PLACEMENT_3D('',#47048,#28151,#28152);
#24080=AXIS2_PLACEMENT_3D('',#47049,#28153,#28154);
#24081=AXIS2_PLACEMENT_3D('',#47050,#28155,#28156);
#24082=AXIS2_PLACEMENT_3D('',#47051,#28157,#28158);
#24083=AXIS2_PLACEMENT_3D('',#47052,#28159,#28160);
#24084=AXIS2_PLACEMENT_3D('',#47053,#28161,#28162);
#24085=AXIS2_PLACEMENT_3D('',#47054,#28163,#28164);
#24086=AXIS2_PLACEMENT_3D('',#47055,#28165,#28166);
#24087=AXIS2_PLACEMENT_3D('',#47057,#28167,#28168);
#24088=AXIS2_PLACEMENT_3D('',#47103,#28170,#28171);
#24089=AXIS2_PLACEMENT_3D('',#47105,#28172,#28173);
#24090=AXIS2_PLACEMENT_3D('',#47108,#28175,#28176);
#24091=AXIS2_PLACEMENT_3D('',#47109,#28177,#28178);
#24092=AXIS2_PLACEMENT_3D('',#47111,#28179,#28180);
#24093=AXIS2_PLACEMENT_3D('',#47113,#28182,#28183);
#24094=AXIS2_PLACEMENT_3D('',#47147,#28187,#28188);
#24095=AXIS2_PLACEMENT_3D('',#47151,#28190,#28191);
#24096=AXIS2_PLACEMENT_3D('',#47152,#28192,#28193);
#24097=AXIS2_PLACEMENT_3D('',#47156,#28196,#28197);
#24098=AXIS2_PLACEMENT_3D('',#47157,#28198,#28199);
#24099=AXIS2_PLACEMENT_3D('',#47158,#28200,#28201);
#24100=AXIS2_PLACEMENT_3D('',#47159,#28202,#28203);
#24101=AXIS2_PLACEMENT_3D('',#47160,#28204,#28205);
#24102=AXIS2_PLACEMENT_3D('',#47162,#28206,#28207);
#24103=AXIS2_PLACEMENT_3D('',#47165,#28209,#28210);
#24104=AXIS2_PLACEMENT_3D('',#47166,#28211,#28212);
#24105=AXIS2_PLACEMENT_3D('',#47167,#28213,#28214);
#24106=AXIS2_PLACEMENT_3D('',#47169,#28215,#28216);
#24107=AXIS2_PLACEMENT_3D('',#47170,#28217,#28218);
#24108=AXIS2_PLACEMENT_3D('',#47171,#28219,#28220);
#24109=AXIS2_PLACEMENT_3D('',#47173,#28221,#28222);
#24110=AXIS2_PLACEMENT_3D('',#47176,#28224,#28225);
#24111=AXIS2_PLACEMENT_3D('',#47177,#28226,#28227);
#24112=AXIS2_PLACEMENT_3D('',#47179,#28228,#28229);
#24113=AXIS2_PLACEMENT_3D('',#47181,#28230,#28231);
#24114=AXIS2_PLACEMENT_3D('',#47183,#28232,#28233);
#24115=AXIS2_PLACEMENT_3D('',#47185,#28234,#28235);
#24116=AXIS2_PLACEMENT_3D('',#47187,#28236,#28237);
#24117=AXIS2_PLACEMENT_3D('',#47189,#28238,#28239);
#24118=AXIS2_PLACEMENT_3D('',#47191,#28240,#28241);
#24119=AXIS2_PLACEMENT_3D('',#47192,#28242,#28243);
#24120=AXIS2_PLACEMENT_3D('',#47195,#28245,#28246);
#24121=AXIS2_PLACEMENT_3D('',#47196,#28247,#28248);
#24122=AXIS2_PLACEMENT_3D('',#47199,#28250,#28251);
#24123=AXIS2_PLACEMENT_3D('',#47200,#28252,#28253);
#24124=AXIS2_PLACEMENT_3D('',#47203,#28255,#28256);
#24125=AXIS2_PLACEMENT_3D('',#47204,#28257,#28258);
#24126=AXIS2_PLACEMENT_3D('',#47207,#28260,#28261);
#24127=AXIS2_PLACEMENT_3D('',#47208,#28262,#28263);
#24128=AXIS2_PLACEMENT_3D('',#47211,#28265,#28266);
#24129=AXIS2_PLACEMENT_3D('',#47212,#28267,#28268);
#24130=AXIS2_PLACEMENT_3D('',#47215,#28270,#28271);
#24131=AXIS2_PLACEMENT_3D('',#47216,#28272,#28273);
#24132=AXIS2_PLACEMENT_3D('',#47219,#28275,#28276);
#24133=AXIS2_PLACEMENT_3D('',#47220,#28277,#28278);
#24134=AXIS2_PLACEMENT_3D('',#47223,#28280,#28281);
#24135=AXIS2_PLACEMENT_3D('',#47224,#28282,#28283);
#24136=AXIS2_PLACEMENT_3D('',#47227,#28285,#28286);
#24137=AXIS2_PLACEMENT_3D('',#47228,#28287,#28288);
#24138=AXIS2_PLACEMENT_3D('',#47231,#28290,#28291);
#24139=AXIS2_PLACEMENT_3D('',#47232,#28292,#28293);
#24140=AXIS2_PLACEMENT_3D('',#47235,#28295,#28296);
#24141=AXIS2_PLACEMENT_3D('',#47236,#28297,#28298);
#24142=AXIS2_PLACEMENT_3D('',#47239,#28300,#28301);
#24143=AXIS2_PLACEMENT_3D('',#47242,#28303,#28304);
#24144=AXIS2_PLACEMENT_3D('',#47245,#28306,#28307);
#24145=AXIS2_PLACEMENT_3D('',#47248,#28309,#28310);
#24146=AXIS2_PLACEMENT_3D('',#47251,#28312,#28313);
#24147=AXIS2_PLACEMENT_3D('',#47254,#28315,#28316);
#24148=AXIS2_PLACEMENT_3D('',#47258,#28318,#28319);
#24149=AXIS2_PLACEMENT_3D('',#47259,#28320,#28321);
#24150=AXIS2_PLACEMENT_3D('',#47260,#28322,#28323);
#24151=AXIS2_PLACEMENT_3D('',#47262,#28324,#28325);
#24152=AXIS2_PLACEMENT_3D('',#47264,#28327,#28328);
#24153=AXIS2_PLACEMENT_3D('',#47265,#28329,#28330);
#24154=AXIS2_PLACEMENT_3D('',#47267,#28332,#28333);
#24155=AXIS2_PLACEMENT_3D('',#47269,#28334,#28335);
#24156=AXIS2_PLACEMENT_3D('',#47270,#28336,#28337);
#24157=AXIS2_PLACEMENT_3D('',#47273,#28339,#28340);
#24158=AXIS2_PLACEMENT_3D('',#47274,#28341,#28342);
#27551=DIRECTION('axis',(0.,0.,1.));
#27552=DIRECTION('refdir',(1.,0.,0.));
#27553=DIRECTION('',(0.,0.,-1.));
#27554=DIRECTION('',(0.,0.,-1.));
#27555=DIRECTION('',(0.,0.,-1.));
#27556=DIRECTION('',(0.,0.,-1.));
#27557=DIRECTION('',(0.,0.,-1.));
#27558=DIRECTION('',(0.,0.,-1.));
#27559=DIRECTION('',(0.,0.,-1.));
#27560=DIRECTION('',(0.,0.,-1.));
#27561=DIRECTION('',(0.,0.,-1.));
#27562=DIRECTION('',(0.,0.,-1.));
#27563=DIRECTION('center_axis',(-1.,0.,0.));
#27564=DIRECTION('ref_axis',(0.,1.,0.));
#27565=DIRECTION('',(0.,1.,0.));
#27566=DIRECTION('',(0.,1.,0.));
#27567=DIRECTION('',(0.,0.,-1.));
#27568=DIRECTION('',(0.,0.,-1.));
#27569=DIRECTION('',(0.,0.,-1.));
#27570=DIRECTION('center_axis',(1.,0.,0.));
#27571=DIRECTION('ref_axis',(0.,-1.,0.));
#27572=DIRECTION('',(0.,-1.,0.));
#27573=DIRECTION('',(0.,0.,-1.));
#27574=DIRECTION('',(0.,-1.,0.));
#27575=DIRECTION('',(0.,0.,-1.));
#27576=DIRECTION('',(0.,0.,-1.));
#27577=DIRECTION('',(0.,0.,-1.));
#27578=DIRECTION('',(0.,0.,-1.));
#27579=DIRECTION('',(0.,0.,-1.));
#27580=DIRECTION('',(0.,0.,-1.));
#27581=DIRECTION('',(0.,0.,-1.));
#27582=DIRECTION('center_axis',(-0.135112645952214,-0.990830244241561,0.));
#27583=DIRECTION('ref_axis',(-0.990830244241561,0.135112645952214,0.));
#27584=DIRECTION('',(-0.990830244241561,0.135112645952214,0.));
#27585=DIRECTION('',(0.,0.,-1.));
#27586=DIRECTION('',(-0.990830244241561,0.135112645952214,0.));
#27587=DIRECTION('',(0.,0.,-1.));
#27588=DIRECTION('',(0.,0.,-1.));
#27589=DIRECTION('',(0.,0.,-1.));
#27590=DIRECTION('',(0.,0.,-1.));
#27591=DIRECTION('',(0.,0.,-1.));
#27592=DIRECTION('',(0.,0.,-1.));
#27593=DIRECTION('',(0.,0.,-1.));
#27594=DIRECTION('',(0.,0.,-1.));
#27595=DIRECTION('',(0.,0.,-1.));
#27596=DIRECTION('',(0.,0.,-1.));
#27597=DIRECTION('',(0.,0.,-1.));
#27598=DIRECTION('',(0.,0.,-1.));
#27599=DIRECTION('',(0.,0.,-1.));
#27600=DIRECTION('',(0.,0.,-1.));
#27601=DIRECTION('',(0.,0.,-1.));
#27602=DIRECTION('center_axis',(-1.57407341770917E-15,-1.,0.));
#27603=DIRECTION('ref_axis',(-1.,1.57407341770917E-15,0.));
#27604=DIRECTION('',(-1.,1.57407341770917E-15,0.));
#27605=DIRECTION('',(-1.,1.57407341770917E-15,0.));
#27606=DIRECTION('center_axis',(0.,0.,1.));
#27607=DIRECTION('ref_axis',(1.,0.,0.));
#27608=DIRECTION('',(0.,0.,-1.));
#27609=DIRECTION('',(0.,0.,-1.));
#27610=DIRECTION('',(0.,0.,-1.));
#27611=DIRECTION('',(0.,0.,-1.));
#27612=DIRECTION('',(0.,0.,-1.));
#27613=DIRECTION('',(0.,0.,-1.));
#27614=DIRECTION('',(0.,0.,-1.));
#27615=DIRECTION('',(0.,0.,-1.));
#27616=DIRECTION('',(0.,0.,-1.));
#27617=DIRECTION('',(0.,0.,-1.));
#27618=DIRECTION('',(0.,0.,-1.));
#27619=DIRECTION('',(0.,0.,-1.));
#27620=DIRECTION('',(0.,0.,-1.));
#27621=DIRECTION('',(0.,0.,-1.));
#27622=DIRECTION('',(0.,0.,-1.));
#27623=DIRECTION('',(0.,0.,-1.));
#27624=DIRECTION('',(0.,0.,-1.));
#27625=DIRECTION('',(0.,0.,-1.));
#27626=DIRECTION('',(0.,0.,-1.));
#27627=DIRECTION('',(0.,0.,-1.));
#27628=DIRECTION('center_axis',(0.,0.,1.));
#27629=DIRECTION('ref_axis',(1.,0.,0.));
#27630=DIRECTION('',(0.,0.,-1.));
#27631=DIRECTION('',(0.,0.,-1.));
#27632=DIRECTION('',(0.,0.,-1.));
#27633=DIRECTION('center_axis',(-1.,0.,0.));
#27634=DIRECTION('ref_axis',(0.,1.,0.));
#27635=DIRECTION('',(0.,1.,0.));
#27636=DIRECTION('',(0.,0.,-1.));
#27637=DIRECTION('',(0.,1.,0.));
#27638=DIRECTION('',(0.,0.,-1.));
#27639=DIRECTION('',(0.,0.,-1.));
#27640=DIRECTION('center_axis',(-1.,0.,0.));
#27641=DIRECTION('ref_axis',(0.,1.,0.));
#27642=DIRECTION('',(0.,1.,0.));
#27643=DIRECTION('',(0.,0.,-1.));
#27644=DIRECTION('',(0.,1.,0.));
#27645=DIRECTION('center_axis',(0.,-1.,0.));
#27646=DIRECTION('ref_axis',(-1.,0.,0.));
#27647=DIRECTION('',(-1.,0.,0.));
#27648=DIRECTION('',(0.,0.,-1.));
#27649=DIRECTION('',(-1.,0.,0.));
#27650=DIRECTION('center_axis',(1.,0.,0.));
#27651=DIRECTION('ref_axis',(0.,-1.,0.));
#27652=DIRECTION('',(0.,-1.,0.));
#27653=DIRECTION('',(0.,0.,-1.));
#27654=DIRECTION('',(0.,-1.,0.));
#27655=DIRECTION('center_axis',(0.,1.,0.));
#27656=DIRECTION('ref_axis',(1.,0.,0.));
#27657=DIRECTION('',(1.,0.,0.));
#27658=DIRECTION('',(1.,0.,0.));
#27659=DIRECTION('center_axis',(0.,0.,1.));
#27660=DIRECTION('ref_axis',(1.,0.,0.));
#27661=DIRECTION('center_axis',(-0.946846713341944,-0.321685096691715,0.));
#27662=DIRECTION('ref_axis',(-0.321685096691715,0.946846713341944,0.));
#27663=DIRECTION('',(-0.321685096691715,0.946846713341944,0.));
#27664=DIRECTION('',(0.,0.,-1.));
#27665=DIRECTION('',(-0.321685096691715,0.946846713341944,0.));
#27666=DIRECTION('',(0.,0.,-1.));
#27667=DIRECTION('center_axis',(0.,-1.,0.));
#27668=DIRECTION('ref_axis',(-1.,0.,0.));
#27669=DIRECTION('',(-1.,0.,0.));
#27670=DIRECTION('',(0.,0.,-1.));
#27671=DIRECTION('',(-1.,0.,0.));
#27672=DIRECTION('center_axis',(0.944683612861939,-0.327983035521831,0.));
#27673=DIRECTION('ref_axis',(-0.327983035521831,-0.944683612861939,0.));
#27674=DIRECTION('',(-0.327983035521831,-0.944683612861939,0.));
#27675=DIRECTION('',(0.,0.,-1.));
#27676=DIRECTION('',(-0.327983035521831,-0.944683612861939,0.));
#27677=DIRECTION('center_axis',(-1.,0.,0.));
#27678=DIRECTION('ref_axis',(0.,1.,0.));
#27679=DIRECTION('',(0.,1.,0.));
#27680=DIRECTION('',(0.,0.,-1.));
#27681=DIRECTION('',(0.,1.,0.));
#27682=DIRECTION('center_axis',(0.,-1.,0.));
#27683=DIRECTION('ref_axis',(-1.,0.,0.));
#27684=DIRECTION('',(-1.,0.,0.));
#27685=DIRECTION('',(0.,0.,-1.));
#27686=DIRECTION('',(-1.,0.,0.));
#27687=DIRECTION('center_axis',(1.,0.,0.));
#27688=DIRECTION('ref_axis',(0.,-1.,0.));
#27689=DIRECTION('',(0.,-1.,0.));
#27690=DIRECTION('',(0.,0.,-1.));
#27691=DIRECTION('',(0.,-1.,0.));
#27692=DIRECTION('center_axis',(0.,1.,0.));
#27693=DIRECTION('ref_axis',(1.,0.,0.));
#27694=DIRECTION('',(1.,0.,0.));
#27695=DIRECTION('',(0.,0.,-1.));
#27696=DIRECTION('',(1.,0.,0.));
#27697=DIRECTION('center_axis',(-0.945579690186978,0.325390610660323,0.));
#27698=DIRECTION('ref_axis',(0.325390610660323,0.945579690186978,0.));
#27699=DIRECTION('',(0.325390610660323,0.945579690186978,0.));
#27700=DIRECTION('',(0.,0.,-1.));
#27701=DIRECTION('',(0.325390610660323,0.945579690186978,0.));
#27702=DIRECTION('',(0.,0.,-1.));
#27703=DIRECTION('',(0.,0.,-1.));
#27704=DIRECTION('center_axis',(0.948408837989887,0.317049958244238,0.));
#27705=DIRECTION('ref_axis',(0.317049958244238,-0.948408837989887,0.));
#27706=DIRECTION('',(0.317049958244238,-0.948408837989887,0.));
#27707=DIRECTION('',(0.,0.,-1.));
#27708=DIRECTION('',(0.317049958244238,-0.948408837989887,0.));
#27709=DIRECTION('center_axis',(0.,1.,0.));
#27710=DIRECTION('ref_axis',(1.,0.,0.));
#27711=DIRECTION('',(1.,0.,0.));
#27712=DIRECTION('',(0.,0.,-1.));
#27713=DIRECTION('',(1.,0.,0.));
#27714=DIRECTION('center_axis',(-1.,0.,0.));
#27715=DIRECTION('ref_axis',(0.,1.,0.));
#27716=DIRECTION('',(0.,1.,0.));
#27717=DIRECTION('',(0.,0.,-1.));
#27718=DIRECTION('',(0.,1.,0.));
#27719=DIRECTION('center_axis',(0.,-1.,0.));
#27720=DIRECTION('ref_axis',(-1.,0.,0.));
#27721=DIRECTION('',(-1.,0.,0.));
#27722=DIRECTION('',(0.,0.,-1.));
#27723=DIRECTION('',(-1.,0.,0.));
#27724=DIRECTION('center_axis',(1.,0.,0.));
#27725=DIRECTION('ref_axis',(0.,-1.,0.));
#27726=DIRECTION('',(0.,-1.,0.));
#27727=DIRECTION('',(0.,-1.,0.));
#27728=DIRECTION('center_axis',(0.,0.,1.));
#27729=DIRECTION('ref_axis',(1.,0.,0.));
#27730=DIRECTION('',(0.,0.,-1.));
#27731=DIRECTION('',(0.,0.,-1.));
#27732=DIRECTION('',(0.,0.,-1.));
#27733=DIRECTION('',(0.,0.,-1.));
#27734=DIRECTION('',(0.,0.,-1.));
#27735=DIRECTION('',(0.,0.,-1.));
#27736=DIRECTION('',(0.,0.,-1.));
#27737=DIRECTION('',(0.,0.,-1.));
#27738=DIRECTION('',(0.,0.,-1.));
#27739=DIRECTION('',(0.,0.,-1.));
#27740=DIRECTION('',(0.,0.,-1.));
#27741=DIRECTION('',(0.,0.,-1.));
#27742=DIRECTION('center_axis',(-0.175032773131272,-0.984562607623292,0.));
#27743=DIRECTION('ref_axis',(-0.984562607623292,0.175032773131272,0.));
#27744=DIRECTION('',(-0.984562607623292,0.175032773131272,0.));
#27745=DIRECTION('',(0.,0.,-1.));
#27746=DIRECTION('',(-0.984562607623292,0.175032773131272,0.));
#27747=DIRECTION('',(0.,0.,-1.));
#27748=DIRECTION('',(0.,0.,-1.));
#27749=DIRECTION('',(0.,0.,-1.));
#27750=DIRECTION('',(0.,0.,-1.));
#27751=DIRECTION('',(0.,0.,-1.));
#27752=DIRECTION('',(0.,0.,-1.));
#27753=DIRECTION('',(0.,0.,-1.));
#27754=DIRECTION('center_axis',(-0.992083762154323,0.125577899607075,0.));
#27755=DIRECTION('ref_axis',(0.125577899607075,0.992083762154323,0.));
#27756=DIRECTION('',(0.125577899607075,0.992083762154323,0.));
#27757=DIRECTION('',(0.,0.,-1.));
#27758=DIRECTION('',(0.125577899607075,0.992083762154323,0.));
#27759=DIRECTION('',(0.,0.,-1.));
#27760=DIRECTION('',(0.,0.,-1.));
#27761=DIRECTION('',(0.,0.,-1.));
#27762=DIRECTION('',(0.,0.,-1.));
#27763=DIRECTION('',(0.,0.,-1.));
#27764=DIRECTION('',(0.,0.,-1.));
#27765=DIRECTION('',(0.,0.,-1.));
#27766=DIRECTION('center_axis',(-0.132163748744578,0.99122789686216,0.));
#27767=DIRECTION('ref_axis',(0.99122789686216,0.132163748744578,0.));
#27768=DIRECTION('',(0.99122789686216,0.132163748744578,0.));
#27769=DIRECTION('',(0.,0.,-1.));
#27770=DIRECTION('',(0.99122789686216,0.132163748744578,0.));
#27771=DIRECTION('',(0.,0.,-1.));
#27772=DIRECTION('center_axis',(0.,0.,1.));
#27773=DIRECTION('ref_axis',(1.,0.,0.));
#27774=DIRECTION('center_axis',(0.,1.,0.));
#27775=DIRECTION('ref_axis',(1.,0.,0.));
#27776=DIRECTION('',(1.,0.,0.));
#27777=DIRECTION('',(0.,0.,-1.));
#27778=DIRECTION('',(1.,0.,0.));
#27779=DIRECTION('',(0.,0.,-1.));
#27780=DIRECTION('center_axis',(-1.,0.,0.));
#27781=DIRECTION('ref_axis',(0.,1.,0.));
#27782=DIRECTION('',(0.,1.,0.));
#27783=DIRECTION('',(0.,0.,-1.));
#27784=DIRECTION('',(0.,1.,0.));
#27785=DIRECTION('center_axis',(0.,-1.,0.));
#27786=DIRECTION('ref_axis',(-1.,0.,0.));
#27787=DIRECTION('',(-1.,0.,0.));
#27788=DIRECTION('',(0.,0.,-1.));
#27789=DIRECTION('',(-1.,0.,0.));
#27790=DIRECTION('center_axis',(1.,0.,0.));
#27791=DIRECTION('ref_axis',(0.,-1.,0.));
#27792=DIRECTION('',(0.,-1.,0.));
#27793=DIRECTION('',(0.,-1.,0.));
#27794=DIRECTION('center_axis',(0.,0.,-1.));
#27795=DIRECTION('ref_axis',(-1.,0.,0.));
#27796=DIRECTION('',(0.,0.,-1.));
#27797=DIRECTION('',(0.,0.,-1.));
#27798=DIRECTION('',(0.,0.,-1.));
#27799=DIRECTION('center_axis',(-0.935759711779643,-0.352638287498792,0.));
#27800=DIRECTION('ref_axis',(-0.352638287498792,0.935759711779643,0.));
#27801=DIRECTION('',(-0.352638287498792,0.935759711779643,0.));
#27802=DIRECTION('',(0.,0.,-1.));
#27803=DIRECTION('',(-0.352638287498792,0.935759711779643,0.));
#27804=DIRECTION('center_axis',(0.,1.,0.));
#27805=DIRECTION('ref_axis',(1.,0.,0.));
#27806=DIRECTION('',(1.,0.,0.));
#27807=DIRECTION('',(0.,0.,-1.));
#27808=DIRECTION('',(1.,0.,0.));
#27809=DIRECTION('center_axis',(0.936507962144564,-0.35064631302758,0.));
#27810=DIRECTION('ref_axis',(-0.35064631302758,-0.936507962144564,0.));
#27811=DIRECTION('',(-0.35064631302758,-0.936507962144564,0.));
#27812=DIRECTION('',(-0.35064631302758,-0.936507962144564,0.));
#27813=DIRECTION('center_axis',(0.,-1.,0.));
#27814=DIRECTION('ref_axis',(-1.,0.,0.));
#27815=DIRECTION('',(-1.,0.,0.));
#27816=DIRECTION('',(0.,0.,-1.));
#27817=DIRECTION('',(-1.,0.,0.));
#27818=DIRECTION('',(0.,0.,-1.));
#27819=DIRECTION('center_axis',(-0.933183037129681,-0.359401473582713,0.));
#27820=DIRECTION('ref_axis',(-0.359401473582713,0.933183037129681,0.));
#27821=DIRECTION('',(-0.359401473582713,0.933183037129681,0.));
#27822=DIRECTION('',(0.,0.,-1.));
#27823=DIRECTION('',(-0.359401473582713,0.933183037129681,0.));
#27824=DIRECTION('center_axis',(0.,-1.,0.));
#27825=DIRECTION('ref_axis',(-1.,0.,0.));
#27826=DIRECTION('',(-1.,0.,0.));
#27827=DIRECTION('',(0.,0.,-1.));
#27828=DIRECTION('',(-1.,0.,0.));
#27829=DIRECTION('center_axis',(0.925486618796678,0.378780303643539,0.));
#27830=DIRECTION('ref_axis',(0.378780303643539,-0.925486618796678,0.));
#27831=DIRECTION('',(0.378780303643539,-0.925486618796678,0.));
#27832=DIRECTION('',(0.,0.,-1.));
#27833=DIRECTION('',(0.378780303643539,-0.925486618796678,0.));
#27834=DIRECTION('center_axis',(0.,1.,0.));
#27835=DIRECTION('ref_axis',(1.,0.,0.));
#27836=DIRECTION('',(1.,0.,0.));
#27837=DIRECTION('',(0.,0.,-1.));
#27838=DIRECTION('',(1.,0.,0.));
#27839=DIRECTION('center_axis',(-0.93352603941556,0.35850960061496,0.));
#27840=DIRECTION('ref_axis',(0.35850960061496,0.93352603941556,0.));
#27841=DIRECTION('',(0.35850960061496,0.93352603941556,0.));
#27842=DIRECTION('',(0.,0.,-1.));
#27843=DIRECTION('',(0.35850960061496,0.93352603941556,0.));
#27844=DIRECTION('center_axis',(0.,-1.,0.));
#27845=DIRECTION('ref_axis',(-1.,0.,0.));
#27846=DIRECTION('',(-1.,0.,0.));
#27847=DIRECTION('',(0.,0.,-1.));
#27848=DIRECTION('',(-1.,0.,0.));
#27849=DIRECTION('center_axis',(0.940102154683871,-0.340892855247427,0.));
#27850=DIRECTION('ref_axis',(-0.340892855247427,-0.940102154683871,0.));
#27851=DIRECTION('',(-0.340892855247427,-0.940102154683871,0.));
#27852=DIRECTION('',(-0.340892855247427,-0.940102154683871,0.));
#27853=DIRECTION('center_axis',(0.,0.,1.));
#27854=DIRECTION('ref_axis',(1.,0.,0.));
#27855=DIRECTION('',(0.,0.,-1.));
#27856=DIRECTION('',(0.,0.,-1.));
#27857=DIRECTION('',(0.,0.,-1.));
#27858=DIRECTION('',(0.,0.,-1.));
#27859=DIRECTION('',(0.,0.,-1.));
#27860=DIRECTION('',(0.,0.,-1.));
#27861=DIRECTION('',(0.,0.,-1.));
#27862=DIRECTION('',(0.,0.,-1.));
#27863=DIRECTION('',(0.,0.,-1.));
#27864=DIRECTION('',(0.,0.,-1.));
#27865=DIRECTION('',(0.,0.,-1.));
#27866=DIRECTION('',(0.,0.,-1.));
#27867=DIRECTION('',(0.,0.,-1.));
#27868=DIRECTION('',(0.,0.,-1.));
#27869=DIRECTION('center_axis',(0.0750566189565801,-0.99717927372705,0.));
#27870=DIRECTION('ref_axis',(-0.99717927372705,-0.0750566189565801,0.));
#27871=DIRECTION('',(-0.99717927372705,-0.0750566189565801,0.));
#27872=DIRECTION('',(0.,0.,-1.));
#27873=DIRECTION('',(-0.99717927372705,-0.0750566189565801,0.));
#27874=DIRECTION('',(0.,0.,-1.));
#27875=DIRECTION('',(0.,0.,-1.));
#27876=DIRECTION('',(0.,0.,-1.));
#27877=DIRECTION('',(0.,0.,-1.));
#27878=DIRECTION('',(0.,0.,-1.));
#27879=DIRECTION('',(0.,0.,-1.));
#27880=DIRECTION('',(0.,0.,-1.));
#27881=DIRECTION('',(0.,0.,-1.));
#27882=DIRECTION('',(0.,0.,-1.));
#27883=DIRECTION('',(0.,0.,-1.));
#27884=DIRECTION('',(0.,0.,-1.));
#27885=DIRECTION('',(0.,0.,-1.));
#27886=DIRECTION('',(0.,0.,-1.));
#27887=DIRECTION('',(0.,0.,-1.));
#27888=DIRECTION('',(0.,0.,-1.));
#27889=DIRECTION('',(0.,0.,-1.));
#27890=DIRECTION('',(0.,0.,-1.));
#27891=DIRECTION('',(0.,0.,-1.));
#27892=DIRECTION('center_axis',(-0.0870993597080284,0.996199629360728,0.));
#27893=DIRECTION('ref_axis',(0.996199629360728,0.0870993597080284,0.));
#27894=DIRECTION('',(0.996199629360728,0.0870993597080284,0.));
#27895=DIRECTION('',(0.,0.,-1.));
#27896=DIRECTION('',(0.996199629360728,0.0870993597080284,0.));
#27897=DIRECTION('',(0.,0.,-1.));
#27898=DIRECTION('center_axis',(0.,0.,1.));
#27899=DIRECTION('ref_axis',(1.,0.,0.));
#27900=DIRECTION('',(0.,0.,-1.));
#27901=DIRECTION('',(0.,0.,-1.));
#27902=DIRECTION('',(0.,0.,-1.));
#27903=DIRECTION('',(0.,0.,-1.));
#27904=DIRECTION('',(0.,0.,-1.));
#27905=DIRECTION('',(0.,0.,-1.));
#27906=DIRECTION('',(0.,0.,-1.));
#27907=DIRECTION('',(0.,0.,-1.));
#27908=DIRECTION('',(0.,0.,-1.));
#27909=DIRECTION('',(0.,0.,-1.));
#27910=DIRECTION('',(0.,0.,-1.));
#27911=DIRECTION('',(0.,0.,-1.));
#27912=DIRECTION('center_axis',(-0.175032773131272,-0.984562607623292,0.));
#27913=DIRECTION('ref_axis',(-0.984562607623292,0.175032773131272,0.));
#27914=DIRECTION('',(-0.984562607623292,0.175032773131272,0.));
#27915=DIRECTION('',(0.,0.,-1.));
#27916=DIRECTION('',(-0.984562607623292,0.175032773131272,0.));
#27917=DIRECTION('',(0.,0.,-1.));
#27918=DIRECTION('',(0.,0.,-1.));
#27919=DIRECTION('',(0.,0.,-1.));
#27920=DIRECTION('',(0.,0.,-1.));
#27921=DIRECTION('',(0.,0.,-1.));
#27922=DIRECTION('',(0.,0.,-1.));
#27923=DIRECTION('',(0.,0.,-1.));
#27924=DIRECTION('center_axis',(-0.992083762154323,0.125577899607073,0.));
#27925=DIRECTION('ref_axis',(0.125577899607073,0.992083762154323,0.));
#27926=DIRECTION('',(0.125577899607073,0.992083762154323,0.));
#27927=DIRECTION('',(0.,0.,-1.));
#27928=DIRECTION('',(0.125577899607073,0.992083762154323,0.));
#27929=DIRECTION('',(0.,0.,-1.));
#27930=DIRECTION('',(0.,0.,-1.));
#27931=DIRECTION('',(0.,0.,-1.));
#27932=DIRECTION('',(0.,0.,-1.));
#27933=DIRECTION('',(0.,0.,-1.));
#27934=DIRECTION('',(0.,0.,-1.));
#27935=DIRECTION('',(0.,0.,-1.));
#27936=DIRECTION('center_axis',(-0.132163748744578,0.99122789686216,0.));
#27937=DIRECTION('ref_axis',(0.99122789686216,0.132163748744578,0.));
#27938=DIRECTION('',(0.99122789686216,0.132163748744578,0.));
#27939=DIRECTION('',(0.,0.,-1.));
#27940=DIRECTION('',(0.99122789686216,0.132163748744578,0.));
#27941=DIRECTION('',(0.,0.,-1.));
#27942=DIRECTION('center_axis',(0.,0.,1.));
#27943=DIRECTION('ref_axis',(1.,0.,0.));
#27944=DIRECTION('',(0.,0.,-1.));
#27945=DIRECTION('',(0.,0.,-1.));
#27946=DIRECTION('',(0.,0.,-1.));
#27947=DIRECTION('',(0.,0.,-1.));
#27948=DIRECTION('',(0.,0.,-1.));
#27949=DIRECTION('',(0.,0.,-1.));
#27950=DIRECTION('',(0.,0.,-1.));
#27951=DIRECTION('',(0.,0.,-1.));
#27952=DIRECTION('',(0.,0.,-1.));
#27953=DIRECTION('center_axis',(-0.102165340737178,-0.994767431690471,0.));
#27954=DIRECTION('ref_axis',(-0.994767431690471,0.102165340737178,0.));
#27955=DIRECTION('',(-0.994767431690471,0.102165340737178,0.));
#27956=DIRECTION('',(0.,0.,-1.));
#27957=DIRECTION('',(-0.994767431690471,0.102165340737178,0.));
#27958=DIRECTION('',(0.,0.,-1.));
#27959=DIRECTION('',(0.,0.,-1.));
#27960=DIRECTION('',(0.,0.,-1.));
#27961=DIRECTION('',(0.,0.,-1.));
#27962=DIRECTION('',(0.,0.,-1.));
#27963=DIRECTION('',(0.,0.,-1.));
#27964=DIRECTION('',(0.,0.,-1.));
#27965=DIRECTION('',(0.,0.,-1.));
#27966=DIRECTION('',(0.,0.,-1.));
#27967=DIRECTION('center_axis',(0.,-1.,0.));
#27968=DIRECTION('ref_axis',(-1.,0.,0.));
#27969=DIRECTION('',(-1.,0.,0.));
#27970=DIRECTION('',(0.,0.,-1.));
#27971=DIRECTION('',(-1.,0.,0.));
#27972=DIRECTION('center_axis',(1.,0.,0.));
#27973=DIRECTION('ref_axis',(0.,-1.,0.));
#27974=DIRECTION('',(0.,-1.,0.));
#27975=DIRECTION('',(0.,0.,-1.));
#27976=DIRECTION('',(0.,-1.,0.));
#27977=DIRECTION('center_axis',(-1.0289465542069E-16,1.,0.));
#27978=DIRECTION('ref_axis',(1.,1.0289465542069E-16,0.));
#27979=DIRECTION('',(1.,1.0289465542069E-16,0.));
#27980=DIRECTION('',(0.,0.,-1.));
#27981=DIRECTION('',(1.,1.0289465542069E-16,0.));
#27982=DIRECTION('center_axis',(0.,0.,1.));
#27983=DIRECTION('ref_axis',(1.,0.,0.));
#27984=DIRECTION('center_axis',(0.,-1.,0.));
#27985=DIRECTION('ref_axis',(-1.,0.,0.));
#27986=DIRECTION('',(-1.,0.,0.));
#27987=DIRECTION('',(0.,0.,-1.));
#27988=DIRECTION('',(-1.,0.,0.));
#27989=DIRECTION('',(0.,0.,-1.));
#27990=DIRECTION('',(0.,0.,-1.));
#27991=DIRECTION('',(0.,0.,-1.));
#27992=DIRECTION('',(0.,0.,-1.));
#27993=DIRECTION('',(0.,0.,-1.));
#27994=DIRECTION('',(0.,0.,-1.));
#27995=DIRECTION('center_axis',(0.,1.,0.));
#27996=DIRECTION('ref_axis',(1.,0.,0.));
#27997=DIRECTION('',(1.,0.,0.));
#27998=DIRECTION('',(0.,0.,-1.));
#27999=DIRECTION('',(1.,0.,0.));
#28000=DIRECTION('center_axis',(1.,0.,0.));
#28001=DIRECTION('ref_axis',(0.,-1.,0.));
#28002=DIRECTION('',(0.,-1.,0.));
#28003=DIRECTION('',(0.,-1.,0.));
#28004=DIRECTION('center_axis',(0.,-1.,0.));
#28005=DIRECTION('ref_axis',(-1.,0.,0.));
#28006=DIRECTION('',(-1.,0.,0.));
#28007=DIRECTION('',(0.,0.,-1.));
#28008=DIRECTION('',(-1.,0.,0.));
#28009=DIRECTION('',(0.,0.,-1.));
#28010=DIRECTION('',(0.,0.,-1.));
#28011=DIRECTION('',(0.,0.,-1.));
#28012=DIRECTION('',(0.,0.,-1.));
#28013=DIRECTION('',(0.,0.,-1.));
#28014=DIRECTION('',(0.,0.,-1.));
#28015=DIRECTION('',(0.,0.,-1.));
#28016=DIRECTION('center_axis',(0.,1.,0.));
#28017=DIRECTION('ref_axis',(1.,0.,0.));
#28018=DIRECTION('',(1.,0.,0.));
#28019=DIRECTION('',(0.,0.,-1.));
#28020=DIRECTION('',(1.,0.,0.));
#28021=DIRECTION('center_axis',(-1.,0.,0.));
#28022=DIRECTION('ref_axis',(0.,1.,0.));
#28023=DIRECTION('',(0.,1.,0.));
#28024=DIRECTION('',(0.,0.,-1.));
#28025=DIRECTION('',(0.,1.,0.));
#28026=DIRECTION('center_axis',(0.,-1.,0.));
#28027=DIRECTION('ref_axis',(-1.,0.,0.));
#28028=DIRECTION('',(-1.,0.,0.));
#28029=DIRECTION('',(0.,0.,-1.));
#28030=DIRECTION('',(-1.,0.,0.));
#28031=DIRECTION('center_axis',(1.,0.,0.));
#28032=DIRECTION('ref_axis',(0.,-1.,0.));
#28033=DIRECTION('',(0.,-1.,0.));
#28034=DIRECTION('',(0.,-1.,0.));
#28035=DIRECTION('center_axis',(0.,0.,1.));
#28036=DIRECTION('ref_axis',(1.,0.,0.));
#28037=DIRECTION('',(0.,0.,-1.));
#28038=DIRECTION('',(0.,0.,-1.));
#28039=DIRECTION('',(0.,0.,-1.));
#28040=DIRECTION('',(0.,0.,-1.));
#28041=DIRECTION('',(0.,0.,-1.));
#28042=DIRECTION('',(0.,0.,-1.));
#28043=DIRECTION('',(0.,0.,-1.));
#28044=DIRECTION('',(0.,0.,-1.));
#28045=DIRECTION('',(0.,0.,-1.));
#28046=DIRECTION('',(0.,0.,-1.));
#28047=DIRECTION('',(0.,0.,-1.));
#28048=DIRECTION('',(0.,0.,-1.));
#28049=DIRECTION('',(0.,0.,-1.));
#28050=DIRECTION('',(0.,0.,-1.));
#28051=DIRECTION('',(0.,0.,-1.));
#28052=DIRECTION('',(0.,0.,-1.));
#28053=DIRECTION('',(0.,0.,-1.));
#28054=DIRECTION('',(0.,0.,-1.));
#28055=DIRECTION('',(0.,0.,-1.));
#28056=DIRECTION('',(0.,0.,-1.));
#28057=DIRECTION('',(0.,0.,-1.));
#28058=DIRECTION('',(0.,0.,-1.));
#28059=DIRECTION('',(0.,0.,-1.));
#28060=DIRECTION('',(0.,0.,-1.));
#28061=DIRECTION('',(0.,0.,-1.));
#28062=DIRECTION('',(0.,0.,-1.));
#28063=DIRECTION('center_axis',(0.0779744070100615,-0.996955361012432,0.));
#28064=DIRECTION('ref_axis',(-0.996955361012432,-0.0779744070100615,0.));
#28065=DIRECTION('',(-0.996955361012432,-0.0779744070100615,0.));
#28066=DIRECTION('',(0.,0.,-1.));
#28067=DIRECTION('',(-0.996955361012432,-0.0779744070100615,0.));
#28068=DIRECTION('',(0.,0.,-1.));
#28069=DIRECTION('center_axis',(0.,0.,1.));
#28070=DIRECTION('ref_axis',(1.,0.,0.));
#28071=DIRECTION('',(0.,0.,-1.));
#28072=DIRECTION('',(0.,0.,-1.));
#28073=DIRECTION('',(0.,0.,-1.));
#28074=DIRECTION('',(0.,0.,-1.));
#28075=DIRECTION('',(0.,0.,-1.));
#28076=DIRECTION('',(0.,0.,-1.));
#28077=DIRECTION('',(0.,0.,-1.));
#28078=DIRECTION('',(0.,0.,-1.));
#28079=DIRECTION('',(0.,0.,-1.));
#28080=DIRECTION('',(0.,0.,-1.));
#28081=DIRECTION('',(0.,0.,-1.));
#28082=DIRECTION('',(0.,0.,-1.));
#28083=DIRECTION('',(0.,0.,-1.));
#28084=DIRECTION('',(0.,0.,-1.));
#28085=DIRECTION('',(0.,0.,-1.));
#28086=DIRECTION('',(0.,0.,-1.));
#28087=DIRECTION('center_axis',(1.,0.,0.));
#28088=DIRECTION('ref_axis',(0.,-1.,0.));
#28089=DIRECTION('',(0.,-1.,0.));
#28090=DIRECTION('',(0.,0.,-1.));
#28091=DIRECTION('',(0.,-1.,0.));
#28092=DIRECTION('center_axis',(0.,1.,0.));
#28093=DIRECTION('ref_axis',(1.,0.,0.));
#28094=DIRECTION('',(1.,0.,0.));
#28095=DIRECTION('',(0.,0.,-1.));
#28096=DIRECTION('',(1.,0.,0.));
#28097=DIRECTION('center_axis',(-1.,0.,0.));
#28098=DIRECTION('ref_axis',(0.,1.,0.));
#28099=DIRECTION('',(0.,1.,0.));
#28100=DIRECTION('',(0.,0.,-1.));
#28101=DIRECTION('',(0.,1.,0.));
#28102=DIRECTION('center_axis',(0.,-1.,0.));
#28103=DIRECTION('ref_axis',(-1.,0.,0.));
#28104=DIRECTION('',(-1.,0.,0.));
#28105=DIRECTION('',(0.,0.,-1.));
#28106=DIRECTION('',(-1.,0.,0.));
#28107=DIRECTION('center_axis',(1.,0.,0.));
#28108=DIRECTION('ref_axis',(0.,-1.,0.));
#28109=DIRECTION('',(0.,-1.,0.));
#28110=DIRECTION('',(0.,0.,-1.));
#28111=DIRECTION('',(0.,-1.,0.));
#28112=DIRECTION('center_axis',(0.,0.,1.));
#28113=DIRECTION('ref_axis',(1.,0.,0.));
#28114=DIRECTION('',(0.,0.,-1.));
#28115=DIRECTION('',(0.,0.,-1.));
#28116=DIRECTION('',(0.,0.,-1.));
#28117=DIRECTION('',(0.,0.,-1.));
#28118=DIRECTION('',(0.,0.,-1.));
#28119=DIRECTION('center_axis',(0.937477410285731,-0.348046125109819,0.));
#28120=DIRECTION('ref_axis',(-0.348046125109819,-0.937477410285731,0.));
#28121=DIRECTION('',(-0.348046125109819,-0.937477410285731,0.));
#28122=DIRECTION('',(0.,0.,-1.));
#28123=DIRECTION('',(-0.348046125109819,-0.937477410285731,0.));
#28124=DIRECTION('',(0.,0.,-1.));
#28125=DIRECTION('',(0.,0.,-1.));
#28126=DIRECTION('',(0.,0.,-1.));
#28127=DIRECTION('center_axis',(1.,0.,0.));
#28128=DIRECTION('ref_axis',(0.,-1.,0.));
#28129=DIRECTION('',(0.,-1.,0.));
#28130=DIRECTION('',(0.,0.,-1.));
#28131=DIRECTION('',(0.,-1.,0.));
#28132=DIRECTION('center_axis',(0.,1.,0.));
#28133=DIRECTION('ref_axis',(1.,0.,0.));
#28134=DIRECTION('',(1.,0.,0.));
#28135=DIRECTION('',(0.,0.,-1.));
#28136=DIRECTION('',(1.,0.,0.));
#28137=DIRECTION('center_axis',(-1.,0.,0.));
#28138=DIRECTION('ref_axis',(0.,1.,0.));
#28139=DIRECTION('',(0.,1.,0.));
#28140=DIRECTION('',(0.,0.,-1.));
#28141=DIRECTION('',(0.,1.,0.));
#28142=DIRECTION('center_axis',(0.,-1.,0.));
#28143=DIRECTION('ref_axis',(-1.,0.,0.));
#28144=DIRECTION('',(-1.,0.,0.));
#28145=DIRECTION('',(0.,0.,-1.));
#28146=DIRECTION('',(-1.,0.,0.));
#28147=DIRECTION('center_axis',(1.,0.,0.));
#28148=DIRECTION('ref_axis',(0.,-1.,0.));
#28149=DIRECTION('',(0.,-1.,0.));
#28150=DIRECTION('',(0.,-1.,0.));
#28151=DIRECTION('center_axis',(0.,0.,1.));
#28152=DIRECTION('ref_axis',(1.,0.,0.));
#28153=DIRECTION('center_axis',(0.,0.,1.));
#28154=DIRECTION('ref_axis',(1.,0.,0.));
#28155=DIRECTION('center_axis',(0.,0.,1.));
#28156=DIRECTION('ref_axis',(1.,0.,0.));
#28157=DIRECTION('center_axis',(0.,0.,1.));
#28158=DIRECTION('ref_axis',(1.,0.,0.));
#28159=DIRECTION('center_axis',(0.,0.,1.));
#28160=DIRECTION('ref_axis',(1.,0.,0.));
#28161=DIRECTION('center_axis',(0.,0.,1.));
#28162=DIRECTION('ref_axis',(1.,0.,0.));
#28163=DIRECTION('center_axis',(0.,0.,1.));
#28164=DIRECTION('ref_axis',(1.,0.,0.));
#28165=DIRECTION('center_axis',(0.,0.,1.));
#28166=DIRECTION('ref_axis',(1.,0.,0.));
#28167=DIRECTION('center_axis',(0.,0.,1.));
#28168=DIRECTION('ref_axis',(1.,0.,0.));
#28169=DIRECTION('',(0.,0.,1.));
#28170=DIRECTION('center_axis',(0.,1.,0.));
#28171=DIRECTION('ref_axis',(0.,0.,1.));
#28172=DIRECTION('center_axis',(0.,1.,0.));
#28173=DIRECTION('ref_axis',(0.,0.,1.));
#28174=DIRECTION('',(8.65956056235493E-17,-0.707106781186548,0.707106781186548));
#28175=DIRECTION('center_axis',(0.,-1.,0.));
#28176=DIRECTION('ref_axis',(0.,0.,1.));
#28177=DIRECTION('center_axis',(0.,1.,0.));
#28178=DIRECTION('ref_axis',(0.,0.,1.));
#28179=DIRECTION('center_axis',(0.,1.,0.));
#28180=DIRECTION('ref_axis',(1.,0.,0.));
#28181=DIRECTION('',(0.,1.,0.));
#28182=DIRECTION('center_axis',(0.,1.,0.));
#28183=DIRECTION('ref_axis',(1.,0.,0.));
#28184=DIRECTION('',(0.,0.,-1.));
#28185=DIRECTION('',(0.,0.,1.));
#28186=DIRECTION('',(1.,0.,0.));
#28187=DIRECTION('center_axis',(0.,1.,0.));
#28188=DIRECTION('ref_axis',(0.,0.,1.));
#28189=DIRECTION('',(-1.04972719113862E-16,0.515038074910054,-0.857167300702112));
#28190=DIRECTION('center_axis',(0.,1.,0.));
#28191=DIRECTION('ref_axis',(1.,0.,0.));
#28192=DIRECTION('center_axis',(0.,1.,0.));
#28193=DIRECTION('ref_axis',(0.,0.,1.));
#28194=DIRECTION('',(0.,1.,0.));
#28195=DIRECTION('',(0.,1.,0.));
#28196=DIRECTION('center_axis',(0.,1.,0.));
#28197=DIRECTION('ref_axis',(1.,0.,0.));
#28198=DIRECTION('center_axis',(0.,-1.,0.));
#28199=DIRECTION('ref_axis',(0.,0.,-1.));
#28200=DIRECTION('center_axis',(0.,0.,-1.));
#28201=DIRECTION('ref_axis',(-1.,0.,0.));
#28202=DIRECTION('center_axis',(0.,0.,-1.));
#28203=DIRECTION('ref_axis',(1.,0.,0.));
#28204=DIRECTION('center_axis',(0.,0.,1.));
#28205=DIRECTION('ref_axis',(1.,0.,0.));
#28206=DIRECTION('center_axis',(0.,0.,1.));
#28207=DIRECTION('ref_axis',(-1.,1.22464679914735E-16,0.));
#28208=DIRECTION('',(0.,0.,-1.));
#28209=DIRECTION('center_axis',(0.,0.,1.));
#28210=DIRECTION('ref_axis',(1.,0.,0.));
#28211=DIRECTION('center_axis',(0.,0.,1.));
#28212=DIRECTION('ref_axis',(-1.,1.22464679914735E-16,0.));
#28213=DIRECTION('center_axis',(0.,0.,1.));
#28214=DIRECTION('ref_axis',(1.,0.,0.));
#28215=DIRECTION('center_axis',(0.,0.,-1.));
#28216=DIRECTION('ref_axis',(-1.,1.22464679914735E-16,0.));
#28217=DIRECTION('center_axis',(1.22464679914735E-16,-1.,0.));
#28218=DIRECTION('ref_axis',(-1.,-1.22464679914735E-16,0.));
#28219=DIRECTION('center_axis',(0.,0.,-1.));
#28220=DIRECTION('ref_axis',(1.,0.,0.));
#28221=DIRECTION('center_axis',(0.,0.,-1.));
#28222=DIRECTION('ref_axis',(1.,0.,0.));
#28223=DIRECTION('',(0.707106781186548,-8.65956056235493E-17,0.707106781186548));
#28224=DIRECTION('center_axis',(0.,0.,1.));
#28225=DIRECTION('ref_axis',(1.,0.,0.));
#28226=DIRECTION('center_axis',(0.,0.,-1.));
#28227=DIRECTION('ref_axis',(-1.,0.,0.));
#28228=DIRECTION('center_axis',(0.,0.,1.));
#28229=DIRECTION('ref_axis',(1.,0.,0.));
#28230=DIRECTION('center_axis',(0.,0.,-1.));
#28231=DIRECTION('ref_axis',(1.,0.,0.));
#28232=DIRECTION('center_axis',(0.,0.,-1.));
#28233=DIRECTION('ref_axis',(1.,0.,0.));
#28234=DIRECTION('center_axis',(0.,0.,-1.));
#28235=DIRECTION('ref_axis',(-1.,0.,0.));
#28236=DIRECTION('center_axis',(0.,0.,-1.));
#28237=DIRECTION('ref_axis',(1.,0.,0.));
#28238=DIRECTION('center_axis',(0.,0.,-1.));
#28239=DIRECTION('ref_axis',(1.,0.,0.));
#28240=DIRECTION('center_axis',(0.,0.,-1.));
#28241=DIRECTION('ref_axis',(1.,0.,0.));
#28242=DIRECTION('center_axis',(0.,0.,1.));
#28243=DIRECTION('ref_axis',(1.,0.,0.));
#28244=DIRECTION('',(0.,0.,1.));
#28245=DIRECTION('center_axis',(0.,0.,1.));
#28246=DIRECTION('ref_axis',(1.,0.,0.));
#28247=DIRECTION('center_axis',(0.,0.,-1.));
#28248=DIRECTION('ref_axis',(1.,0.,0.));
#28249=DIRECTION('',(0.707106781186548,-8.65956056235493E-17,0.707106781186548));
#28250=DIRECTION('center_axis',(0.,0.,1.));
#28251=DIRECTION('ref_axis',(1.,0.,0.));
#28252=DIRECTION('center_axis',(0.,0.,1.));
#28253=DIRECTION('ref_axis',(1.,0.,0.));
#28254=DIRECTION('',(0.,0.,1.));
#28255=DIRECTION('center_axis',(0.,0.,1.));
#28256=DIRECTION('ref_axis',(1.,0.,0.));
#28257=DIRECTION('center_axis',(0.,0.,-1.));
#28258=DIRECTION('ref_axis',(1.,0.,0.));
#28259=DIRECTION('',(0.707106781186547,-8.65956056235493E-17,0.707106781186547));
#28260=DIRECTION('center_axis',(0.,0.,1.));
#28261=DIRECTION('ref_axis',(1.,0.,0.));
#28262=DIRECTION('center_axis',(0.,0.,1.));
#28263=DIRECTION('ref_axis',(1.,0.,0.));
#28264=DIRECTION('',(0.,0.,1.));
#28265=DIRECTION('center_axis',(0.,0.,1.));
#28266=DIRECTION('ref_axis',(1.,0.,0.));
#28267=DIRECTION('center_axis',(0.,0.,-1.));
#28268=DIRECTION('ref_axis',(1.,0.,0.));
#28269=DIRECTION('',(0.707106781186548,-8.65956056235493E-17,0.707106781186548));
#28270=DIRECTION('center_axis',(0.,0.,1.));
#28271=DIRECTION('ref_axis',(1.,0.,0.));
#28272=DIRECTION('center_axis',(0.,0.,1.));
#28273=DIRECTION('ref_axis',(1.,0.,0.));
#28274=DIRECTION('',(0.,0.,1.));
#28275=DIRECTION('center_axis',(0.,0.,1.));
#28276=DIRECTION('ref_axis',(1.,0.,0.));
#28277=DIRECTION('center_axis',(0.,0.,-1.));
#28278=DIRECTION('ref_axis',(1.,0.,0.));
#28279=DIRECTION('',(0.707106781186548,-8.65956056235493E-17,0.707106781186548));
#28280=DIRECTION('center_axis',(0.,0.,1.));
#28281=DIRECTION('ref_axis',(1.,0.,0.));
#28282=DIRECTION('center_axis',(0.,0.,1.));
#28283=DIRECTION('ref_axis',(1.,0.,0.));
#28284=DIRECTION('',(0.,0.,1.));
#28285=DIRECTION('center_axis',(0.,0.,1.));
#28286=DIRECTION('ref_axis',(1.,0.,0.));
#28287=DIRECTION('center_axis',(0.,0.,-1.));
#28288=DIRECTION('ref_axis',(1.,0.,0.));
#28289=DIRECTION('',(0.707106781186548,-8.65956056235493E-17,0.707106781186548));
#28290=DIRECTION('center_axis',(0.,0.,1.));
#28291=DIRECTION('ref_axis',(1.,0.,0.));
#28292=DIRECTION('center_axis',(0.,0.,1.));
#28293=DIRECTION('ref_axis',(1.,0.,0.));
#28294=DIRECTION('',(0.,0.,1.));
#28295=DIRECTION('center_axis',(0.,0.,1.));
#28296=DIRECTION('ref_axis',(1.,0.,0.));
#28297=DIRECTION('center_axis',(0.,0.,-1.));
#28298=DIRECTION('ref_axis',(1.,0.,0.));
#28299=DIRECTION('',(0.857167300702112,1.04972719113862E-16,0.515038074910054));
#28300=DIRECTION('center_axis',(0.,0.,-1.));
#28301=DIRECTION('ref_axis',(1.,0.,0.));
#28302=DIRECTION('',(0.857167300702112,1.04972719113862E-16,0.515038074910054));
#28303=DIRECTION('center_axis',(0.,0.,-1.));
#28304=DIRECTION('ref_axis',(1.,0.,0.));
#28305=DIRECTION('',(0.857167300702112,1.04972719113862E-16,0.515038074910054));
#28306=DIRECTION('center_axis',(0.,0.,-1.));
#28307=DIRECTION('ref_axis',(1.,0.,0.));
#28308=DIRECTION('',(0.857167300702113,1.04972719113862E-16,0.515038074910053));
#28309=DIRECTION('center_axis',(0.,0.,-1.));
#28310=DIRECTION('ref_axis',(1.,0.,0.));
#28311=DIRECTION('',(0.857167300702112,1.04972719113862E-16,0.515038074910054));
#28312=DIRECTION('center_axis',(0.,0.,-1.));
#28313=DIRECTION('ref_axis',(1.,0.,0.));
#28314=DIRECTION('',(0.857167300702112,1.04972719113862E-16,0.515038074910054));
#28315=DIRECTION('center_axis',(0.,0.,-1.));
#28316=DIRECTION('ref_axis',(-1.,0.,0.));
#28317=DIRECTION('',(-0.707106781186548,8.65956056235493E-17,0.707106781186548));
#28318=DIRECTION('center_axis',(0.,0.,1.));
#28319=DIRECTION('ref_axis',(-1.,0.,0.));
#28320=DIRECTION('center_axis',(0.,0.,1.));
#28321=DIRECTION('ref_axis',(-1.,0.,0.));
#28322=DIRECTION('center_axis',(0.,0.,1.));
#28323=DIRECTION('ref_axis',(1.,0.,0.));
#28324=DIRECTION('center_axis',(0.,0.,1.));
#28325=DIRECTION('ref_axis',(1.,0.,0.));
#28326=DIRECTION('',(0.,0.,-1.));
#28327=DIRECTION('center_axis',(0.,0.,1.));
#28328=DIRECTION('ref_axis',(1.,0.,0.));
#28329=DIRECTION('center_axis',(0.,0.,1.));
#28330=DIRECTION('ref_axis',(1.,0.,0.));
#28331=DIRECTION('',(0.707106781186544,8.65956056235489E-17,-0.707106781186551));
#28332=DIRECTION('center_axis',(0.,0.,-1.));
#28333=DIRECTION('ref_axis',(-1.,0.,0.));
#28334=DIRECTION('center_axis',(0.,0.,1.));
#28335=DIRECTION('ref_axis',(1.,0.,0.));
#28336=DIRECTION('center_axis',(0.,0.,1.));
#28337=DIRECTION('ref_axis',(1.,0.,0.));
#28338=DIRECTION('',(0.,0.,-1.));
#28339=DIRECTION('center_axis',(0.,0.,1.));
#28340=DIRECTION('ref_axis',(1.,0.,0.));
#28341=DIRECTION('center_axis',(0.,0.,-1.));
#28342=DIRECTION('ref_axis',(-1.,0.,0.));
#43215=CARTESIAN_POINT('',(0.,0.,0.));
#43216=CARTESIAN_POINT('Ctrl Pts',(0.156070932745934,-0.596521174907684,
5.4));
#43217=CARTESIAN_POINT('Ctrl Pts',(0.156070932745934,-0.596521174907684,
5.37));
#43218=CARTESIAN_POINT('Ctrl Pts',(0.166950926184654,-0.573635852336884,
5.4));
#43219=CARTESIAN_POINT('Ctrl Pts',(0.166950926184654,-0.573635852336884,
5.37));
#43220=CARTESIAN_POINT('Ctrl Pts',(0.166950926184654,-0.528990542888641,
5.4));
#43221=CARTESIAN_POINT('Ctrl Pts',(0.166950926184654,-0.528990542888641,
5.37));
#43222=CARTESIAN_POINT('',(0.156070932745934,-0.596521174907684,5.4));
#43223=CARTESIAN_POINT('',(0.166950926184654,-0.528990542888641,5.4));
#43224=CARTESIAN_POINT('Ctrl Pts',(0.156070932745934,-0.596521174907684,
5.4));
#43225=CARTESIAN_POINT('Ctrl Pts',(0.166950926184654,-0.573635852336884,
5.4));
#43226=CARTESIAN_POINT('Ctrl Pts',(0.166950926184654,-0.528990542888641,
5.4));
#43227=CARTESIAN_POINT('',(0.156070932745934,-0.596521174907684,5.37));
#43228=CARTESIAN_POINT('',(0.156070932745934,-0.596521174907684,5.4));
#43229=CARTESIAN_POINT('',(0.166950926184654,-0.528990542888641,5.37));
#43230=CARTESIAN_POINT('Ctrl Pts',(0.156070932745934,-0.596521174907684,
5.37));
#43231=CARTESIAN_POINT('Ctrl Pts',(0.166950926184654,-0.573635852336884,
5.37));
#43232=CARTESIAN_POINT('Ctrl Pts',(0.166950926184654,-0.528990542888641,
5.37));
#43233=CARTESIAN_POINT('',(0.166950926184654,-0.528990542888641,5.4));
#43234=CARTESIAN_POINT('Ctrl Pts',(0.111425623297691,-0.643229997158051,
5.4));
#43235=CARTESIAN_POINT('Ctrl Pts',(0.111425623297691,-0.643229997158051,
5.37));
#43236=CARTESIAN_POINT('Ctrl Pts',(0.141814455389977,-0.626159703731537,
5.4));
#43237=CARTESIAN_POINT('Ctrl Pts',(0.141814455389977,-0.626159703731537,
5.37));
#43238=CARTESIAN_POINT('Ctrl Pts',(0.156070932745934,-0.596521174907684,
5.4));
#43239=CARTESIAN_POINT('Ctrl Pts',(0.156070932745934,-0.596521174907684,
5.37));
#43240=CARTESIAN_POINT('',(0.111425623297691,-0.643229997158051,5.4));
#43241=CARTESIAN_POINT('Ctrl Pts',(0.111425623297691,-0.643229997158051,
5.4));
#43242=CARTESIAN_POINT('Ctrl Pts',(0.141814455389977,-0.626159703731537,
5.4));
#43243=CARTESIAN_POINT('Ctrl Pts',(0.156070932745934,-0.596521174907684,
5.4));
#43244=CARTESIAN_POINT('',(0.111425623297691,-0.643229997158051,5.37));
#43245=CARTESIAN_POINT('',(0.111425623297691,-0.643229997158051,5.4));
#43246=CARTESIAN_POINT('Ctrl Pts',(0.111425623297691,-0.643229997158051,
5.37));
#43247=CARTESIAN_POINT('Ctrl Pts',(0.141814455389977,-0.626159703731537,
5.37));
#43248=CARTESIAN_POINT('Ctrl Pts',(0.156070932745934,-0.596521174907684,
5.37));
#43249=CARTESIAN_POINT('Ctrl Pts',(0.0420191138982773,-0.660300171375275,
5.4));
#43250=CARTESIAN_POINT('Ctrl Pts',(0.0420191138982773,-0.660300171375275,
5.37));
#43251=CARTESIAN_POINT('Ctrl Pts',(0.0810367912054062,-0.660300171375275,
5.4));
#43252=CARTESIAN_POINT('Ctrl Pts',(0.0810367912054062,-0.660300171375275,
5.37));
#43253=CARTESIAN_POINT('Ctrl Pts',(0.111425623297691,-0.643229997158051,
5.4));
#43254=CARTESIAN_POINT('Ctrl Pts',(0.111425623297691,-0.643229997158051,
5.37));
#43255=CARTESIAN_POINT('',(0.0420191138982773,-0.660300171375275,5.4));
#43256=CARTESIAN_POINT('Ctrl Pts',(0.0420191138982773,-0.660300171375275,
5.4));
#43257=CARTESIAN_POINT('Ctrl Pts',(0.0810367912054062,-0.660300171375275,
5.4));
#43258=CARTESIAN_POINT('Ctrl Pts',(0.111425623297691,-0.643229997158051,
5.4));
#43259=CARTESIAN_POINT('',(0.0420191138982773,-0.660300171375275,5.37));
#43260=CARTESIAN_POINT('',(0.0420191138982773,-0.660300171375275,5.4));
#43261=CARTESIAN_POINT('Ctrl Pts',(0.0420191138982773,-0.660300171375275,
5.37));
#43262=CARTESIAN_POINT('Ctrl Pts',(0.0810367912054062,-0.660300171375275,
5.37));
#43263=CARTESIAN_POINT('Ctrl Pts',(0.111425623297691,-0.643229997158051,
5.37));
#43264=CARTESIAN_POINT('Ctrl Pts',(-0.0178206115961075,-0.642292058467865,
5.4));
#43265=CARTESIAN_POINT('Ctrl Pts',(-0.0178206115961075,-0.642292058467865,
5.37));
#43266=CARTESIAN_POINT('Ctrl Pts',(0.00262616574764252,-0.660300171375275,
5.4));
#43267=CARTESIAN_POINT('Ctrl Pts',(0.00262616574764252,-0.660300171375275,
5.37));
#43268=CARTESIAN_POINT('Ctrl Pts',(0.0420191138982773,-0.660300171375275,
5.4));
#43269=CARTESIAN_POINT('Ctrl Pts',(0.0420191138982773,-0.660300171375275,
5.37));
#43270=CARTESIAN_POINT('',(-0.0178206115961075,-0.642292058467865,5.4));
#43271=CARTESIAN_POINT('Ctrl Pts',(-0.0178206115961075,-0.642292058467865,
5.4));
#43272=CARTESIAN_POINT('Ctrl Pts',(0.00262616574764252,-0.660300171375275,
5.4));
#43273=CARTESIAN_POINT('Ctrl Pts',(0.0420191138982773,-0.660300171375275,
5.4));
#43274=CARTESIAN_POINT('',(-0.0178206115961075,-0.642292058467865,5.37));
#43275=CARTESIAN_POINT('',(-0.0178206115961075,-0.642292058467865,5.4));
#43276=CARTESIAN_POINT('Ctrl Pts',(-0.0178206115961075,-0.642292058467865,
5.37));
#43277=CARTESIAN_POINT('Ctrl Pts',(0.00262616574764252,-0.660300171375275,
5.37));
#43278=CARTESIAN_POINT('Ctrl Pts',(0.0420191138982773,-0.660300171375275,
5.37));
#43279=CARTESIAN_POINT('Ctrl Pts',(-0.0382673889398575,-0.597271597385406,
5.4));
#43280=CARTESIAN_POINT('Ctrl Pts',(-0.0382673889398575,-0.597271597385406,
5.37));
#43281=CARTESIAN_POINT('Ctrl Pts',(-0.0382673889398575,-0.624283826351166,
5.4));
#43282=CARTESIAN_POINT('Ctrl Pts',(-0.0382673889398575,-0.624283826351166,
5.37));
#43283=CARTESIAN_POINT('Ctrl Pts',(-0.0178206115961075,-0.642292058467865,
5.4));
#43284=CARTESIAN_POINT('Ctrl Pts',(-0.0178206115961075,-0.642292058467865,
5.37));
#43285=CARTESIAN_POINT('',(-0.0382673889398575,-0.597271597385406,5.4));
#43286=CARTESIAN_POINT('Ctrl Pts',(-0.0382673889398575,-0.597271597385406,
5.4));
#43287=CARTESIAN_POINT('Ctrl Pts',(-0.0382673889398575,-0.624283826351166,
5.4));
#43288=CARTESIAN_POINT('Ctrl Pts',(-0.0178206115961075,-0.642292058467865,
5.4));
#43289=CARTESIAN_POINT('',(-0.0382673889398575,-0.597271597385406,5.37));
#43290=CARTESIAN_POINT('',(-0.0382673889398575,-0.597271597385406,5.4));
#43291=CARTESIAN_POINT('Ctrl Pts',(-0.0382673889398575,-0.597271597385406,
5.37));
#43292=CARTESIAN_POINT('Ctrl Pts',(-0.0382673889398575,-0.624283826351166,
5.37));
#43293=CARTESIAN_POINT('Ctrl Pts',(-0.0178206115961075,-0.642292058467865,
5.37));
#43294=CARTESIAN_POINT('Ctrl Pts',(-0.0288882404565811,-0.565194523334503,
5.4));
#43295=CARTESIAN_POINT('Ctrl Pts',(-0.0288882404565811,-0.565194523334503,
5.37));
#43296=CARTESIAN_POINT('Ctrl Pts',(-0.0382673889398575,-0.579638516902924,
5.4));
#43297=CARTESIAN_POINT('Ctrl Pts',(-0.0382673889398575,-0.579638516902924,
5.37));
#43298=CARTESIAN_POINT('Ctrl Pts',(-0.0382673889398575,-0.597271597385406,
5.4));
#43299=CARTESIAN_POINT('Ctrl Pts',(-0.0382673889398575,-0.597271597385406,
5.37));
#43300=CARTESIAN_POINT('',(-0.0288882404565811,-0.565194523334503,5.4));
#43301=CARTESIAN_POINT('Ctrl Pts',(-0.0288882404565811,-0.565194523334503,
5.4));
#43302=CARTESIAN_POINT('Ctrl Pts',(-0.0382673889398575,-0.579638516902924,
5.4));
#43303=CARTESIAN_POINT('Ctrl Pts',(-0.0382673889398575,-0.597271597385406,
5.4));
#43304=CARTESIAN_POINT('',(-0.0288882404565811,-0.565194523334503,5.37));
#43305=CARTESIAN_POINT('',(-0.0288882404565811,-0.565194523334503,5.4));
#43306=CARTESIAN_POINT('Ctrl Pts',(-0.0288882404565811,-0.565194523334503,
5.37));
#43307=CARTESIAN_POINT('Ctrl Pts',(-0.0382673889398575,-0.579638516902924,
5.37));
#43308=CARTESIAN_POINT('Ctrl Pts',(-0.0382673889398575,-0.597271597385406,
5.37));
#43309=CARTESIAN_POINT('Ctrl Pts',(-0.00225116312503815,-0.543247020244598,
5.4));
#43310=CARTESIAN_POINT('Ctrl Pts',(-0.00225116312503815,-0.543247020244598,
5.37));
#43311=CARTESIAN_POINT('Ctrl Pts',(-0.0195088535547256,-0.550750410556793,
5.4));
#43312=CARTESIAN_POINT('Ctrl Pts',(-0.0195088535547256,-0.550750410556793,
5.37));
#43313=CARTESIAN_POINT('Ctrl Pts',(-0.0288882404565811,-0.565194523334503,
5.4));
#43314=CARTESIAN_POINT('Ctrl Pts',(-0.0288882404565811,-0.565194523334503,
5.37));
#43315=CARTESIAN_POINT('',(-0.00225116312503815,-0.543247020244598,5.4));
#43316=CARTESIAN_POINT('Ctrl Pts',(-0.00225116312503815,-0.543247020244598,
5.4));
#43317=CARTESIAN_POINT('Ctrl Pts',(-0.0195088535547256,-0.550750410556793,
5.4));
#43318=CARTESIAN_POINT('Ctrl Pts',(-0.0288882404565811,-0.565194523334503,
5.4));
#43319=CARTESIAN_POINT('',(-0.00225116312503815,-0.543247020244598,5.37));
#43320=CARTESIAN_POINT('',(-0.00225116312503815,-0.543247020244598,5.4));
#43321=CARTESIAN_POINT('Ctrl Pts',(-0.00225116312503815,-0.543247020244598,
5.37));
#43322=CARTESIAN_POINT('Ctrl Pts',(-0.0195088535547256,-0.550750410556793,
5.37));
#43323=CARTESIAN_POINT('Ctrl Pts',(-0.0288882404565811,-0.565194523334503,
5.37));
#43324=CARTESIAN_POINT('Ctrl Pts',(0.0566506236791611,-0.529740846157074,
5.4));
#43325=CARTESIAN_POINT('Ctrl Pts',(0.0566506236791611,-0.529740846157074,
5.37));
#43326=CARTESIAN_POINT('Ctrl Pts',(0.0150067657232285,-0.535743629932404,
5.4));
#43327=CARTESIAN_POINT('Ctrl Pts',(0.0150067657232285,-0.535743629932404,
5.37));
#43328=CARTESIAN_POINT('Ctrl Pts',(-0.00225116312503815,-0.543247020244598,
5.4));
#43329=CARTESIAN_POINT('Ctrl Pts',(-0.00225116312503815,-0.543247020244598,
5.37));
#43330=CARTESIAN_POINT('',(0.0566506236791611,-0.529740846157074,5.4));
#43331=CARTESIAN_POINT('Ctrl Pts',(0.0566506236791611,-0.529740846157074,
5.4));
#43332=CARTESIAN_POINT('Ctrl Pts',(0.0150067657232285,-0.535743629932404,
5.4));
#43333=CARTESIAN_POINT('Ctrl Pts',(-0.00225116312503815,-0.543247020244598,
5.4));
#43334=CARTESIAN_POINT('',(0.0566506236791611,-0.529740846157074,5.37));
#43335=CARTESIAN_POINT('',(0.0566506236791611,-0.529740846157074,5.4));
#43336=CARTESIAN_POINT('Ctrl Pts',(0.0566506236791611,-0.529740846157074,
5.37));
#43337=CARTESIAN_POINT('Ctrl Pts',(0.0150067657232285,-0.535743629932404,
5.37));
#43338=CARTESIAN_POINT('Ctrl Pts',(-0.00225116312503815,-0.543247020244598,
5.37));
#43339=CARTESIAN_POINT('Ctrl Pts',(0.166950926184654,-0.50422922372818,
5.4));
#43340=CARTESIAN_POINT('Ctrl Pts',(0.166950926184654,-0.50422922372818,
5.37));
#43341=CARTESIAN_POINT('Ctrl Pts',(0.130184158682823,-0.519236123561859,
5.4));
#43342=CARTESIAN_POINT('Ctrl Pts',(0.130184158682823,-0.519236123561859,
5.37));
#43343=CARTESIAN_POINT('Ctrl Pts',(0.0566506236791611,-0.529740846157074,
5.4));
#43344=CARTESIAN_POINT('Ctrl Pts',(0.0566506236791611,-0.529740846157074,
5.37));
#43345=CARTESIAN_POINT('',(0.166950926184654,-0.50422922372818,5.4));
#43346=CARTESIAN_POINT('Ctrl Pts',(0.166950926184654,-0.50422922372818,
5.4));
#43347=CARTESIAN_POINT('Ctrl Pts',(0.130184158682823,-0.519236123561859,
5.4));
#43348=CARTESIAN_POINT('Ctrl Pts',(0.0566506236791611,-0.529740846157074,
5.4));
#43349=CARTESIAN_POINT('',(0.166950926184654,-0.50422922372818,5.37));
#43350=CARTESIAN_POINT('',(0.166950926184654,-0.50422922372818,5.4));
#43351=CARTESIAN_POINT('Ctrl Pts',(0.166950926184654,-0.50422922372818,
5.37));
#43352=CARTESIAN_POINT('Ctrl Pts',(0.130184158682823,-0.519236123561859,
5.37));
#43353=CARTESIAN_POINT('Ctrl Pts',(0.0566506236791611,-0.529740846157074,
5.37));
#43354=CARTESIAN_POINT('Origin',(0.166950926184654,-0.528990542888641,5.4));
#43355=CARTESIAN_POINT('',(0.166950926184654,-0.264495271444321,5.4));
#43356=CARTESIAN_POINT('',(0.166950926184654,-0.528990542888641,5.37));
#43357=CARTESIAN_POINT('Ctrl Pts',(0.239546284079552,-0.656360900402069,
5.4));
#43358=CARTESIAN_POINT('Ctrl Pts',(0.239546284079552,-0.656360900402069,
5.37));
#43359=CARTESIAN_POINT('Ctrl Pts',(0.243860706686974,-0.681309735774994,
5.4));
#43360=CARTESIAN_POINT('Ctrl Pts',(0.243860706686974,-0.681309735774994,
5.37));
#43361=CARTESIAN_POINT('Ctrl Pts',(0.256616577506065,-0.704195177555084,
5.4));
#43362=CARTESIAN_POINT('Ctrl Pts',(0.256616577506065,-0.704195177555084,
5.37));
#43363=CARTESIAN_POINT('',(0.239546284079552,-0.656360900402069,5.4));
#43364=CARTESIAN_POINT('',(0.256616577506065,-0.704195177555084,5.4));
#43365=CARTESIAN_POINT('Ctrl Pts',(0.239546284079552,-0.656360900402069,
5.4));
#43366=CARTESIAN_POINT('Ctrl Pts',(0.243860706686974,-0.681309735774994,
5.4));
#43367=CARTESIAN_POINT('Ctrl Pts',(0.256616577506065,-0.704195177555084,
5.4));
#43368=CARTESIAN_POINT('',(0.239546284079552,-0.656360900402069,5.37));
#43369=CARTESIAN_POINT('',(0.239546284079552,-0.656360900402069,5.4));
#43370=CARTESIAN_POINT('',(0.256616577506065,-0.704195177555084,5.37));
#43371=CARTESIAN_POINT('Ctrl Pts',(0.239546284079552,-0.656360900402069,
5.37));
#43372=CARTESIAN_POINT('Ctrl Pts',(0.243860706686974,-0.681309735774994,
5.37));
#43373=CARTESIAN_POINT('Ctrl Pts',(0.256616577506065,-0.704195177555084,
5.37));
#43374=CARTESIAN_POINT('',(0.256616577506065,-0.704195177555084,5.4));
#43375=CARTESIAN_POINT('Ctrl Pts',(0.23523186147213,-0.537244236469269,
5.4));
#43376=CARTESIAN_POINT('Ctrl Pts',(0.23523186147213,-0.537244236469269,
5.37));
#43377=CARTESIAN_POINT('Ctrl Pts',(0.23523186147213,-0.631412065029144,
5.4));
#43378=CARTESIAN_POINT('Ctrl Pts',(0.23523186147213,-0.631412065029144,
5.37));
#43379=CARTESIAN_POINT('Ctrl Pts',(0.239546284079552,-0.656360900402069,
5.4));
#43380=CARTESIAN_POINT('Ctrl Pts',(0.239546284079552,-0.656360900402069,
5.37));
#43381=CARTESIAN_POINT('',(0.23523186147213,-0.537244236469269,5.4));
#43382=CARTESIAN_POINT('Ctrl Pts',(0.23523186147213,-0.537244236469269,
5.4));
#43383=CARTESIAN_POINT('Ctrl Pts',(0.23523186147213,-0.631412065029144,
5.4));
#43384=CARTESIAN_POINT('Ctrl Pts',(0.239546284079552,-0.656360900402069,
5.4));
#43385=CARTESIAN_POINT('',(0.23523186147213,-0.537244236469269,5.37));
#43386=CARTESIAN_POINT('',(0.23523186147213,-0.537244236469269,5.4));
#43387=CARTESIAN_POINT('Ctrl Pts',(0.23523186147213,-0.537244236469269,
5.37));
#43388=CARTESIAN_POINT('Ctrl Pts',(0.23523186147213,-0.631412065029144,
5.37));
#43389=CARTESIAN_POINT('Ctrl Pts',(0.239546284079552,-0.656360900402069,
5.37));
#43390=CARTESIAN_POINT('Origin',(0.23523186147213,-0.447203314304352,5.4));
#43391=CARTESIAN_POINT('',(0.23523186147213,-0.447203314304352,5.4));
#43392=CARTESIAN_POINT('',(0.23523186147213,-0.223601657152176,5.4));
#43393=CARTESIAN_POINT('',(0.23523186147213,-0.447203314304352,5.37));
#43394=CARTESIAN_POINT('',(0.23523186147213,-0.447203314304352,5.4));
#43395=CARTESIAN_POINT('',(0.23523186147213,-0.447203314304352,5.37));
#43396=CARTESIAN_POINT('Ctrl Pts',(0.231855377554893,-0.384925043582916,
5.4));
#43397=CARTESIAN_POINT('Ctrl Pts',(0.231855377554893,-0.384925043582916,
5.37));
#43398=CARTESIAN_POINT('Ctrl Pts',(0.23523186147213,-0.402182853221893,
5.4));
#43399=CARTESIAN_POINT('Ctrl Pts',(0.23523186147213,-0.402182853221893,
5.37));
#43400=CARTESIAN_POINT('Ctrl Pts',(0.23523186147213,-0.447203314304352,
5.4));
#43401=CARTESIAN_POINT('Ctrl Pts',(0.23523186147213,-0.447203314304352,
5.37));
#43402=CARTESIAN_POINT('',(0.231855377554893,-0.384925043582916,5.4));
#43403=CARTESIAN_POINT('Ctrl Pts',(0.231855377554893,-0.384925043582916,
5.4));
#43404=CARTESIAN_POINT('Ctrl Pts',(0.23523186147213,-0.402182853221893,
5.4));
#43405=CARTESIAN_POINT('Ctrl Pts',(0.23523186147213,-0.447203314304352,
5.4));
#43406=CARTESIAN_POINT('',(0.231855377554893,-0.384925043582916,5.37));
#43407=CARTESIAN_POINT('',(0.231855377554893,-0.384925043582916,5.4));
#43408=CARTESIAN_POINT('Ctrl Pts',(0.231855377554893,-0.384925043582916,
5.37));
#43409=CARTESIAN_POINT('Ctrl Pts',(0.23523186147213,-0.402182853221893,
5.37));
#43410=CARTESIAN_POINT('Ctrl Pts',(0.23523186147213,-0.447203314304352,
5.37));
#43411=CARTESIAN_POINT('Ctrl Pts',(0.210845932364464,-0.338966643810272,
5.4));
#43412=CARTESIAN_POINT('Ctrl Pts',(0.210845932364464,-0.338966643810272,
5.37));
#43413=CARTESIAN_POINT('Ctrl Pts',(0.225852712988853,-0.357162392139435,
5.4));
#43414=CARTESIAN_POINT('Ctrl Pts',(0.225852712988853,-0.357162392139435,
5.37));
#43415=CARTESIAN_POINT('Ctrl Pts',(0.231855377554893,-0.384925043582916,
5.4));
#43416=CARTESIAN_POINT('Ctrl Pts',(0.231855377554893,-0.384925043582916,
5.37));
#43417=CARTESIAN_POINT('',(0.210845932364464,-0.338966643810272,5.4));
#43418=CARTESIAN_POINT('Ctrl Pts',(0.210845932364464,-0.338966643810272,
5.4));
#43419=CARTESIAN_POINT('Ctrl Pts',(0.225852712988853,-0.357162392139435,
5.4));
#43420=CARTESIAN_POINT('Ctrl Pts',(0.231855377554893,-0.384925043582916,
5.4));
#43421=CARTESIAN_POINT('',(0.210845932364464,-0.338966643810272,5.37));
#43422=CARTESIAN_POINT('',(0.210845932364464,-0.338966643810272,5.4));
#43423=CARTESIAN_POINT('Ctrl Pts',(0.210845932364464,-0.338966643810272,
5.37));
#43424=CARTESIAN_POINT('Ctrl Pts',(0.225852712988853,-0.357162392139435,
5.37));
#43425=CARTESIAN_POINT('Ctrl Pts',(0.231855377554893,-0.384925043582916,
5.37));
#43426=CARTESIAN_POINT('Ctrl Pts',(0.163949474692345,-0.30876544713974,
5.4));
#43427=CARTESIAN_POINT('Ctrl Pts',(0.163949474692345,-0.30876544713974,
5.37));
#43428=CARTESIAN_POINT('Ctrl Pts',(0.195838913321495,-0.32077089548111,
5.4));
#43429=CARTESIAN_POINT('Ctrl Pts',(0.195838913321495,-0.32077089548111,
5.37));
#43430=CARTESIAN_POINT('Ctrl Pts',(0.210845932364464,-0.338966643810272,
5.4));
#43431=CARTESIAN_POINT('Ctrl Pts',(0.210845932364464,-0.338966643810272,
5.37));
#43432=CARTESIAN_POINT('',(0.163949474692345,-0.30876544713974,5.4));
#43433=CARTESIAN_POINT('Ctrl Pts',(0.163949474692345,-0.30876544713974,
5.4));
#43434=CARTESIAN_POINT('Ctrl Pts',(0.195838913321495,-0.32077089548111,
5.4));
#43435=CARTESIAN_POINT('Ctrl Pts',(0.210845932364464,-0.338966643810272,
5.4));
#43436=CARTESIAN_POINT('',(0.163949474692345,-0.30876544713974,5.37));
#43437=CARTESIAN_POINT('',(0.163949474692345,-0.30876544713974,5.4));
#43438=CARTESIAN_POINT('Ctrl Pts',(0.163949474692345,-0.30876544713974,
5.37));
#43439=CARTESIAN_POINT('Ctrl Pts',(0.195838913321495,-0.32077089548111,
5.37));
#43440=CARTESIAN_POINT('Ctrl Pts',(0.210845932364464,-0.338966643810272,
5.37));
#43441=CARTESIAN_POINT('Ctrl Pts',(0.0810367912054062,-0.296759939193726,
5.4));
#43442=CARTESIAN_POINT('Ctrl Pts',(0.0810367912054062,-0.296759939193726,
5.37));
#43443=CARTESIAN_POINT('Ctrl Pts',(0.132060036063194,-0.296759939193726,
5.4));
#43444=CARTESIAN_POINT('Ctrl Pts',(0.132060036063194,-0.296759939193726,
5.37));
#43445=CARTESIAN_POINT('Ctrl Pts',(0.163949474692345,-0.30876544713974,
5.4));
#43446=CARTESIAN_POINT('Ctrl Pts',(0.163949474692345,-0.30876544713974,
5.37));
#43447=CARTESIAN_POINT('',(0.0810367912054062,-0.296759939193726,5.4));
#43448=CARTESIAN_POINT('Ctrl Pts',(0.0810367912054062,-0.296759939193726,
5.4));
#43449=CARTESIAN_POINT('Ctrl Pts',(0.132060036063194,-0.296759939193726,
5.4));
#43450=CARTESIAN_POINT('Ctrl Pts',(0.163949474692345,-0.30876544713974,
5.4));
#43451=CARTESIAN_POINT('',(0.0810367912054062,-0.296759939193726,5.37));
#43452=CARTESIAN_POINT('',(0.0810367912054062,-0.296759939193726,5.4));
#43453=CARTESIAN_POINT('Ctrl Pts',(0.0810367912054062,-0.296759939193726,
5.37));
#43454=CARTESIAN_POINT('Ctrl Pts',(0.132060036063194,-0.296759939193726,
5.37));
#43455=CARTESIAN_POINT('Ctrl Pts',(0.163949474692345,-0.30876544713974,
5.37));
#43456=CARTESIAN_POINT('Ctrl Pts',(-0.00937940180301666,-0.310828840732574,
5.4));
#43457=CARTESIAN_POINT('Ctrl Pts',(-0.00937940180301666,-0.310828840732574,
5.37));
#43458=CARTESIAN_POINT('Ctrl Pts',(0.0296385139226913,-0.296759939193726,
5.4));
#43459=CARTESIAN_POINT('Ctrl Pts',(0.0296385139226913,-0.296759939193726,
5.37));
#43460=CARTESIAN_POINT('Ctrl Pts',(0.0810367912054062,-0.296759939193726,
5.4));
#43461=CARTESIAN_POINT('Ctrl Pts',(0.0810367912054062,-0.296759939193726,
5.37));
#43462=CARTESIAN_POINT('',(-0.00937940180301666,-0.310828840732574,5.4));
#43463=CARTESIAN_POINT('Ctrl Pts',(-0.00937940180301666,-0.310828840732574,
5.4));
#43464=CARTESIAN_POINT('Ctrl Pts',(0.0296385139226913,-0.296759939193726,
5.4));
#43465=CARTESIAN_POINT('Ctrl Pts',(0.0810367912054062,-0.296759939193726,
5.4));
#43466=CARTESIAN_POINT('',(-0.00937940180301666,-0.310828840732574,5.37));
#43467=CARTESIAN_POINT('',(-0.00937940180301666,-0.310828840732574,5.4));
#43468=CARTESIAN_POINT('Ctrl Pts',(-0.00937940180301666,-0.310828840732574,
5.37));
#43469=CARTESIAN_POINT('Ctrl Pts',(0.0296385139226913,-0.296759939193726,
5.37));
#43470=CARTESIAN_POINT('Ctrl Pts',(0.0810367912054062,-0.296759939193726,
5.37));
#43471=CARTESIAN_POINT('Ctrl Pts',(-0.0690312534570694,-0.350972092151642,
5.4));
#43472=CARTESIAN_POINT('Ctrl Pts',(-0.0690312534570694,-0.350972092151642,
5.37));
#43473=CARTESIAN_POINT('Ctrl Pts',(-0.0483970791101456,-0.324897742271423,
5.4));
#43474=CARTESIAN_POINT('Ctrl Pts',(-0.0483970791101456,-0.324897742271423,
5.37));
#43475=CARTESIAN_POINT('Ctrl Pts',(-0.00937940180301666,-0.310828840732574,
5.4));
#43476=CARTESIAN_POINT('Ctrl Pts',(-0.00937940180301666,-0.310828840732574,
5.37));
#43477=CARTESIAN_POINT('',(-0.0690312534570694,-0.350972092151642,5.4));
#43478=CARTESIAN_POINT('Ctrl Pts',(-0.0690312534570694,-0.350972092151642,
5.4));
#43479=CARTESIAN_POINT('Ctrl Pts',(-0.0483970791101456,-0.324897742271423,
5.4));
#43480=CARTESIAN_POINT('Ctrl Pts',(-0.00937940180301666,-0.310828840732574,
5.4));
#43481=CARTESIAN_POINT('',(-0.0690312534570694,-0.350972092151642,5.37));
#43482=CARTESIAN_POINT('',(-0.0690312534570694,-0.350972092151642,5.4));
#43483=CARTESIAN_POINT('Ctrl Pts',(-0.0690312534570694,-0.350972092151642,
5.37));
#43484=CARTESIAN_POINT('Ctrl Pts',(-0.0483970791101456,-0.324897742271423,
5.37));
#43485=CARTESIAN_POINT('Ctrl Pts',(-0.00937940180301666,-0.310828840732574,
5.37));
#43486=CARTESIAN_POINT('Ctrl Pts',(-0.0986697822809219,-0.419440722465515,
5.4));
#43487=CARTESIAN_POINT('Ctrl Pts',(-0.0986697822809219,-0.419440722465515,
5.37));
#43488=CARTESIAN_POINT('Ctrl Pts',(-0.0896656662225723,-0.37704644203186,
5.4));
#43489=CARTESIAN_POINT('Ctrl Pts',(-0.0896656662225723,-0.37704644203186,
5.37));
#43490=CARTESIAN_POINT('Ctrl Pts',(-0.0690312534570694,-0.350972092151642,
5.4));
#43491=CARTESIAN_POINT('Ctrl Pts',(-0.0690312534570694,-0.350972092151642,
5.37));
#43492=CARTESIAN_POINT('',(-0.0986697822809219,-0.419440722465515,5.4));
#43493=CARTESIAN_POINT('Ctrl Pts',(-0.0986697822809219,-0.419440722465515,
5.4));
#43494=CARTESIAN_POINT('Ctrl Pts',(-0.0896656662225723,-0.37704644203186,
5.4));
#43495=CARTESIAN_POINT('Ctrl Pts',(-0.0690312534570694,-0.350972092151642,
5.4));
#43496=CARTESIAN_POINT('',(-0.0986697822809219,-0.419440722465515,5.37));
#43497=CARTESIAN_POINT('',(-0.0986697822809219,-0.419440722465515,5.4));
#43498=CARTESIAN_POINT('Ctrl Pts',(-0.0986697822809219,-0.419440722465515,
5.37));
#43499=CARTESIAN_POINT('Ctrl Pts',(-0.0896656662225723,-0.37704644203186,
5.37));
#43500=CARTESIAN_POINT('Ctrl Pts',(-0.0690312534570694,-0.350972092151642,
5.37));
#43501=CARTESIAN_POINT('Origin',(-0.0326397567987442,-0.42844477891922,
5.4));
#43502=CARTESIAN_POINT('',(-0.0326397567987442,-0.42844477891922,5.4));
#43503=CARTESIAN_POINT('',(-0.0452965477902544,-0.426718860145479,5.4));
#43504=CARTESIAN_POINT('',(-0.0326397567987442,-0.42844477891922,5.37));
#43505=CARTESIAN_POINT('',(-0.0326397567987442,-0.42844477891922,5.4));
#43506=CARTESIAN_POINT('',(-0.0326397567987442,-0.42844477891922,5.37));
#43507=CARTESIAN_POINT('Ctrl Pts',(0.000937923789024353,-0.369355475902557,
5.4));
#43508=CARTESIAN_POINT('Ctrl Pts',(0.000937923789024353,-0.369355475902557,
5.37));
#43509=CARTESIAN_POINT('Ctrl Pts',(-0.0217600017786026,-0.386050498485565,
5.4));
#43510=CARTESIAN_POINT('Ctrl Pts',(-0.0217600017786026,-0.386050498485565,
5.37));
#43511=CARTESIAN_POINT('Ctrl Pts',(-0.0326397567987442,-0.42844477891922,
5.4));
#43512=CARTESIAN_POINT('Ctrl Pts',(-0.0326397567987442,-0.42844477891922,
5.37));
#43513=CARTESIAN_POINT('',(0.000937923789024353,-0.369355475902557,5.4));
#43514=CARTESIAN_POINT('Ctrl Pts',(0.000937923789024353,-0.369355475902557,
5.4));
#43515=CARTESIAN_POINT('Ctrl Pts',(-0.0217600017786026,-0.386050498485565,
5.4));
#43516=CARTESIAN_POINT('Ctrl Pts',(-0.0326397567987442,-0.42844477891922,
5.4));
#43517=CARTESIAN_POINT('',(0.000937923789024353,-0.369355475902557,5.37));
#43518=CARTESIAN_POINT('',(0.000937923789024353,-0.369355475902557,5.4));
#43519=CARTESIAN_POINT('Ctrl Pts',(0.000937923789024353,-0.369355475902557,
5.37));
#43520=CARTESIAN_POINT('Ctrl Pts',(-0.0217600017786026,-0.386050498485565,
5.37));
#43521=CARTESIAN_POINT('Ctrl Pts',(-0.0326397567987442,-0.42844477891922,
5.37));
#43522=CARTESIAN_POINT('Ctrl Pts',(0.071282371878624,-0.35266033411026,
5.4));
#43523=CARTESIAN_POINT('Ctrl Pts',(0.071282371878624,-0.35266033411026,
5.37));
#43524=CARTESIAN_POINT('Ctrl Pts',(0.0236358493566513,-0.35266033411026,
5.4));
#43525=CARTESIAN_POINT('Ctrl Pts',(0.0236358493566513,-0.35266033411026,
5.37));
#43526=CARTESIAN_POINT('Ctrl Pts',(0.000937923789024353,-0.369355475902557,
5.4));
#43527=CARTESIAN_POINT('Ctrl Pts',(0.000937923789024353,-0.369355475902557,
5.37));
#43528=CARTESIAN_POINT('',(0.071282371878624,-0.35266033411026,5.4));
#43529=CARTESIAN_POINT('Ctrl Pts',(0.071282371878624,-0.35266033411026,
5.4));
#43530=CARTESIAN_POINT('Ctrl Pts',(0.0236358493566513,-0.35266033411026,
5.4));
#43531=CARTESIAN_POINT('Ctrl Pts',(0.000937923789024353,-0.369355475902557,
5.4));
#43532=CARTESIAN_POINT('',(0.071282371878624,-0.35266033411026,5.37));
#43533=CARTESIAN_POINT('',(0.071282371878624,-0.35266033411026,5.4));
#43534=CARTESIAN_POINT('Ctrl Pts',(0.071282371878624,-0.35266033411026,
5.37));
#43535=CARTESIAN_POINT('Ctrl Pts',(0.0236358493566513,-0.35266033411026,
5.37));
#43536=CARTESIAN_POINT('Ctrl Pts',(0.000937923789024353,-0.369355475902557,
5.37));
#43537=CARTESIAN_POINT('Ctrl Pts',(0.148192390799522,-0.37554577589035,
5.4));
#43538=CARTESIAN_POINT('Ctrl Pts',(0.148192390799522,-0.37554577589035,
5.37));
#43539=CARTESIAN_POINT('Ctrl Pts',(0.122305616736412,-0.35266033411026,
5.4));
#43540=CARTESIAN_POINT('Ctrl Pts',(0.122305616736412,-0.35266033411026,
5.37));
#43541=CARTESIAN_POINT('Ctrl Pts',(0.071282371878624,-0.35266033411026,
5.4));
#43542=CARTESIAN_POINT('Ctrl Pts',(0.071282371878624,-0.35266033411026,
5.37));
#43543=CARTESIAN_POINT('',(0.148192390799522,-0.37554577589035,5.4));
#43544=CARTESIAN_POINT('Ctrl Pts',(0.148192390799522,-0.37554577589035,
5.4));
#43545=CARTESIAN_POINT('Ctrl Pts',(0.122305616736412,-0.35266033411026,
5.4));
#43546=CARTESIAN_POINT('Ctrl Pts',(0.071282371878624,-0.35266033411026,
5.4));
#43547=CARTESIAN_POINT('',(0.148192390799522,-0.37554577589035,5.37));
#43548=CARTESIAN_POINT('',(0.148192390799522,-0.37554577589035,5.4));
#43549=CARTESIAN_POINT('Ctrl Pts',(0.148192390799522,-0.37554577589035,
5.37));
#43550=CARTESIAN_POINT('Ctrl Pts',(0.122305616736412,-0.35266033411026,
5.37));
#43551=CARTESIAN_POINT('Ctrl Pts',(0.071282371878624,-0.35266033411026,
5.37));
#43552=CARTESIAN_POINT('Ctrl Pts',(0.167325958609581,-0.433697199821472,
5.4));
#43553=CARTESIAN_POINT('Ctrl Pts',(0.167325958609581,-0.433697199821472,
5.37));
#43554=CARTESIAN_POINT('Ctrl Pts',(0.167325958609581,-0.392428433895111,
5.4));
#43555=CARTESIAN_POINT('Ctrl Pts',(0.167325958609581,-0.392428433895111,
5.37));
#43556=CARTESIAN_POINT('Ctrl Pts',(0.148192390799522,-0.37554577589035,
5.4));
#43557=CARTESIAN_POINT('Ctrl Pts',(0.148192390799522,-0.37554577589035,
5.37));
#43558=CARTESIAN_POINT('',(0.167325958609581,-0.433697199821472,5.4));
#43559=CARTESIAN_POINT('Ctrl Pts',(0.167325958609581,-0.433697199821472,
5.4));
#43560=CARTESIAN_POINT('Ctrl Pts',(0.167325958609581,-0.392428433895111,
5.4));
#43561=CARTESIAN_POINT('Ctrl Pts',(0.148192390799522,-0.37554577589035,
5.4));
#43562=CARTESIAN_POINT('',(0.167325958609581,-0.433697199821472,5.37));
#43563=CARTESIAN_POINT('',(0.167325958609581,-0.433697199821472,5.4));
#43564=CARTESIAN_POINT('Ctrl Pts',(0.167325958609581,-0.433697199821472,
5.37));
#43565=CARTESIAN_POINT('Ctrl Pts',(0.167325958609581,-0.392428433895111,
5.37));
#43566=CARTESIAN_POINT('Ctrl Pts',(0.148192390799522,-0.37554577589035,
5.37));
#43567=CARTESIAN_POINT('Ctrl Pts',(0.166950926184654,-0.45133022069931,
5.4));
#43568=CARTESIAN_POINT('Ctrl Pts',(0.166950926184654,-0.45133022069931,
5.37));
#43569=CARTESIAN_POINT('Ctrl Pts',(0.167325958609581,-0.43744889497757,
5.4));
#43570=CARTESIAN_POINT('Ctrl Pts',(0.167325958609581,-0.43744889497757,
5.37));
#43571=CARTESIAN_POINT('Ctrl Pts',(0.167325958609581,-0.433697199821472,
5.4));
#43572=CARTESIAN_POINT('Ctrl Pts',(0.167325958609581,-0.433697199821472,
5.37));
#43573=CARTESIAN_POINT('',(0.166950926184654,-0.45133022069931,5.4));
#43574=CARTESIAN_POINT('Ctrl Pts',(0.166950926184654,-0.45133022069931,
5.4));
#43575=CARTESIAN_POINT('Ctrl Pts',(0.167325958609581,-0.43744889497757,
5.4));
#43576=CARTESIAN_POINT('Ctrl Pts',(0.167325958609581,-0.433697199821472,
5.4));
#43577=CARTESIAN_POINT('',(0.166950926184654,-0.45133022069931,5.37));
#43578=CARTESIAN_POINT('',(0.166950926184654,-0.45133022069931,5.4));
#43579=CARTESIAN_POINT('Ctrl Pts',(0.166950926184654,-0.45133022069931,
5.37));
#43580=CARTESIAN_POINT('Ctrl Pts',(0.167325958609581,-0.43744889497757,
5.37));
#43581=CARTESIAN_POINT('Ctrl Pts',(0.167325958609581,-0.433697199821472,
5.37));
#43582=CARTESIAN_POINT('Ctrl Pts',(0.0465211719274521,-0.474590814113617,
5.4));
#43583=CARTESIAN_POINT('Ctrl Pts',(0.0465211719274521,-0.474590814113617,
5.37));
#43584=CARTESIAN_POINT('Ctrl Pts',(0.128308281302452,-0.464836394786835,
5.4));
#43585=CARTESIAN_POINT('Ctrl Pts',(0.128308281302452,-0.464836394786835,
5.37));
#43586=CARTESIAN_POINT('Ctrl Pts',(0.166950926184654,-0.45133022069931,
5.4));
#43587=CARTESIAN_POINT('Ctrl Pts',(0.166950926184654,-0.45133022069931,
5.37));
#43588=CARTESIAN_POINT('',(0.0465211719274521,-0.474590814113617,5.4));
#43589=CARTESIAN_POINT('Ctrl Pts',(0.0465211719274521,-0.474590814113617,
5.4));
#43590=CARTESIAN_POINT('Ctrl Pts',(0.128308281302452,-0.464836394786835,
5.4));
#43591=CARTESIAN_POINT('Ctrl Pts',(0.166950926184654,-0.45133022069931,
5.4));
#43592=CARTESIAN_POINT('',(0.0465211719274521,-0.474590814113617,5.37));
#43593=CARTESIAN_POINT('',(0.0465211719274521,-0.474590814113617,5.4));
#43594=CARTESIAN_POINT('Ctrl Pts',(0.0465211719274521,-0.474590814113617,
5.37));
#43595=CARTESIAN_POINT('Ctrl Pts',(0.128308281302452,-0.464836394786835,
5.37));
#43596=CARTESIAN_POINT('Ctrl Pts',(0.166950926184654,-0.45133022069931,
5.37));
#43597=CARTESIAN_POINT('Ctrl Pts',(-0.0135061889886856,-0.484720385074615,
5.4));
#43598=CARTESIAN_POINT('Ctrl Pts',(-0.0135061889886856,-0.484720385074615,
5.37));
#43599=CARTESIAN_POINT('Ctrl Pts',(0.0063779205083847,-0.479468023777008,
5.4));
#43600=CARTESIAN_POINT('Ctrl Pts',(0.0063779205083847,-0.479468023777008,
5.37));
#43601=CARTESIAN_POINT('Ctrl Pts',(0.0465211719274521,-0.474590814113617,
5.4));
#43602=CARTESIAN_POINT('Ctrl Pts',(0.0465211719274521,-0.474590814113617,
5.37));
#43603=CARTESIAN_POINT('',(-0.0135061889886856,-0.484720385074615,5.4));
#43604=CARTESIAN_POINT('Ctrl Pts',(-0.0135061889886856,-0.484720385074615,
5.4));
#43605=CARTESIAN_POINT('Ctrl Pts',(0.0063779205083847,-0.479468023777008,
5.4));
#43606=CARTESIAN_POINT('Ctrl Pts',(0.0465211719274521,-0.474590814113617,
5.4));
#43607=CARTESIAN_POINT('',(-0.0135061889886856,-0.484720385074615,5.37));
#43608=CARTESIAN_POINT('',(-0.0135061889886856,-0.484720385074615,5.4));
#43609=CARTESIAN_POINT('Ctrl Pts',(-0.0135061889886856,-0.484720385074615,
5.37));
#43610=CARTESIAN_POINT('Ctrl Pts',(0.0063779205083847,-0.479468023777008,
5.37));
#43611=CARTESIAN_POINT('Ctrl Pts',(0.0465211719274521,-0.474590814113617,
5.37));
#43612=CARTESIAN_POINT('Ctrl Pts',(-0.0620906502008438,-0.506855404376984,
5.4));
#43613=CARTESIAN_POINT('Ctrl Pts',(-0.0620906502008438,-0.506855404376984,
5.37));
#43614=CARTESIAN_POINT('Ctrl Pts',(-0.0405182987451553,-0.49222377538681,
5.4));
#43615=CARTESIAN_POINT('Ctrl Pts',(-0.0405182987451553,-0.49222377538681,
5.37));
#43616=CARTESIAN_POINT('Ctrl Pts',(-0.0135061889886856,-0.484720385074615,
5.4));
#43617=CARTESIAN_POINT('Ctrl Pts',(-0.0135061889886856,-0.484720385074615,
5.37));
#43618=CARTESIAN_POINT('',(-0.0620906502008438,-0.506855404376984,5.4));
#43619=CARTESIAN_POINT('Ctrl Pts',(-0.0620906502008438,-0.506855404376984,
5.4));
#43620=CARTESIAN_POINT('Ctrl Pts',(-0.0405182987451553,-0.49222377538681,
5.4));
#43621=CARTESIAN_POINT('Ctrl Pts',(-0.0135061889886856,-0.484720385074615,
5.4));
#43622=CARTESIAN_POINT('',(-0.0620906502008438,-0.506855404376984,5.37));
#43623=CARTESIAN_POINT('',(-0.0620906502008438,-0.506855404376984,5.4));
#43624=CARTESIAN_POINT('Ctrl Pts',(-0.0620906502008438,-0.506855404376984,
5.37));
#43625=CARTESIAN_POINT('Ctrl Pts',(-0.0405182987451553,-0.49222377538681,
5.37));
#43626=CARTESIAN_POINT('Ctrl Pts',(-0.0135061889886856,-0.484720385074615,
5.37));
#43627=CARTESIAN_POINT('Ctrl Pts',(-0.0969815403223038,-0.545685684680939,
5.4));
#43628=CARTESIAN_POINT('Ctrl Pts',(-0.0969815403223038,-0.545685684680939,
5.37));
#43629=CARTESIAN_POINT('Ctrl Pts',(-0.0836630016565323,-0.521487152576447,
5.4));
#43630=CARTESIAN_POINT('Ctrl Pts',(-0.0836630016565323,-0.521487152576447,
5.37));
#43631=CARTESIAN_POINT('Ctrl Pts',(-0.0620906502008438,-0.506855404376984,
5.4));
#43632=CARTESIAN_POINT('Ctrl Pts',(-0.0620906502008438,-0.506855404376984,
5.37));
#43633=CARTESIAN_POINT('',(-0.0969815403223038,-0.545685684680939,5.4));
#43634=CARTESIAN_POINT('Ctrl Pts',(-0.0969815403223038,-0.545685684680939,
5.4));
#43635=CARTESIAN_POINT('Ctrl Pts',(-0.0836630016565323,-0.521487152576447,
5.4));
#43636=CARTESIAN_POINT('Ctrl Pts',(-0.0620906502008438,-0.506855404376984,
5.4));
#43637=CARTESIAN_POINT('',(-0.0969815403223038,-0.545685684680939,5.37));
#43638=CARTESIAN_POINT('',(-0.0969815403223038,-0.545685684680939,5.4));
#43639=CARTESIAN_POINT('Ctrl Pts',(-0.0969815403223038,-0.545685684680939,
5.37));
#43640=CARTESIAN_POINT('Ctrl Pts',(-0.0836630016565323,-0.521487152576447,
5.37));
#43641=CARTESIAN_POINT('Ctrl Pts',(-0.0620906502008438,-0.506855404376984,
5.37));
#43642=CARTESIAN_POINT('Ctrl Pts',(-0.110300078988075,-0.599147474765778,
5.4));
#43643=CARTESIAN_POINT('Ctrl Pts',(-0.110300078988075,-0.599147474765778,
5.37));
#43644=CARTESIAN_POINT('Ctrl Pts',(-0.110300078988075,-0.569884097576141,
5.4));
#43645=CARTESIAN_POINT('Ctrl Pts',(-0.110300078988075,-0.569884097576141,
5.37));
#43646=CARTESIAN_POINT('Ctrl Pts',(-0.0969815403223038,-0.545685684680939,
5.4));
#43647=CARTESIAN_POINT('Ctrl Pts',(-0.0969815403223038,-0.545685684680939,
5.37));
#43648=CARTESIAN_POINT('',(-0.110300078988075,-0.599147474765778,5.4));
#43649=CARTESIAN_POINT('Ctrl Pts',(-0.110300078988075,-0.599147474765778,
5.4));
#43650=CARTESIAN_POINT('Ctrl Pts',(-0.110300078988075,-0.569884097576141,
5.4));
#43651=CARTESIAN_POINT('Ctrl Pts',(-0.0969815403223038,-0.545685684680939,
5.4));
#43652=CARTESIAN_POINT('',(-0.110300078988075,-0.599147474765778,5.37));
#43653=CARTESIAN_POINT('',(-0.110300078988075,-0.599147474765778,5.4));
#43654=CARTESIAN_POINT('Ctrl Pts',(-0.110300078988075,-0.599147474765778,
5.37));
#43655=CARTESIAN_POINT('Ctrl Pts',(-0.110300078988075,-0.569884097576141,
5.37));
#43656=CARTESIAN_POINT('Ctrl Pts',(-0.0969815403223038,-0.545685684680939,
5.37));
#43657=CARTESIAN_POINT('Ctrl Pts',(-0.0750341564416885,-0.68112221956253,
5.4));
#43658=CARTESIAN_POINT('Ctrl Pts',(-0.0750341564416885,-0.68112221956253,
5.37));
#43659=CARTESIAN_POINT('Ctrl Pts',(-0.110300078988075,-0.649045145511627,
5.4));
#43660=CARTESIAN_POINT('Ctrl Pts',(-0.110300078988075,-0.649045145511627,
5.37));
#43661=CARTESIAN_POINT('Ctrl Pts',(-0.110300078988075,-0.599147474765778,
5.4));
#43662=CARTESIAN_POINT('Ctrl Pts',(-0.110300078988075,-0.599147474765778,
5.37));
#43663=CARTESIAN_POINT('',(-0.0750341564416885,-0.68112221956253,5.4));
#43664=CARTESIAN_POINT('Ctrl Pts',(-0.0750341564416885,-0.68112221956253,
5.4));
#43665=CARTESIAN_POINT('Ctrl Pts',(-0.110300078988075,-0.649045145511627,
5.4));
#43666=CARTESIAN_POINT('Ctrl Pts',(-0.110300078988075,-0.599147474765778,
5.4));
#43667=CARTESIAN_POINT('',(-0.0750341564416885,-0.68112221956253,5.37));
#43668=CARTESIAN_POINT('',(-0.0750341564416885,-0.68112221956253,5.4));
#43669=CARTESIAN_POINT('Ctrl Pts',(-0.0750341564416885,-0.68112221956253,
5.37));
#43670=CARTESIAN_POINT('Ctrl Pts',(-0.110300078988075,-0.649045145511627,
5.37));
#43671=CARTESIAN_POINT('Ctrl Pts',(-0.110300078988075,-0.599147474765778,
5.37));
#43672=CARTESIAN_POINT('Ctrl Pts',(0.0258867591619492,-0.713199293613434,
5.4));
#43673=CARTESIAN_POINT('Ctrl Pts',(0.0258867591619492,-0.713199293613434,
5.37));
#43674=CARTESIAN_POINT('Ctrl Pts',(-0.0397679954767227,-0.713199293613434,
5.4));
#43675=CARTESIAN_POINT('Ctrl Pts',(-0.0397679954767227,-0.713199293613434,
5.37));
#43676=CARTESIAN_POINT('Ctrl Pts',(-0.0750341564416885,-0.68112221956253,
5.4));
#43677=CARTESIAN_POINT('Ctrl Pts',(-0.0750341564416885,-0.68112221956253,
5.37));
#43678=CARTESIAN_POINT('',(0.0258867591619492,-0.713199293613434,5.4));
#43679=CARTESIAN_POINT('Ctrl Pts',(0.0258867591619492,-0.713199293613434,
5.4));
#43680=CARTESIAN_POINT('Ctrl Pts',(-0.0397679954767227,-0.713199293613434,
5.4));
#43681=CARTESIAN_POINT('Ctrl Pts',(-0.0750341564416885,-0.68112221956253,
5.4));
#43682=CARTESIAN_POINT('',(0.0258867591619492,-0.713199293613434,5.37));
#43683=CARTESIAN_POINT('',(0.0258867591619492,-0.713199293613434,5.4));
#43684=CARTESIAN_POINT('Ctrl Pts',(0.0258867591619492,-0.713199293613434,
5.37));
#43685=CARTESIAN_POINT('Ctrl Pts',(-0.0397679954767227,-0.713199293613434,
5.37));
#43686=CARTESIAN_POINT('Ctrl Pts',(-0.0750341564416885,-0.68112221956253,
5.37));
#43687=CARTESIAN_POINT('Ctrl Pts',(0.100357994437218,-0.700068271160126,
5.4));
#43688=CARTESIAN_POINT('Ctrl Pts',(0.100357994437218,-0.700068271160126,
5.37));
#43689=CARTESIAN_POINT('Ctrl Pts',(0.0656547397375107,-0.713199293613434,
5.4));
#43690=CARTESIAN_POINT('Ctrl Pts',(0.0656547397375107,-0.713199293613434,
5.37));
#43691=CARTESIAN_POINT('Ctrl Pts',(0.0258867591619492,-0.713199293613434,
5.4));
#43692=CARTESIAN_POINT('Ctrl Pts',(0.0258867591619492,-0.713199293613434,
5.37));
#43693=CARTESIAN_POINT('',(0.100357994437218,-0.700068271160126,5.4));
#43694=CARTESIAN_POINT('Ctrl Pts',(0.100357994437218,-0.700068271160126,
5.4));
#43695=CARTESIAN_POINT('Ctrl Pts',(0.0656547397375107,-0.713199293613434,
5.4));
#43696=CARTESIAN_POINT('Ctrl Pts',(0.0258867591619492,-0.713199293613434,
5.4));
#43697=CARTESIAN_POINT('',(0.100357994437218,-0.700068271160126,5.37));
#43698=CARTESIAN_POINT('',(0.100357994437218,-0.700068271160126,5.4));
#43699=CARTESIAN_POINT('Ctrl Pts',(0.100357994437218,-0.700068271160126,
5.37));
#43700=CARTESIAN_POINT('Ctrl Pts',(0.0656547397375107,-0.713199293613434,
5.37));
#43701=CARTESIAN_POINT('Ctrl Pts',(0.0258867591619492,-0.713199293613434,
5.37));
#43702=CARTESIAN_POINT('Ctrl Pts',(0.172578319907188,-0.655047810077667,
5.4));
#43703=CARTESIAN_POINT('Ctrl Pts',(0.172578319907188,-0.655047810077667,
5.37));
#43704=CARTESIAN_POINT('Ctrl Pts',(0.135061249136925,-0.686937367916107,
5.4));
#43705=CARTESIAN_POINT('Ctrl Pts',(0.135061249136925,-0.686937367916107,
5.37));
#43706=CARTESIAN_POINT('Ctrl Pts',(0.100357994437218,-0.700068271160126,
5.4));
#43707=CARTESIAN_POINT('Ctrl Pts',(0.100357994437218,-0.700068271160126,
5.37));
#43708=CARTESIAN_POINT('',(0.172578319907188,-0.655047810077667,5.4));
#43709=CARTESIAN_POINT('Ctrl Pts',(0.172578319907188,-0.655047810077667,
5.4));
#43710=CARTESIAN_POINT('Ctrl Pts',(0.135061249136925,-0.686937367916107,
5.4));
#43711=CARTESIAN_POINT('Ctrl Pts',(0.100357994437218,-0.700068271160126,
5.4));
#43712=CARTESIAN_POINT('',(0.172578319907188,-0.655047810077667,5.37));
#43713=CARTESIAN_POINT('',(0.172578319907188,-0.655047810077667,5.4));
#43714=CARTESIAN_POINT('Ctrl Pts',(0.172578319907188,-0.655047810077667,
5.37));
#43715=CARTESIAN_POINT('Ctrl Pts',(0.135061249136925,-0.686937367916107,
5.37));
#43716=CARTESIAN_POINT('Ctrl Pts',(0.100357994437218,-0.700068271160126,
5.37));
#43717=CARTESIAN_POINT('Ctrl Pts',(0.186084732413292,-0.704195177555084,
5.4));
#43718=CARTESIAN_POINT('Ctrl Pts',(0.186084732413292,-0.704195177555084,
5.37));
#43719=CARTESIAN_POINT('Ctrl Pts',(0.175579771399498,-0.683185613155365,
5.4));
#43720=CARTESIAN_POINT('Ctrl Pts',(0.175579771399498,-0.683185613155365,
5.37));
#43721=CARTESIAN_POINT('Ctrl Pts',(0.172578319907188,-0.655047810077667,
5.4));
#43722=CARTESIAN_POINT('Ctrl Pts',(0.172578319907188,-0.655047810077667,
5.37));
#43723=CARTESIAN_POINT('',(0.186084732413292,-0.704195177555084,5.4));
#43724=CARTESIAN_POINT('Ctrl Pts',(0.186084732413292,-0.704195177555084,
5.4));
#43725=CARTESIAN_POINT('Ctrl Pts',(0.175579771399498,-0.683185613155365,
5.4));
#43726=CARTESIAN_POINT('Ctrl Pts',(0.172578319907188,-0.655047810077667,
5.4));
#43727=CARTESIAN_POINT('',(0.186084732413292,-0.704195177555084,5.37));
#43728=CARTESIAN_POINT('',(0.186084732413292,-0.704195177555084,5.4));
#43729=CARTESIAN_POINT('Ctrl Pts',(0.186084732413292,-0.704195177555084,
5.37));
#43730=CARTESIAN_POINT('Ctrl Pts',(0.175579771399498,-0.683185613155365,
5.37));
#43731=CARTESIAN_POINT('Ctrl Pts',(0.172578319907188,-0.655047810077667,
5.37));
#43732=CARTESIAN_POINT('Origin',(0.256616577506065,-0.704195177555084,5.4));
#43733=CARTESIAN_POINT('',(0.128308288753032,-0.704195177555084,5.4));
#43734=CARTESIAN_POINT('',(0.256616577506065,-0.704195177555084,5.37));
#43735=CARTESIAN_POINT('Origin',(0.0731582492589951,-0.50497961640358,5.37));
#43736=CARTESIAN_POINT('Ctrl Pts',(2.58492515981197,0.650545740127563,5.4));
#43737=CARTESIAN_POINT('Ctrl Pts',(2.58492515981197,0.650545740127563,5.37));
#43738=CARTESIAN_POINT('Ctrl Pts',(2.53840397298336,0.650545740127563,5.4));
#43739=CARTESIAN_POINT('Ctrl Pts',(2.53840397298336,0.650545740127563,5.37));
#43740=CARTESIAN_POINT('Ctrl Pts',(2.51064155995846,0.611152821779251,5.4));
#43741=CARTESIAN_POINT('Ctrl Pts',(2.51064155995846,0.611152821779251,5.37));
#43742=CARTESIAN_POINT('',(2.58492515981197,0.650545740127563,5.4));
#43743=CARTESIAN_POINT('',(2.51064155995846,0.611152821779251,5.4));
#43744=CARTESIAN_POINT('Ctrl Pts',(2.58492515981197,0.650545740127563,5.4));
#43745=CARTESIAN_POINT('Ctrl Pts',(2.53840397298336,0.650545740127563,5.4));
#43746=CARTESIAN_POINT('Ctrl Pts',(2.51064155995846,0.611152821779251,5.4));
#43747=CARTESIAN_POINT('',(2.58492515981197,0.650545740127563,5.37));
#43748=CARTESIAN_POINT('',(2.58492515981197,0.650545740127563,5.4));
#43749=CARTESIAN_POINT('',(2.51064155995846,0.611152821779251,5.37));
#43750=CARTESIAN_POINT('Ctrl Pts',(2.58492515981197,0.650545740127563,5.37));
#43751=CARTESIAN_POINT('Ctrl Pts',(2.53840397298336,0.650545740127563,5.37));
#43752=CARTESIAN_POINT('Ctrl Pts',(2.51064155995846,0.611152821779251,5.37));
#43753=CARTESIAN_POINT('',(2.51064155995846,0.611152821779251,5.4));
#43754=CARTESIAN_POINT('Ctrl Pts',(2.66389845311642,0.605900430679321,5.4));
#43755=CARTESIAN_POINT('Ctrl Pts',(2.66389845311642,0.605900430679321,5.37));
#43756=CARTESIAN_POINT('Ctrl Pts',(2.63219641149044,0.650545740127563,5.4));
#43757=CARTESIAN_POINT('Ctrl Pts',(2.63219641149044,0.650545740127563,5.37));
#43758=CARTESIAN_POINT('Ctrl Pts',(2.58492515981197,0.650545740127563,5.4));
#43759=CARTESIAN_POINT('Ctrl Pts',(2.58492515981197,0.650545740127563,5.37));
#43760=CARTESIAN_POINT('',(2.66389845311642,0.605900430679321,5.4));
#43761=CARTESIAN_POINT('Ctrl Pts',(2.66389845311642,0.605900430679321,5.4));
#43762=CARTESIAN_POINT('Ctrl Pts',(2.63219641149044,0.650545740127563,5.4));
#43763=CARTESIAN_POINT('Ctrl Pts',(2.58492515981197,0.650545740127563,5.4));
#43764=CARTESIAN_POINT('',(2.66389845311642,0.605900430679321,5.37));
#43765=CARTESIAN_POINT('',(2.66389845311642,0.605900430679321,5.4));
#43766=CARTESIAN_POINT('Ctrl Pts',(2.66389845311642,0.605900430679321,5.37));
#43767=CARTESIAN_POINT('Ctrl Pts',(2.63219641149044,0.650545740127563,5.37));
#43768=CARTESIAN_POINT('Ctrl Pts',(2.58492515981197,0.650545740127563,5.37));
#43769=CARTESIAN_POINT('Ctrl Pts',(2.69560049474239,0.425443404912949,5.4));
#43770=CARTESIAN_POINT('Ctrl Pts',(2.69560049474239,0.425443404912949,5.37));
#43771=CARTESIAN_POINT('Ctrl Pts',(2.69560049474239,0.561255151033402,5.4));
#43772=CARTESIAN_POINT('Ctrl Pts',(2.69560049474239,0.561255151033402,5.37));
#43773=CARTESIAN_POINT('Ctrl Pts',(2.66389845311642,0.605900430679321,5.4));
#43774=CARTESIAN_POINT('Ctrl Pts',(2.66389845311642,0.605900430679321,5.37));
#43775=CARTESIAN_POINT('',(2.69560049474239,0.425443404912949,5.4));
#43776=CARTESIAN_POINT('Ctrl Pts',(2.69560049474239,0.425443404912949,5.4));
#43777=CARTESIAN_POINT('Ctrl Pts',(2.69560049474239,0.561255151033402,5.4));
#43778=CARTESIAN_POINT('Ctrl Pts',(2.66389845311642,0.605900430679321,5.4));
#43779=CARTESIAN_POINT('',(2.69560049474239,0.425443404912949,5.37));
#43780=CARTESIAN_POINT('',(2.69560049474239,0.425443404912949,5.4));
#43781=CARTESIAN_POINT('Ctrl Pts',(2.69560049474239,0.425443404912949,5.37));
#43782=CARTESIAN_POINT('Ctrl Pts',(2.69560049474239,0.561255151033402,5.37));
#43783=CARTESIAN_POINT('Ctrl Pts',(2.66389845311642,0.605900430679321,5.37));
#43784=CARTESIAN_POINT('Ctrl Pts',(2.66389845311642,0.245361530780792,5.4));
#43785=CARTESIAN_POINT('Ctrl Pts',(2.66389845311642,0.245361530780792,5.37));
#43786=CARTESIAN_POINT('Ctrl Pts',(2.69560049474239,0.290381991863251,5.4));
#43787=CARTESIAN_POINT('Ctrl Pts',(2.69560049474239,0.290381991863251,5.37));
#43788=CARTESIAN_POINT('Ctrl Pts',(2.69560049474239,0.425443404912949,5.4));
#43789=CARTESIAN_POINT('Ctrl Pts',(2.69560049474239,0.425443404912949,5.37));
#43790=CARTESIAN_POINT('',(2.66389845311642,0.245361530780792,5.4));
#43791=CARTESIAN_POINT('Ctrl Pts',(2.66389845311642,0.245361530780792,5.4));
#43792=CARTESIAN_POINT('Ctrl Pts',(2.69560049474239,0.290381991863251,5.4));
#43793=CARTESIAN_POINT('Ctrl Pts',(2.69560049474239,0.425443404912949,5.4));
#43794=CARTESIAN_POINT('',(2.66389845311642,0.245361530780792,5.37));
#43795=CARTESIAN_POINT('',(2.66389845311642,0.245361530780792,5.4));
#43796=CARTESIAN_POINT('Ctrl Pts',(2.66389845311642,0.245361530780792,5.37));
#43797=CARTESIAN_POINT('Ctrl Pts',(2.69560049474239,0.290381991863251,5.37));
#43798=CARTESIAN_POINT('Ctrl Pts',(2.69560049474239,0.425443404912949,5.37));
#43799=CARTESIAN_POINT('Ctrl Pts',(2.58567522466183,0.200341069698334,5.4));
#43800=CARTESIAN_POINT('Ctrl Pts',(2.58567522466183,0.200341069698334,5.37));
#43801=CARTESIAN_POINT('Ctrl Pts',(2.63219641149044,0.200341069698334,5.4));
#43802=CARTESIAN_POINT('Ctrl Pts',(2.63219641149044,0.200341069698334,5.37));
#43803=CARTESIAN_POINT('Ctrl Pts',(2.66389845311642,0.245361530780792,5.4));
#43804=CARTESIAN_POINT('Ctrl Pts',(2.66389845311642,0.245361530780792,5.37));
#43805=CARTESIAN_POINT('',(2.58567522466183,0.200341069698334,5.4));
#43806=CARTESIAN_POINT('Ctrl Pts',(2.58567522466183,0.200341069698334,5.4));
#43807=CARTESIAN_POINT('Ctrl Pts',(2.63219641149044,0.200341069698334,5.4));
#43808=CARTESIAN_POINT('Ctrl Pts',(2.66389845311642,0.245361530780792,5.4));
#43809=CARTESIAN_POINT('',(2.58567522466183,0.200341069698334,5.37));
#43810=CARTESIAN_POINT('',(2.58567522466183,0.200341069698334,5.4));
#43811=CARTESIAN_POINT('Ctrl Pts',(2.58567522466183,0.200341069698334,5.37));
#43812=CARTESIAN_POINT('Ctrl Pts',(2.63219641149044,0.200341069698334,5.37));
#43813=CARTESIAN_POINT('Ctrl Pts',(2.66389845311642,0.245361530780792,5.37));
#43814=CARTESIAN_POINT('Ctrl Pts',(2.5074524730444,0.245173954963684,5.4));
#43815=CARTESIAN_POINT('Ctrl Pts',(2.5074524730444,0.245173954963684,5.37));
#43816=CARTESIAN_POINT('Ctrl Pts',(2.53915451467037,0.200341069698334,5.4));
#43817=CARTESIAN_POINT('Ctrl Pts',(2.53915451467037,0.200341069698334,5.37));
#43818=CARTESIAN_POINT('Ctrl Pts',(2.58567522466183,0.200341069698334,5.4));
#43819=CARTESIAN_POINT('Ctrl Pts',(2.58567522466183,0.200341069698334,5.37));
#43820=CARTESIAN_POINT('',(2.5074524730444,0.245173954963684,5.4));
#43821=CARTESIAN_POINT('Ctrl Pts',(2.5074524730444,0.245173954963684,5.4));
#43822=CARTESIAN_POINT('Ctrl Pts',(2.53915451467037,0.200341069698334,5.4));
#43823=CARTESIAN_POINT('Ctrl Pts',(2.58567522466183,0.200341069698334,5.4));
#43824=CARTESIAN_POINT('',(2.5074524730444,0.245173954963684,5.37));
#43825=CARTESIAN_POINT('',(2.5074524730444,0.245173954963684,5.4));
#43826=CARTESIAN_POINT('Ctrl Pts',(2.5074524730444,0.245173954963684,5.37));
#43827=CARTESIAN_POINT('Ctrl Pts',(2.53915451467037,0.200341069698334,5.37));
#43828=CARTESIAN_POINT('Ctrl Pts',(2.58567522466183,0.200341069698334,5.37));
#43829=CARTESIAN_POINT('Ctrl Pts',(2.47575043141842,0.425443404912949,5.4));
#43830=CARTESIAN_POINT('Ctrl Pts',(2.47575043141842,0.425443404912949,5.37));
#43831=CARTESIAN_POINT('Ctrl Pts',(2.47575043141842,0.290006840229034,5.4));
#43832=CARTESIAN_POINT('Ctrl Pts',(2.47575043141842,0.290006840229034,5.37));
#43833=CARTESIAN_POINT('Ctrl Pts',(2.5074524730444,0.245173954963684,5.4));
#43834=CARTESIAN_POINT('Ctrl Pts',(2.5074524730444,0.245173954963684,5.37));
#43835=CARTESIAN_POINT('',(2.47575043141842,0.425443404912949,5.4));
#43836=CARTESIAN_POINT('Ctrl Pts',(2.47575043141842,0.425443404912949,5.4));
#43837=CARTESIAN_POINT('Ctrl Pts',(2.47575043141842,0.290006840229034,5.4));
#43838=CARTESIAN_POINT('Ctrl Pts',(2.5074524730444,0.245173954963684,5.4));
#43839=CARTESIAN_POINT('',(2.47575043141842,0.425443404912949,5.37));
#43840=CARTESIAN_POINT('',(2.47575043141842,0.425443404912949,5.4));
#43841=CARTESIAN_POINT('Ctrl Pts',(2.47575043141842,0.425443404912949,5.37));
#43842=CARTESIAN_POINT('Ctrl Pts',(2.47575043141842,0.290006840229034,5.37));
#43843=CARTESIAN_POINT('Ctrl Pts',(2.5074524730444,0.245173954963684,5.37));
#43844=CARTESIAN_POINT('Ctrl Pts',(2.51064155995846,0.611152821779251,5.4));
#43845=CARTESIAN_POINT('Ctrl Pts',(2.51064155995846,0.611152821779251,5.37));
#43846=CARTESIAN_POINT('Ctrl Pts',(2.47575043141842,0.560879969596863,5.4));
#43847=CARTESIAN_POINT('Ctrl Pts',(2.47575043141842,0.560879969596863,5.37));
#43848=CARTESIAN_POINT('Ctrl Pts',(2.47575043141842,0.425443404912949,5.4));
#43849=CARTESIAN_POINT('Ctrl Pts',(2.47575043141842,0.425443404912949,5.37));
#43850=CARTESIAN_POINT('Ctrl Pts',(2.51064155995846,0.611152821779251,5.4));
#43851=CARTESIAN_POINT('Ctrl Pts',(2.47575043141842,0.560879969596863,5.4));
#43852=CARTESIAN_POINT('Ctrl Pts',(2.47575043141842,0.425443404912949,5.4));
#43853=CARTESIAN_POINT('Ctrl Pts',(2.51064155995846,0.611152821779251,5.37));
#43854=CARTESIAN_POINT('Ctrl Pts',(2.47575043141842,0.560879969596863,5.37));
#43855=CARTESIAN_POINT('Ctrl Pts',(2.47575043141842,0.425443404912949,5.37));
#43856=CARTESIAN_POINT('Ctrl Pts',(2.68565843999386,0.177268081903458,5.4));
#43857=CARTESIAN_POINT('Ctrl Pts',(2.68565843999386,0.177268081903458,5.37));
#43858=CARTESIAN_POINT('Ctrl Pts',(2.64607809484005,0.144815826416016,5.4));
#43859=CARTESIAN_POINT('Ctrl Pts',(2.64607809484005,0.144815826416016,5.37));
#43860=CARTESIAN_POINT('Ctrl Pts',(2.58567522466183,0.144815826416016,5.4));
#43861=CARTESIAN_POINT('Ctrl Pts',(2.58567522466183,0.144815826416016,5.37));
#43862=CARTESIAN_POINT('',(2.68565843999386,0.177268081903458,5.4));
#43863=CARTESIAN_POINT('',(2.58567522466183,0.144815826416016,5.4));
#43864=CARTESIAN_POINT('Ctrl Pts',(2.68565843999386,0.177268081903458,5.4));
#43865=CARTESIAN_POINT('Ctrl Pts',(2.64607809484005,0.144815826416016,5.4));
#43866=CARTESIAN_POINT('Ctrl Pts',(2.58567522466183,0.144815826416016,5.4));
#43867=CARTESIAN_POINT('',(2.68565843999386,0.177268081903458,5.37));
#43868=CARTESIAN_POINT('',(2.68565843999386,0.177268081903458,5.4));
#43869=CARTESIAN_POINT('',(2.58567522466183,0.144815826416016,5.37));
#43870=CARTESIAN_POINT('Ctrl Pts',(2.68565843999386,0.177268081903458,5.37));
#43871=CARTESIAN_POINT('Ctrl Pts',(2.64607809484005,0.144815826416016,5.37));
#43872=CARTESIAN_POINT('Ctrl Pts',(2.58567522466183,0.144815826416016,5.37));
#43873=CARTESIAN_POINT('',(2.58567522466183,0.144815826416016,5.4));
#43874=CARTESIAN_POINT('Ctrl Pts',(2.74512289464474,0.269184851646423,5.4));
#43875=CARTESIAN_POINT('Ctrl Pts',(2.74512289464474,0.269184851646423,5.37));
#43876=CARTESIAN_POINT('Ctrl Pts',(2.72523878514767,0.2097203373909,5.4));
#43877=CARTESIAN_POINT('Ctrl Pts',(2.72523878514767,0.2097203373909,5.37));
#43878=CARTESIAN_POINT('Ctrl Pts',(2.68565843999386,0.177268081903458,5.4));
#43879=CARTESIAN_POINT('Ctrl Pts',(2.68565843999386,0.177268081903458,5.37));
#43880=CARTESIAN_POINT('',(2.74512289464474,0.269184851646423,5.4));
#43881=CARTESIAN_POINT('Ctrl Pts',(2.74512289464474,0.269184851646423,5.4));
#43882=CARTESIAN_POINT('Ctrl Pts',(2.72523878514767,0.2097203373909,5.4));
#43883=CARTESIAN_POINT('Ctrl Pts',(2.68565843999386,0.177268081903458,5.4));
#43884=CARTESIAN_POINT('',(2.74512289464474,0.269184851646423,5.37));
#43885=CARTESIAN_POINT('',(2.74512289464474,0.269184851646423,5.4));
#43886=CARTESIAN_POINT('Ctrl Pts',(2.74512289464474,0.269184851646423,5.37));
#43887=CARTESIAN_POINT('Ctrl Pts',(2.72523878514767,0.2097203373909,5.37));
#43888=CARTESIAN_POINT('Ctrl Pts',(2.68565843999386,0.177268081903458,5.37));
#43889=CARTESIAN_POINT('Ctrl Pts',(2.76500700414181,0.425443404912949,5.4));
#43890=CARTESIAN_POINT('Ctrl Pts',(2.76500700414181,0.425443404912949,5.37));
#43891=CARTESIAN_POINT('Ctrl Pts',(2.76500700414181,0.328649395704269,5.4));
#43892=CARTESIAN_POINT('Ctrl Pts',(2.76500700414181,0.328649395704269,5.37));
#43893=CARTESIAN_POINT('Ctrl Pts',(2.74512289464474,0.269184851646423,5.4));
#43894=CARTESIAN_POINT('Ctrl Pts',(2.74512289464474,0.269184851646423,5.37));
#43895=CARTESIAN_POINT('',(2.76500700414181,0.425443404912949,5.4));
#43896=CARTESIAN_POINT('Ctrl Pts',(2.76500700414181,0.425443404912949,5.4));
#43897=CARTESIAN_POINT('Ctrl Pts',(2.76500700414181,0.328649395704269,5.4));
#43898=CARTESIAN_POINT('Ctrl Pts',(2.74512289464474,0.269184851646423,5.4));
#43899=CARTESIAN_POINT('',(2.76500700414181,0.425443404912949,5.37));
#43900=CARTESIAN_POINT('',(2.76500700414181,0.425443404912949,5.4));
#43901=CARTESIAN_POINT('Ctrl Pts',(2.76500700414181,0.425443404912949,5.37));
#43902=CARTESIAN_POINT('Ctrl Pts',(2.76500700414181,0.328649395704269,5.37));
#43903=CARTESIAN_POINT('Ctrl Pts',(2.74512289464474,0.269184851646423,5.37));
#43904=CARTESIAN_POINT('Ctrl Pts',(2.75262640416622,0.555440002679825,5.4));
#43905=CARTESIAN_POINT('Ctrl Pts',(2.75262640416622,0.555440002679825,5.37));
#43906=CARTESIAN_POINT('Ctrl Pts',(2.76500700414181,0.507230573892593,5.4));
#43907=CARTESIAN_POINT('Ctrl Pts',(2.76500700414181,0.507230573892593,5.37));
#43908=CARTESIAN_POINT('Ctrl Pts',(2.76500700414181,0.425443404912949,5.4));
#43909=CARTESIAN_POINT('Ctrl Pts',(2.76500700414181,0.425443404912949,5.37));
#43910=CARTESIAN_POINT('',(2.75262640416622,0.555440002679825,5.4));
#43911=CARTESIAN_POINT('Ctrl Pts',(2.75262640416622,0.555440002679825,5.4));
#43912=CARTESIAN_POINT('Ctrl Pts',(2.76500700414181,0.507230573892593,5.4));
#43913=CARTESIAN_POINT('Ctrl Pts',(2.76500700414181,0.425443404912949,5.4));
#43914=CARTESIAN_POINT('',(2.75262640416622,0.555440002679825,5.37));
#43915=CARTESIAN_POINT('',(2.75262640416622,0.555440002679825,5.4));
#43916=CARTESIAN_POINT('Ctrl Pts',(2.75262640416622,0.555440002679825,5.37));
#43917=CARTESIAN_POINT('Ctrl Pts',(2.76500700414181,0.507230573892593,5.37));
#43918=CARTESIAN_POINT('Ctrl Pts',(2.76500700414181,0.425443404912949,5.37));
#43919=CARTESIAN_POINT('Ctrl Pts',(2.71848581731319,0.63722717165947,5.4));
#43920=CARTESIAN_POINT('Ctrl Pts',(2.71848581731319,0.63722717165947,5.37));
#43921=CARTESIAN_POINT('Ctrl Pts',(2.74024580419064,0.603649401664734,5.4));
#43922=CARTESIAN_POINT('Ctrl Pts',(2.74024580419064,0.603649401664734,5.37));
#43923=CARTESIAN_POINT('Ctrl Pts',(2.75262640416622,0.555440002679825,5.4));
#43924=CARTESIAN_POINT('Ctrl Pts',(2.75262640416622,0.555440002679825,5.37));
#43925=CARTESIAN_POINT('',(2.71848581731319,0.63722717165947,5.4));
#43926=CARTESIAN_POINT('Ctrl Pts',(2.71848581731319,0.63722717165947,5.4));
#43927=CARTESIAN_POINT('Ctrl Pts',(2.74024580419064,0.603649401664734,5.4));
#43928=CARTESIAN_POINT('Ctrl Pts',(2.75262640416622,0.555440002679825,5.4));
#43929=CARTESIAN_POINT('',(2.71848581731319,0.63722717165947,5.37));
#43930=CARTESIAN_POINT('',(2.71848581731319,0.63722717165947,5.4));
#43931=CARTESIAN_POINT('Ctrl Pts',(2.71848581731319,0.63722717165947,5.37));
#43932=CARTESIAN_POINT('Ctrl Pts',(2.74024580419064,0.603649401664734,5.37));
#43933=CARTESIAN_POINT('Ctrl Pts',(2.75262640416622,0.555440002679825,5.37));
#43934=CARTESIAN_POINT('Ctrl Pts',(2.66333578526974,0.688625538349152,5.4));
#43935=CARTESIAN_POINT('Ctrl Pts',(2.66333578526974,0.688625538349152,5.37));
#43936=CARTESIAN_POINT('Ctrl Pts',(2.69672583043575,0.670804941654205,5.4));
#43937=CARTESIAN_POINT('Ctrl Pts',(2.69672583043575,0.670804941654205,5.37));
#43938=CARTESIAN_POINT('Ctrl Pts',(2.71848581731319,0.63722717165947,5.4));
#43939=CARTESIAN_POINT('Ctrl Pts',(2.71848581731319,0.63722717165947,5.37));
#43940=CARTESIAN_POINT('',(2.66333578526974,0.688625538349152,5.4));
#43941=CARTESIAN_POINT('Ctrl Pts',(2.66333578526974,0.688625538349152,5.4));
#43942=CARTESIAN_POINT('Ctrl Pts',(2.69672583043575,0.670804941654205,5.4));
#43943=CARTESIAN_POINT('Ctrl Pts',(2.71848581731319,0.63722717165947,5.4));
#43944=CARTESIAN_POINT('',(2.66333578526974,0.688625538349152,5.37));
#43945=CARTESIAN_POINT('',(2.66333578526974,0.688625538349152,5.4));
#43946=CARTESIAN_POINT('Ctrl Pts',(2.66333578526974,0.688625538349152,5.37));
#43947=CARTESIAN_POINT('Ctrl Pts',(2.69672583043575,0.670804941654205,5.37));
#43948=CARTESIAN_POINT('Ctrl Pts',(2.71848581731319,0.63722717165947,5.37));
#43949=CARTESIAN_POINT('Ctrl Pts',(2.58567522466183,0.706446135044098,5.4));
#43950=CARTESIAN_POINT('Ctrl Pts',(2.58567522466183,0.706446135044098,5.37));
#43951=CARTESIAN_POINT('Ctrl Pts',(2.62994574010372,0.706446135044098,5.4));
#43952=CARTESIAN_POINT('Ctrl Pts',(2.62994574010372,0.706446135044098,5.37));
#43953=CARTESIAN_POINT('Ctrl Pts',(2.66333578526974,0.688625538349152,5.4));
#43954=CARTESIAN_POINT('Ctrl Pts',(2.66333578526974,0.688625538349152,5.37));
#43955=CARTESIAN_POINT('',(2.58567522466183,0.706446135044098,5.4));
#43956=CARTESIAN_POINT('Ctrl Pts',(2.58567522466183,0.706446135044098,5.4));
#43957=CARTESIAN_POINT('Ctrl Pts',(2.62994574010372,0.706446135044098,5.4));
#43958=CARTESIAN_POINT('Ctrl Pts',(2.66333578526974,0.688625538349152,5.4));
#43959=CARTESIAN_POINT('',(2.58567522466183,0.706446135044098,5.37));
#43960=CARTESIAN_POINT('',(2.58567522466183,0.706446135044098,5.4));
#43961=CARTESIAN_POINT('Ctrl Pts',(2.58567522466183,0.706446135044098,5.37));
#43962=CARTESIAN_POINT('Ctrl Pts',(2.62994574010372,0.706446135044098,5.37));
#43963=CARTESIAN_POINT('Ctrl Pts',(2.66333578526974,0.688625538349152,5.37));
#43964=CARTESIAN_POINT('Ctrl Pts',(2.48606775701046,0.674181485176086,5.4));
#43965=CARTESIAN_POINT('Ctrl Pts',(2.48606775701046,0.674181485176086,5.37));
#43966=CARTESIAN_POINT('Ctrl Pts',(2.52564810216427,0.706446135044098,5.4));
#43967=CARTESIAN_POINT('Ctrl Pts',(2.52564810216427,0.706446135044098,5.37));
#43968=CARTESIAN_POINT('Ctrl Pts',(2.58567522466183,0.706446135044098,5.4));
#43969=CARTESIAN_POINT('Ctrl Pts',(2.58567522466183,0.706446135044098,5.37));
#43970=CARTESIAN_POINT('',(2.48606775701046,0.674181485176086,5.4));
#43971=CARTESIAN_POINT('Ctrl Pts',(2.48606775701046,0.674181485176086,5.4));
#43972=CARTESIAN_POINT('Ctrl Pts',(2.52564810216427,0.706446135044098,5.4));
#43973=CARTESIAN_POINT('Ctrl Pts',(2.58567522466183,0.706446135044098,5.4));
#43974=CARTESIAN_POINT('',(2.48606775701046,0.674181485176086,5.37));
#43975=CARTESIAN_POINT('',(2.48606775701046,0.674181485176086,5.4));
#43976=CARTESIAN_POINT('Ctrl Pts',(2.48606775701046,0.674181485176086,5.37));
#43977=CARTESIAN_POINT('Ctrl Pts',(2.52564810216427,0.706446135044098,5.37));
#43978=CARTESIAN_POINT('Ctrl Pts',(2.58567522466183,0.706446135044098,5.37));
#43979=CARTESIAN_POINT('Ctrl Pts',(2.42641542851925,0.582452261447907,5.4));
#43980=CARTESIAN_POINT('Ctrl Pts',(2.42641542851925,0.582452261447907,5.37));
#43981=CARTESIAN_POINT('Ctrl Pts',(2.44648693501949,0.641916805505753,5.4));
#43982=CARTESIAN_POINT('Ctrl Pts',(2.44648693501949,0.641916805505753,5.37));
#43983=CARTESIAN_POINT('Ctrl Pts',(2.48606775701046,0.674181485176086,5.4));
#43984=CARTESIAN_POINT('Ctrl Pts',(2.48606775701046,0.674181485176086,5.37));
#43985=CARTESIAN_POINT('',(2.42641542851925,0.582452261447907,5.4));
#43986=CARTESIAN_POINT('Ctrl Pts',(2.42641542851925,0.582452261447907,5.4));
#43987=CARTESIAN_POINT('Ctrl Pts',(2.44648693501949,0.641916805505753,5.4));
#43988=CARTESIAN_POINT('Ctrl Pts',(2.48606775701046,0.674181485176086,5.4));
#43989=CARTESIAN_POINT('',(2.42641542851925,0.582452261447907,5.37));
#43990=CARTESIAN_POINT('',(2.42641542851925,0.582452261447907,5.4));
#43991=CARTESIAN_POINT('Ctrl Pts',(2.42641542851925,0.582452261447907,5.37));
#43992=CARTESIAN_POINT('Ctrl Pts',(2.44648693501949,0.641916805505753,5.37));
#43993=CARTESIAN_POINT('Ctrl Pts',(2.48606775701046,0.674181485176086,5.37));
#43994=CARTESIAN_POINT('Ctrl Pts',(2.406343922019,0.425443404912949,5.4));
#43995=CARTESIAN_POINT('Ctrl Pts',(2.406343922019,0.425443404912949,5.37));
#43996=CARTESIAN_POINT('Ctrl Pts',(2.406343922019,0.522987747192383,5.4));
#43997=CARTESIAN_POINT('Ctrl Pts',(2.406343922019,0.522987747192383,5.37));
#43998=CARTESIAN_POINT('Ctrl Pts',(2.42641542851925,0.582452261447907,5.4));
#43999=CARTESIAN_POINT('Ctrl Pts',(2.42641542851925,0.582452261447907,5.37));
#44000=CARTESIAN_POINT('',(2.406343922019,0.425443404912949,5.4));
#44001=CARTESIAN_POINT('Ctrl Pts',(2.406343922019,0.425443404912949,5.4));
#44002=CARTESIAN_POINT('Ctrl Pts',(2.406343922019,0.522987747192383,5.4));
#44003=CARTESIAN_POINT('Ctrl Pts',(2.42641542851925,0.582452261447907,5.4));
#44004=CARTESIAN_POINT('',(2.406343922019,0.425443404912949,5.37));
#44005=CARTESIAN_POINT('',(2.406343922019,0.425443404912949,5.4));
#44006=CARTESIAN_POINT('Ctrl Pts',(2.406343922019,0.425443404912949,5.37));
#44007=CARTESIAN_POINT('Ctrl Pts',(2.406343922019,0.522987747192383,5.37));
#44008=CARTESIAN_POINT('Ctrl Pts',(2.42641542851925,0.582452261447907,5.37));
#44009=CARTESIAN_POINT('Ctrl Pts',(2.46074388921261,0.201841765642166,5.4));
#44010=CARTESIAN_POINT('Ctrl Pts',(2.46074388921261,0.201841765642166,5.37));
#44011=CARTESIAN_POINT('Ctrl Pts',(2.406343922019,0.270497941970825,5.4));
#44012=CARTESIAN_POINT('Ctrl Pts',(2.406343922019,0.270497941970825,5.37));
#44013=CARTESIAN_POINT('Ctrl Pts',(2.406343922019,0.425443404912949,5.4));
#44014=CARTESIAN_POINT('Ctrl Pts',(2.406343922019,0.425443404912949,5.37));
#44015=CARTESIAN_POINT('',(2.46074388921261,0.201841765642166,5.4));
#44016=CARTESIAN_POINT('Ctrl Pts',(2.46074388921261,0.201841765642166,5.4));
#44017=CARTESIAN_POINT('Ctrl Pts',(2.406343922019,0.270497941970825,5.4));
#44018=CARTESIAN_POINT('Ctrl Pts',(2.406343922019,0.425443404912949,5.4));
#44019=CARTESIAN_POINT('',(2.46074388921261,0.201841765642166,5.37));
#44020=CARTESIAN_POINT('',(2.46074388921261,0.201841765642166,5.4));
#44021=CARTESIAN_POINT('Ctrl Pts',(2.46074388921261,0.201841765642166,5.37));
#44022=CARTESIAN_POINT('Ctrl Pts',(2.406343922019,0.270497941970825,5.37));
#44023=CARTESIAN_POINT('Ctrl Pts',(2.406343922019,0.425443404912949,5.37));
#44024=CARTESIAN_POINT('Ctrl Pts',(2.58567522466183,0.144815826416016,5.4));
#44025=CARTESIAN_POINT('Ctrl Pts',(2.58567522466183,0.144815826416016,5.37));
#44026=CARTESIAN_POINT('Ctrl Pts',(2.5061392635107,0.144815826416016,5.4));
#44027=CARTESIAN_POINT('Ctrl Pts',(2.5061392635107,0.144815826416016,5.37));
#44028=CARTESIAN_POINT('Ctrl Pts',(2.46074388921261,0.201841765642166,5.4));
#44029=CARTESIAN_POINT('Ctrl Pts',(2.46074388921261,0.201841765642166,5.37));
#44030=CARTESIAN_POINT('Ctrl Pts',(2.58567522466183,0.144815826416016,5.4));
#44031=CARTESIAN_POINT('Ctrl Pts',(2.5061392635107,0.144815826416016,5.4));
#44032=CARTESIAN_POINT('Ctrl Pts',(2.46074388921261,0.201841765642166,5.4));
#44033=CARTESIAN_POINT('Ctrl Pts',(2.58567522466183,0.144815826416016,5.37));
#44034=CARTESIAN_POINT('Ctrl Pts',(2.5061392635107,0.144815826416016,5.37));
#44035=CARTESIAN_POINT('Ctrl Pts',(2.46074388921261,0.201841765642166,5.37));
#44036=CARTESIAN_POINT('Origin',(2.58567546308041,0.425630980730057,5.37));
#44037=CARTESIAN_POINT('Ctrl Pts',(1.70252369344234,0.632912719249725,5.4));
#44038=CARTESIAN_POINT('Ctrl Pts',(1.70252369344234,0.632912719249725,5.37));
#44039=CARTESIAN_POINT('Ctrl Pts',(1.74491833150387,0.670804941654205,5.4));
#44040=CARTESIAN_POINT('Ctrl Pts',(1.74491833150387,0.670804941654205,5.37));
#44041=CARTESIAN_POINT('Ctrl Pts',(1.76255129277706,0.706446135044098,5.4));
#44042=CARTESIAN_POINT('Ctrl Pts',(1.76255129277706,0.706446135044098,5.37));
#44043=CARTESIAN_POINT('',(1.70252369344234,0.632912719249725,5.4));
#44044=CARTESIAN_POINT('',(1.76255129277706,0.706446135044098,5.4));
#44045=CARTESIAN_POINT('Ctrl Pts',(1.70252369344234,0.632912719249725,5.4));
#44046=CARTESIAN_POINT('Ctrl Pts',(1.74491833150387,0.670804941654205,5.4));
#44047=CARTESIAN_POINT('Ctrl Pts',(1.76255129277706,0.706446135044098,5.4));
#44048=CARTESIAN_POINT('',(1.70252369344234,0.632912719249725,5.37));
#44049=CARTESIAN_POINT('',(1.70252369344234,0.632912719249725,5.4));
#44050=CARTESIAN_POINT('',(1.76255129277706,0.706446135044098,5.37));
#44051=CARTESIAN_POINT('Ctrl Pts',(1.70252369344234,0.632912719249725,5.37));
#44052=CARTESIAN_POINT('Ctrl Pts',(1.74491833150387,0.670804941654205,5.37));
#44053=CARTESIAN_POINT('Ctrl Pts',(1.76255129277706,0.706446135044098,5.37));
#44054=CARTESIAN_POINT('',(1.76255129277706,0.706446135044098,5.4));
#44055=CARTESIAN_POINT('Ctrl Pts',(1.60347889363766,0.56838338971138,5.4));
#44056=CARTESIAN_POINT('Ctrl Pts',(1.60347889363766,0.56838338971138,5.37));
#44057=CARTESIAN_POINT('Ctrl Pts',(1.66012953221798,0.595020496845245,5.4));
#44058=CARTESIAN_POINT('Ctrl Pts',(1.66012953221798,0.595020496845245,5.37));
#44059=CARTESIAN_POINT('Ctrl Pts',(1.70252369344234,0.632912719249725,5.4));
#44060=CARTESIAN_POINT('Ctrl Pts',(1.70252369344234,0.632912719249725,5.37));
#44061=CARTESIAN_POINT('',(1.60347889363766,0.56838338971138,5.4));
#44062=CARTESIAN_POINT('Ctrl Pts',(1.60347889363766,0.56838338971138,5.4));
#44063=CARTESIAN_POINT('Ctrl Pts',(1.66012953221798,0.595020496845245,5.4));
#44064=CARTESIAN_POINT('Ctrl Pts',(1.70252369344234,0.632912719249725,5.4));
#44065=CARTESIAN_POINT('',(1.60347889363766,0.56838338971138,5.37));
#44066=CARTESIAN_POINT('',(1.60347889363766,0.56838338971138,5.4));
#44067=CARTESIAN_POINT('Ctrl Pts',(1.60347889363766,0.56838338971138,5.37));
#44068=CARTESIAN_POINT('Ctrl Pts',(1.66012953221798,0.595020496845245,5.37));
#44069=CARTESIAN_POINT('Ctrl Pts',(1.70252369344234,0.632912719249725,5.37));
#44070=CARTESIAN_POINT('Origin',(1.60347889363766,0.503103697299957,5.4));
#44071=CARTESIAN_POINT('',(1.60347889363766,0.503103697299957,5.4));
#44072=CARTESIAN_POINT('',(1.60347889363766,0.251551848649979,5.4));
#44073=CARTESIAN_POINT('',(1.60347889363766,0.503103697299957,5.37));
#44074=CARTESIAN_POINT('',(1.60347889363766,0.503103697299957,5.4));
#44075=CARTESIAN_POINT('',(1.60347889363766,0.503103697299957,5.37));
#44076=CARTESIAN_POINT('Ctrl Pts',(1.67457388341427,0.537994557619095,5.4));
#44077=CARTESIAN_POINT('Ctrl Pts',(1.67457388341427,0.537994557619095,5.37));
#44078=CARTESIAN_POINT('Ctrl Pts',(1.6349930614233,0.514733994007111,5.4));
#44079=CARTESIAN_POINT('Ctrl Pts',(1.6349930614233,0.514733994007111,5.37));
#44080=CARTESIAN_POINT('Ctrl Pts',(1.60347889363766,0.503103697299957,5.4));
#44081=CARTESIAN_POINT('Ctrl Pts',(1.60347889363766,0.503103697299957,5.37));
#44082=CARTESIAN_POINT('',(1.67457388341427,0.537994557619095,5.4));
#44083=CARTESIAN_POINT('Ctrl Pts',(1.67457388341427,0.537994557619095,5.4));
#44084=CARTESIAN_POINT('Ctrl Pts',(1.6349930614233,0.514733994007111,5.4));
#44085=CARTESIAN_POINT('Ctrl Pts',(1.60347889363766,0.503103697299957,5.4));
#44086=CARTESIAN_POINT('',(1.67457388341427,0.537994557619095,5.37));
#44087=CARTESIAN_POINT('',(1.67457388341427,0.537994557619095,5.4));
#44088=CARTESIAN_POINT('Ctrl Pts',(1.67457388341427,0.537994557619095,5.37));
#44089=CARTESIAN_POINT('Ctrl Pts',(1.6349930614233,0.514733994007111,5.37));
#44090=CARTESIAN_POINT('Ctrl Pts',(1.60347889363766,0.503103697299957,5.37));
#44091=CARTESIAN_POINT('Ctrl Pts',(1.73854015767574,0.584515714645386,5.4));
#44092=CARTESIAN_POINT('Ctrl Pts',(1.73854015767574,0.584515714645386,5.37));
#44093=CARTESIAN_POINT('Ctrl Pts',(1.71415422856808,0.561255151033402,5.4));
#44094=CARTESIAN_POINT('Ctrl Pts',(1.71415422856808,0.561255151033402,5.37));
#44095=CARTESIAN_POINT('Ctrl Pts',(1.67457388341427,0.537994557619095,5.4));
#44096=CARTESIAN_POINT('Ctrl Pts',(1.67457388341427,0.537994557619095,5.37));
#44097=CARTESIAN_POINT('',(1.73854015767574,0.584515714645386,5.4));
#44098=CARTESIAN_POINT('Ctrl Pts',(1.73854015767574,0.584515714645386,5.4));
#44099=CARTESIAN_POINT('Ctrl Pts',(1.71415422856808,0.561255151033402,5.4));
#44100=CARTESIAN_POINT('Ctrl Pts',(1.67457388341427,0.537994557619095,5.4));
#44101=CARTESIAN_POINT('',(1.73854015767574,0.584515714645386,5.37));
#44102=CARTESIAN_POINT('',(1.73854015767574,0.584515714645386,5.4));
#44103=CARTESIAN_POINT('Ctrl Pts',(1.73854015767574,0.584515714645386,5.37));
#44104=CARTESIAN_POINT('Ctrl Pts',(1.71415422856808,0.561255151033402,5.37));
#44105=CARTESIAN_POINT('Ctrl Pts',(1.67457388341427,0.537994557619095,5.37));
#44106=CARTESIAN_POINT('Origin',(1.73854015767574,0.154195094108582,5.4));
#44107=CARTESIAN_POINT('',(1.73854015767574,0.154195094108582,5.4));
#44108=CARTESIAN_POINT('',(1.73854015767574,0.0770975470542908,5.4));
#44109=CARTESIAN_POINT('',(1.73854015767574,0.154195094108582,5.37));
#44110=CARTESIAN_POINT('',(1.73854015767574,0.154195094108582,5.4));
#44111=CARTESIAN_POINT('',(1.73854015767574,0.154195094108582,5.37));
#44112=CARTESIAN_POINT('Origin',(1.80607078969479,0.154195094108582,5.4));
#44113=CARTESIAN_POINT('',(1.80607078969479,0.154195094108582,5.4));
#44114=CARTESIAN_POINT('',(0.903035394847393,0.154195094108582,5.4));
#44115=CARTESIAN_POINT('',(1.80607078969479,0.154195094108582,5.37));
#44116=CARTESIAN_POINT('',(1.80607078969479,0.154195094108582,5.4));
#44117=CARTESIAN_POINT('',(1.80607078969479,0.154195094108582,5.37));
#44118=CARTESIAN_POINT('Origin',(1.80607078969479,0.706446135044098,5.4));
#44119=CARTESIAN_POINT('',(1.80607078969479,0.706446135044098,5.4));
#44120=CARTESIAN_POINT('',(1.80607078969479,0.353223067522049,5.4));
#44121=CARTESIAN_POINT('',(1.80607078969479,0.706446135044098,5.37));
#44122=CARTESIAN_POINT('',(1.80607078969479,0.706446135044098,5.4));
#44123=CARTESIAN_POINT('',(1.80607078969479,0.706446135044098,5.37));
#44124=CARTESIAN_POINT('Origin',(1.76255129277706,0.706446135044098,5.4));
#44125=CARTESIAN_POINT('',(0.881275646388531,0.706446135044098,5.4));
#44126=CARTESIAN_POINT('',(1.76255129277706,0.706446135044098,5.37));
#44127=CARTESIAN_POINT('Origin',(1.70477484166622,0.43032061457634,5.37));
#44128=CARTESIAN_POINT('Origin',(-2.53577782213688,0.154195094108582,5.4));
#44129=CARTESIAN_POINT('',(-2.53577782213688,0.154195094108582,5.4));
#44130=CARTESIAN_POINT('',(-2.69485013186932,0.622407937049866,5.4));
#44131=CARTESIAN_POINT('',(-2.38109215733969,-0.301106114497601,5.4));
#44132=CARTESIAN_POINT('',(-2.53577782213688,0.154195094108582,5.37));
#44133=CARTESIAN_POINT('',(-2.53577782213688,0.154195094108582,5.4));
#44134=CARTESIAN_POINT('',(-2.69485013186932,0.622407937049866,5.37));
#44135=CARTESIAN_POINT('',(-2.53577782213688,0.154195094108582,5.37));
#44136=CARTESIAN_POINT('',(-2.69485013186932,0.622407937049866,5.4));
#44137=CARTESIAN_POINT('Origin',(-2.47012294828892,0.154195094108582,5.4));
#44138=CARTESIAN_POINT('',(-2.47012294828892,0.154195094108582,5.4));
#44139=CARTESIAN_POINT('',(-1.23506147414446,0.154195094108582,5.4));
#44140=CARTESIAN_POINT('',(-2.47012294828892,0.154195094108582,5.37));
#44141=CARTESIAN_POINT('',(-2.47012294828892,0.154195094108582,5.4));
#44142=CARTESIAN_POINT('',(-2.47012294828892,0.154195094108582,5.37));
#44143=CARTESIAN_POINT('Origin',(-2.31030030548573,0.614529365301132,5.4));
#44144=CARTESIAN_POINT('',(-2.31030030548573,0.614529365301132,5.4));
#44145=CARTESIAN_POINT('',(-2.28124043684146,0.698229980049323,5.4));
#44146=CARTESIAN_POINT('',(-2.31030030548573,0.614529365301132,5.37));
#44147=CARTESIAN_POINT('',(-2.31030030548573,0.614529365301132,5.4));
#44148=CARTESIAN_POINT('',(-2.31030030548573,0.614529365301132,5.37));
#44149=CARTESIAN_POINT('Origin',(-2.31030030548573,0.154195094108582,5.4));
#44150=CARTESIAN_POINT('',(-2.31030030548573,0.154195094108582,5.4));
#44151=CARTESIAN_POINT('',(-2.31030030548573,0.0770975470542908,5.4));
#44152=CARTESIAN_POINT('',(-2.31030030548573,0.154195094108582,5.37));
#44153=CARTESIAN_POINT('',(-2.31030030548573,0.154195094108582,5.4));
#44154=CARTESIAN_POINT('',(-2.31030030548573,0.154195094108582,5.37));
#44155=CARTESIAN_POINT('Origin',(-2.24014343321323,0.154195094108582,5.4));
#44156=CARTESIAN_POINT('',(-2.24014343321323,0.154195094108582,5.4));
#44157=CARTESIAN_POINT('',(-1.12007171660662,0.154195094108582,5.4));
#44158=CARTESIAN_POINT('',(-2.24014343321323,0.154195094108582,5.37));
#44159=CARTESIAN_POINT('',(-2.24014343321323,0.154195094108582,5.4));
#44160=CARTESIAN_POINT('',(-2.24014343321323,0.154195094108582,5.37));
#44161=CARTESIAN_POINT('Origin',(-2.24014343321323,0.704195106029511,5.4));
#44162=CARTESIAN_POINT('',(-2.24014343321323,0.704195106029511,5.4));
#44163=CARTESIAN_POINT('',(-2.24014343321323,0.352097553014755,5.4));
#44164=CARTESIAN_POINT('',(-2.24014343321323,0.704195106029511,5.37));
#44165=CARTESIAN_POINT('',(-2.24014343321323,0.704195106029511,5.4));
#44166=CARTESIAN_POINT('',(-2.24014343321323,0.704195106029511,5.37));
#44167=CARTESIAN_POINT('Origin',(-2.33806295692921,0.704195106029511,5.4));
#44168=CARTESIAN_POINT('',(-2.33806295692921,0.704195106029511,5.4));
#44169=CARTESIAN_POINT('',(-1.1690314784646,0.704195106029511,5.4));
#44170=CARTESIAN_POINT('',(-2.33806295692921,0.704195106029511,5.37));
#44171=CARTESIAN_POINT('',(-2.33806295692921,0.704195106029511,5.4));
#44172=CARTESIAN_POINT('',(-2.33806295692921,0.704195106029511,5.37));
#44173=CARTESIAN_POINT('Origin',(-2.4697477966547,0.321521157026291,5.4));
#44174=CARTESIAN_POINT('',(-2.4697477966547,0.321521157026291,5.4));
#44175=CARTESIAN_POINT('',(-2.38846377938169,0.557731156184516,5.4));
#44176=CARTESIAN_POINT('',(-2.4697477966547,0.321521157026291,5.37));
#44177=CARTESIAN_POINT('',(-2.4697477966547,0.321521157026291,5.4));
#44178=CARTESIAN_POINT('',(-2.4697477966547,0.321521157026291,5.37));
#44179=CARTESIAN_POINT('Ctrl Pts',(-2.49901111423969,0.233356082439423,
5.4));
#44180=CARTESIAN_POINT('Ctrl Pts',(-2.49901111423969,0.233356082439423,
5.37));
#44181=CARTESIAN_POINT('Ctrl Pts',(-2.48963184654713,0.263369733095169,
5.4));
#44182=CARTESIAN_POINT('Ctrl Pts',(-2.48963184654713,0.263369733095169,
5.37));
#44183=CARTESIAN_POINT('Ctrl Pts',(-2.4697477966547,0.321521157026291,5.4));
#44184=CARTESIAN_POINT('Ctrl Pts',(-2.4697477966547,0.321521157026291,5.37));
#44185=CARTESIAN_POINT('',(-2.49901111423969,0.233356082439423,5.4));
#44186=CARTESIAN_POINT('Ctrl Pts',(-2.49901111423969,0.233356082439423,
5.4));
#44187=CARTESIAN_POINT('Ctrl Pts',(-2.48963184654713,0.263369733095169,
5.4));
#44188=CARTESIAN_POINT('Ctrl Pts',(-2.4697477966547,0.321521157026291,5.4));
#44189=CARTESIAN_POINT('',(-2.49901111423969,0.233356082439423,5.37));
#44190=CARTESIAN_POINT('',(-2.49901111423969,0.233356082439423,5.4));
#44191=CARTESIAN_POINT('Ctrl Pts',(-2.49901111423969,0.233356082439423,
5.37));
#44192=CARTESIAN_POINT('Ctrl Pts',(-2.48963184654713,0.263369733095169,
5.37));
#44193=CARTESIAN_POINT('Ctrl Pts',(-2.4697477966547,0.321521157026291,5.37));
#44194=CARTESIAN_POINT('Ctrl Pts',(-2.52527303993702,0.31476808488369,5.4));
#44195=CARTESIAN_POINT('Ctrl Pts',(-2.52527303993702,0.31476808488369,5.37));
#44196=CARTESIAN_POINT('Ctrl Pts',(-2.50726486742496,0.260368371009827,
5.4));
#44197=CARTESIAN_POINT('Ctrl Pts',(-2.50726486742496,0.260368371009827,
5.37));
#44198=CARTESIAN_POINT('Ctrl Pts',(-2.49901111423969,0.233356082439423,
5.4));
#44199=CARTESIAN_POINT('Ctrl Pts',(-2.49901111423969,0.233356082439423,
5.37));
#44200=CARTESIAN_POINT('',(-2.52527303993702,0.31476808488369,5.4));
#44201=CARTESIAN_POINT('Ctrl Pts',(-2.52527303993702,0.31476808488369,5.4));
#44202=CARTESIAN_POINT('Ctrl Pts',(-2.50726486742496,0.260368371009827,
5.4));
#44203=CARTESIAN_POINT('Ctrl Pts',(-2.49901111423969,0.233356082439423,
5.4));
#44204=CARTESIAN_POINT('',(-2.52527303993702,0.31476808488369,5.37));
#44205=CARTESIAN_POINT('',(-2.52527303993702,0.31476808488369,5.4));
#44206=CARTESIAN_POINT('Ctrl Pts',(-2.52527303993702,0.31476808488369,5.37));
#44207=CARTESIAN_POINT('Ctrl Pts',(-2.50726486742496,0.260368371009827,
5.37));
#44208=CARTESIAN_POINT('Ctrl Pts',(-2.49901111423969,0.233356082439423,
5.37));
#44209=CARTESIAN_POINT('Origin',(-2.655457213521,0.704195106029511,5.4));
#44210=CARTESIAN_POINT('',(-2.655457213521,0.704195106029511,5.4));
#44211=CARTESIAN_POINT('',(-2.41611977305377,-0.0117480376252982,5.4));
#44212=CARTESIAN_POINT('',(-2.655457213521,0.704195106029511,5.37));
#44213=CARTESIAN_POINT('',(-2.655457213521,0.704195106029511,5.4));
#44214=CARTESIAN_POINT('',(-2.655457213521,0.704195106029511,5.37));
#44215=CARTESIAN_POINT('Origin',(-2.76500703394413,0.704195106029511,5.4));
#44216=CARTESIAN_POINT('',(-2.76500703394413,0.704195106029511,5.4));
#44217=CARTESIAN_POINT('',(-1.38250351697206,0.704195106029511,5.4));
#44218=CARTESIAN_POINT('',(-2.76500703394413,0.704195106029511,5.37));
#44219=CARTESIAN_POINT('',(-2.76500703394413,0.704195106029511,5.4));
#44220=CARTESIAN_POINT('',(-2.76500703394413,0.704195106029511,5.37));
#44221=CARTESIAN_POINT('Origin',(-2.76500703394413,0.154195094108582,5.4));
#44222=CARTESIAN_POINT('',(-2.76500703394413,0.154195094108582,5.4));
#44223=CARTESIAN_POINT('',(-2.76500703394413,0.0770975470542908,5.4));
#44224=CARTESIAN_POINT('',(-2.76500703394413,0.154195094108582,5.37));
#44225=CARTESIAN_POINT('',(-2.76500703394413,0.154195094108582,5.4));
#44226=CARTESIAN_POINT('',(-2.76500703394413,0.154195094108582,5.37));
#44227=CARTESIAN_POINT('Origin',(-2.69485013186932,0.154195094108582,5.4));
#44228=CARTESIAN_POINT('',(-2.69485013186932,0.154195094108582,5.4));
#44229=CARTESIAN_POINT('',(-1.34742506593466,0.154195094108582,5.4));
#44230=CARTESIAN_POINT('',(-2.69485013186932,0.154195094108582,5.37));
#44231=CARTESIAN_POINT('',(-2.69485013186932,0.154195094108582,5.4));
#44232=CARTESIAN_POINT('',(-2.69485013186932,0.154195094108582,5.37));
#44233=CARTESIAN_POINT('Origin',(-2.69485013186932,0.622407937049866,5.4));
#44234=CARTESIAN_POINT('',(-2.69485013186932,0.311203968524933,5.4));
#44235=CARTESIAN_POINT('',(-2.69485013186932,0.622407937049866,5.37));
#44236=CARTESIAN_POINT('Origin',(-2.50257523357868,0.429195100069046,5.37));
#44237=CARTESIAN_POINT('Ctrl Pts',(-0.133935943245888,0.194525921344757,
5.4));
#44238=CARTESIAN_POINT('Ctrl Pts',(-0.133935943245888,0.194525921344757,
5.37));
#44239=CARTESIAN_POINT('Ctrl Pts',(-0.186459794640541,0.144440674781799,
5.4));
#44240=CARTESIAN_POINT('Ctrl Pts',(-0.186459794640541,0.144440674781799,
5.37));
#44241=CARTESIAN_POINT('Ctrl Pts',(-0.266746297478676,0.144440674781799,
5.4));
#44242=CARTESIAN_POINT('Ctrl Pts',(-0.266746297478676,0.144440674781799,
5.37));
#44243=CARTESIAN_POINT('',(-0.133935943245888,0.194525921344757,5.4));
#44244=CARTESIAN_POINT('',(-0.266746297478676,0.144440674781799,5.4));
#44245=CARTESIAN_POINT('Ctrl Pts',(-0.133935943245888,0.194525921344757,
5.4));
#44246=CARTESIAN_POINT('Ctrl Pts',(-0.186459794640541,0.144440674781799,
5.4));
#44247=CARTESIAN_POINT('Ctrl Pts',(-0.266746297478676,0.144440674781799,
5.4));
#44248=CARTESIAN_POINT('',(-0.133935943245888,0.194525921344757,5.37));
#44249=CARTESIAN_POINT('',(-0.133935943245888,0.194525921344757,5.4));
#44250=CARTESIAN_POINT('',(-0.266746297478676,0.144440674781799,5.37));
#44251=CARTESIAN_POINT('Ctrl Pts',(-0.133935943245888,0.194525921344757,
5.37));
#44252=CARTESIAN_POINT('Ctrl Pts',(-0.186459794640541,0.144440674781799,
5.37));
#44253=CARTESIAN_POINT('Ctrl Pts',(-0.266746297478676,0.144440674781799,
5.37));
#44254=CARTESIAN_POINT('',(-0.266746297478676,0.144440674781799,5.4));
#44255=CARTESIAN_POINT('Ctrl Pts',(-0.0814120918512344,0.316643932461739,
5.4));
#44256=CARTESIAN_POINT('Ctrl Pts',(-0.0814120918512344,0.316643932461739,
5.37));
#44257=CARTESIAN_POINT('Ctrl Pts',(-0.0814120918512344,0.244611197710037,
5.4));
#44258=CARTESIAN_POINT('Ctrl Pts',(-0.0814120918512344,0.244611197710037,
5.37));
#44259=CARTESIAN_POINT('Ctrl Pts',(-0.133935943245888,0.194525921344757,
5.4));
#44260=CARTESIAN_POINT('Ctrl Pts',(-0.133935943245888,0.194525921344757,
5.37));
#44261=CARTESIAN_POINT('',(-0.0814120918512344,0.316643932461739,5.4));
#44262=CARTESIAN_POINT('Ctrl Pts',(-0.0814120918512344,0.316643932461739,
5.4));
#44263=CARTESIAN_POINT('Ctrl Pts',(-0.0814120918512344,0.244611197710037,
5.4));
#44264=CARTESIAN_POINT('Ctrl Pts',(-0.133935943245888,0.194525921344757,
5.4));
#44265=CARTESIAN_POINT('',(-0.0814120918512344,0.316643932461739,5.37));
#44266=CARTESIAN_POINT('',(-0.0814120918512344,0.316643932461739,5.4));
#44267=CARTESIAN_POINT('Ctrl Pts',(-0.0814120918512344,0.316643932461739,
5.37));
#44268=CARTESIAN_POINT('Ctrl Pts',(-0.0814120918512344,0.244611197710037,
5.37));
#44269=CARTESIAN_POINT('Ctrl Pts',(-0.133935943245888,0.194525921344757,
5.37));
#44270=CARTESIAN_POINT('Ctrl Pts',(-0.108424201607704,0.405371749401093,
5.4));
#44271=CARTESIAN_POINT('Ctrl Pts',(-0.108424201607704,0.405371749401093,
5.37));
#44272=CARTESIAN_POINT('Ctrl Pts',(-0.0814120918512344,0.369918146729469,
5.4));
#44273=CARTESIAN_POINT('Ctrl Pts',(-0.0814120918512344,0.369918146729469,
5.37));
#44274=CARTESIAN_POINT('Ctrl Pts',(-0.0814120918512344,0.316643932461739,
5.4));
#44275=CARTESIAN_POINT('Ctrl Pts',(-0.0814120918512344,0.316643932461739,
5.37));
#44276=CARTESIAN_POINT('',(-0.108424201607704,0.405371749401093,5.4));
#44277=CARTESIAN_POINT('Ctrl Pts',(-0.108424201607704,0.405371749401093,
5.4));
#44278=CARTESIAN_POINT('Ctrl Pts',(-0.0814120918512344,0.369918146729469,
5.4));
#44279=CARTESIAN_POINT('Ctrl Pts',(-0.0814120918512344,0.316643932461739,
5.4));
#44280=CARTESIAN_POINT('',(-0.108424201607704,0.405371749401093,5.37));
#44281=CARTESIAN_POINT('',(-0.108424201607704,0.405371749401093,5.4));
#44282=CARTESIAN_POINT('Ctrl Pts',(-0.108424201607704,0.405371749401093,
5.37));
#44283=CARTESIAN_POINT('Ctrl Pts',(-0.0814120918512344,0.369918146729469,
5.37));
#44284=CARTESIAN_POINT('Ctrl Pts',(-0.0814120918512344,0.316643932461739,
5.37));
#44285=CARTESIAN_POINT('Ctrl Pts',(-0.184208884835243,0.452080512046814,
5.4));
#44286=CARTESIAN_POINT('Ctrl Pts',(-0.184208884835243,0.452080512046814,
5.37));
#44287=CARTESIAN_POINT('Ctrl Pts',(-0.135436549782753,0.440825366973877,
5.4));
#44288=CARTESIAN_POINT('Ctrl Pts',(-0.135436549782753,0.440825366973877,
5.37));
#44289=CARTESIAN_POINT('Ctrl Pts',(-0.108424201607704,0.405371749401093,
5.4));
#44290=CARTESIAN_POINT('Ctrl Pts',(-0.108424201607704,0.405371749401093,
5.37));
#44291=CARTESIAN_POINT('',(-0.184208884835243,0.452080512046814,5.4));
#44292=CARTESIAN_POINT('Ctrl Pts',(-0.184208884835243,0.452080512046814,
5.4));
#44293=CARTESIAN_POINT('Ctrl Pts',(-0.135436549782753,0.440825366973877,
5.4));
#44294=CARTESIAN_POINT('Ctrl Pts',(-0.108424201607704,0.405371749401093,
5.4));
#44295=CARTESIAN_POINT('',(-0.184208884835243,0.452080512046814,5.37));
#44296=CARTESIAN_POINT('',(-0.184208884835243,0.452080512046814,5.4));
#44297=CARTESIAN_POINT('Ctrl Pts',(-0.184208884835243,0.452080512046814,
5.37));
#44298=CARTESIAN_POINT('Ctrl Pts',(-0.135436549782753,0.440825366973877,
5.37));
#44299=CARTESIAN_POINT('Ctrl Pts',(-0.108424201607704,0.405371749401093,
5.37));
#44300=CARTESIAN_POINT('Ctrl Pts',(-0.127558007836342,0.498601639270782,
5.4));
#44301=CARTESIAN_POINT('Ctrl Pts',(-0.127558007836342,0.498601639270782,
5.37));
#44302=CARTESIAN_POINT('Ctrl Pts',(-0.14669181406498,0.469338321685791,
5.4));
#44303=CARTESIAN_POINT('Ctrl Pts',(-0.14669181406498,0.469338321685791,
5.37));
#44304=CARTESIAN_POINT('Ctrl Pts',(-0.184208884835243,0.452080512046814,
5.4));
#44305=CARTESIAN_POINT('Ctrl Pts',(-0.184208884835243,0.452080512046814,
5.37));
#44306=CARTESIAN_POINT('',(-0.127558007836342,0.498601639270782,5.4));
#44307=CARTESIAN_POINT('Ctrl Pts',(-0.127558007836342,0.498601639270782,
5.4));
#44308=CARTESIAN_POINT('Ctrl Pts',(-0.14669181406498,0.469338321685791,
5.4));
#44309=CARTESIAN_POINT('Ctrl Pts',(-0.184208884835243,0.452080512046814,
5.4));
#44310=CARTESIAN_POINT('',(-0.127558007836342,0.498601639270782,5.37));
#44311=CARTESIAN_POINT('',(-0.127558007836342,0.498601639270782,5.4));
#44312=CARTESIAN_POINT('Ctrl Pts',(-0.127558007836342,0.498601639270782,
5.37));
#44313=CARTESIAN_POINT('Ctrl Pts',(-0.14669181406498,0.469338321685791,
5.37));
#44314=CARTESIAN_POINT('Ctrl Pts',(-0.184208884835243,0.452080512046814,
5.37));
#44315=CARTESIAN_POINT('Ctrl Pts',(-0.108424201607704,0.563506150245667,
5.4));
#44316=CARTESIAN_POINT('Ctrl Pts',(-0.108424201607704,0.563506150245667,
5.37));
#44317=CARTESIAN_POINT('Ctrl Pts',(-0.108424201607704,0.527864956855774,
5.4));
#44318=CARTESIAN_POINT('Ctrl Pts',(-0.108424201607704,0.527864956855774,
5.37));
#44319=CARTESIAN_POINT('Ctrl Pts',(-0.127558007836342,0.498601639270782,
5.4));
#44320=CARTESIAN_POINT('Ctrl Pts',(-0.127558007836342,0.498601639270782,
5.37));
#44321=CARTESIAN_POINT('',(-0.108424201607704,0.563506150245667,5.4));
#44322=CARTESIAN_POINT('Ctrl Pts',(-0.108424201607704,0.563506150245667,
5.4));
#44323=CARTESIAN_POINT('Ctrl Pts',(-0.108424201607704,0.527864956855774,
5.4));
#44324=CARTESIAN_POINT('Ctrl Pts',(-0.127558007836342,0.498601639270782,
5.4));
#44325=CARTESIAN_POINT('',(-0.108424201607704,0.563506150245667,5.37));
#44326=CARTESIAN_POINT('',(-0.108424201607704,0.563506150245667,5.4));
#44327=CARTESIAN_POINT('Ctrl Pts',(-0.108424201607704,0.563506150245667,
5.37));
#44328=CARTESIAN_POINT('Ctrl Pts',(-0.108424201607704,0.527864956855774,
5.37));
#44329=CARTESIAN_POINT('Ctrl Pts',(-0.127558007836342,0.498601639270782,
5.37));
#44330=CARTESIAN_POINT('Ctrl Pts',(-0.128495946526527,0.634413385391235,
5.4));
#44331=CARTESIAN_POINT('Ctrl Pts',(-0.128495946526527,0.634413385391235,
5.37));
#44332=CARTESIAN_POINT('Ctrl Pts',(-0.108424201607704,0.601023161411285,
5.4));
#44333=CARTESIAN_POINT('Ctrl Pts',(-0.108424201607704,0.601023161411285,
5.37));
#44334=CARTESIAN_POINT('Ctrl Pts',(-0.108424201607704,0.563506150245667,
5.4));
#44335=CARTESIAN_POINT('Ctrl Pts',(-0.108424201607704,0.563506150245667,
5.37));
#44336=CARTESIAN_POINT('',(-0.128495946526527,0.634413385391235,5.4));
#44337=CARTESIAN_POINT('Ctrl Pts',(-0.128495946526527,0.634413385391235,
5.4));
#44338=CARTESIAN_POINT('Ctrl Pts',(-0.108424201607704,0.601023161411285,
5.4));
#44339=CARTESIAN_POINT('Ctrl Pts',(-0.108424201607704,0.563506150245667,
5.4));
#44340=CARTESIAN_POINT('',(-0.128495946526527,0.634413385391235,5.37));
#44341=CARTESIAN_POINT('',(-0.128495946526527,0.634413385391235,5.4));
#44342=CARTESIAN_POINT('Ctrl Pts',(-0.128495946526527,0.634413385391235,
5.37));
#44343=CARTESIAN_POINT('Ctrl Pts',(-0.108424201607704,0.601023161411285,
5.37));
#44344=CARTESIAN_POINT('Ctrl Pts',(-0.108424201607704,0.563506150245667,
5.37));
#44345=CARTESIAN_POINT('Ctrl Pts',(-0.186459794640541,0.687124812602997,
5.4));
#44346=CARTESIAN_POINT('Ctrl Pts',(-0.186459794640541,0.687124812602997,
5.37));
#44347=CARTESIAN_POINT('Ctrl Pts',(-0.148567691445351,0.667803549766541,
5.4));
#44348=CARTESIAN_POINT('Ctrl Pts',(-0.148567691445351,0.667803549766541,
5.37));
#44349=CARTESIAN_POINT('Ctrl Pts',(-0.128495946526527,0.634413385391235,
5.4));
#44350=CARTESIAN_POINT('Ctrl Pts',(-0.128495946526527,0.634413385391235,
5.37));
#44351=CARTESIAN_POINT('',(-0.186459794640541,0.687124812602997,5.4));
#44352=CARTESIAN_POINT('Ctrl Pts',(-0.186459794640541,0.687124812602997,
5.4));
#44353=CARTESIAN_POINT('Ctrl Pts',(-0.148567691445351,0.667803549766541,
5.4));
#44354=CARTESIAN_POINT('Ctrl Pts',(-0.128495946526527,0.634413385391235,
5.4));
#44355=CARTESIAN_POINT('',(-0.186459794640541,0.687124812602997,5.37));
#44356=CARTESIAN_POINT('',(-0.186459794640541,0.687124812602997,5.4));
#44357=CARTESIAN_POINT('Ctrl Pts',(-0.186459794640541,0.687124812602997,
5.37));
#44358=CARTESIAN_POINT('Ctrl Pts',(-0.148567691445351,0.667803549766541,
5.37));
#44359=CARTESIAN_POINT('Ctrl Pts',(-0.128495946526527,0.634413385391235,
5.37));
#44360=CARTESIAN_POINT('Ctrl Pts',(-0.26937247812748,0.706446135044098,
5.4));
#44361=CARTESIAN_POINT('Ctrl Pts',(-0.26937247812748,0.706446135044098,
5.37));
#44362=CARTESIAN_POINT('Ctrl Pts',(-0.224352136254311,0.706446135044098,
5.4));
#44363=CARTESIAN_POINT('Ctrl Pts',(-0.224352136254311,0.706446135044098,
5.37));
#44364=CARTESIAN_POINT('Ctrl Pts',(-0.186459794640541,0.687124812602997,
5.4));
#44365=CARTESIAN_POINT('Ctrl Pts',(-0.186459794640541,0.687124812602997,
5.37));
#44366=CARTESIAN_POINT('',(-0.26937247812748,0.706446135044098,5.4));
#44367=CARTESIAN_POINT('Ctrl Pts',(-0.26937247812748,0.706446135044098,
5.4));
#44368=CARTESIAN_POINT('Ctrl Pts',(-0.224352136254311,0.706446135044098,
5.4));
#44369=CARTESIAN_POINT('Ctrl Pts',(-0.186459794640541,0.687124812602997,
5.4));
#44370=CARTESIAN_POINT('',(-0.26937247812748,0.706446135044098,5.37));
#44371=CARTESIAN_POINT('',(-0.26937247812748,0.706446135044098,5.4));
#44372=CARTESIAN_POINT('Ctrl Pts',(-0.26937247812748,0.706446135044098,
5.37));
#44373=CARTESIAN_POINT('Ctrl Pts',(-0.224352136254311,0.706446135044098,
5.37));
#44374=CARTESIAN_POINT('Ctrl Pts',(-0.186459794640541,0.687124812602997,
5.37));
#44375=CARTESIAN_POINT('Ctrl Pts',(-0.378547206521034,0.669116640090942,
5.4));
#44376=CARTESIAN_POINT('Ctrl Pts',(-0.378547206521034,0.669116640090942,
5.37));
#44377=CARTESIAN_POINT('Ctrl Pts',(-0.334652200341225,0.706446135044098,
5.4));
#44378=CARTESIAN_POINT('Ctrl Pts',(-0.334652200341225,0.706446135044098,
5.37));
#44379=CARTESIAN_POINT('Ctrl Pts',(-0.26937247812748,0.706446135044098,
5.4));
#44380=CARTESIAN_POINT('Ctrl Pts',(-0.26937247812748,0.706446135044098,
5.37));
#44381=CARTESIAN_POINT('',(-0.378547206521034,0.669116640090942,5.4));
#44382=CARTESIAN_POINT('Ctrl Pts',(-0.378547206521034,0.669116640090942,
5.4));
#44383=CARTESIAN_POINT('Ctrl Pts',(-0.334652200341225,0.706446135044098,
5.4));
#44384=CARTESIAN_POINT('Ctrl Pts',(-0.26937247812748,0.706446135044098,
5.4));
#44385=CARTESIAN_POINT('',(-0.378547206521034,0.669116640090942,5.37));
#44386=CARTESIAN_POINT('',(-0.378547206521034,0.669116640090942,5.4));
#44387=CARTESIAN_POINT('Ctrl Pts',(-0.378547206521034,0.669116640090942,
5.37));
#44388=CARTESIAN_POINT('Ctrl Pts',(-0.334652200341225,0.706446135044098,
5.37));
#44389=CARTESIAN_POINT('Ctrl Pts',(-0.26937247812748,0.706446135044098,
5.37));
#44390=CARTESIAN_POINT('Ctrl Pts',(-0.43482281267643,0.563881301879883,
5.4));
#44391=CARTESIAN_POINT('Ctrl Pts',(-0.43482281267643,0.563881301879883,
5.37));
#44392=CARTESIAN_POINT('Ctrl Pts',(-0.422441974282265,0.631787145137787,
5.4));
#44393=CARTESIAN_POINT('Ctrl Pts',(-0.422441974282265,0.631787145137787,
5.37));
#44394=CARTESIAN_POINT('Ctrl Pts',(-0.378547206521034,0.669116640090942,
5.4));
#44395=CARTESIAN_POINT('Ctrl Pts',(-0.378547206521034,0.669116640090942,
5.37));
#44396=CARTESIAN_POINT('',(-0.43482281267643,0.563881301879883,5.4));
#44397=CARTESIAN_POINT('Ctrl Pts',(-0.43482281267643,0.563881301879883,
5.4));
#44398=CARTESIAN_POINT('Ctrl Pts',(-0.422441974282265,0.631787145137787,
5.4));
#44399=CARTESIAN_POINT('Ctrl Pts',(-0.378547206521034,0.669116640090942,
5.4));
#44400=CARTESIAN_POINT('',(-0.43482281267643,0.563881301879883,5.37));
#44401=CARTESIAN_POINT('',(-0.43482281267643,0.563881301879883,5.4));
#44402=CARTESIAN_POINT('Ctrl Pts',(-0.43482281267643,0.563881301879883,
5.37));
#44403=CARTESIAN_POINT('Ctrl Pts',(-0.422441974282265,0.631787145137787,
5.37));
#44404=CARTESIAN_POINT('Ctrl Pts',(-0.378547206521034,0.669116640090942,
5.37));
#44405=CARTESIAN_POINT('Origin',(-0.367291942238808,0.551875853538513,5.4));
#44406=CARTESIAN_POINT('',(-0.367291942238808,0.551875853538513,5.4));
#44407=CARTESIAN_POINT('',(-0.141719653140393,0.511774245985313,5.4));
#44408=CARTESIAN_POINT('',(-0.367291942238808,0.551875853538513,5.37));
#44409=CARTESIAN_POINT('',(-0.367291942238808,0.551875853538513,5.4));
#44410=CARTESIAN_POINT('',(-0.367291942238808,0.551875853538513,5.37));
#44411=CARTESIAN_POINT('Ctrl Pts',(-0.333526626229286,0.626159632205963,
5.4));
#44412=CARTESIAN_POINT('Ctrl Pts',(-0.333526626229286,0.626159632205963,
5.37));
#44413=CARTESIAN_POINT('Ctrl Pts',(-0.359788671135902,0.601398372650147,
5.4));
#44414=CARTESIAN_POINT('Ctrl Pts',(-0.359788671135902,0.601398372650147,
5.37));
#44415=CARTESIAN_POINT('Ctrl Pts',(-0.367291942238808,0.551875853538513,
5.4));
#44416=CARTESIAN_POINT('Ctrl Pts',(-0.367291942238808,0.551875853538513,
5.37));
#44417=CARTESIAN_POINT('',(-0.333526626229286,0.626159632205963,5.4));
#44418=CARTESIAN_POINT('Ctrl Pts',(-0.333526626229286,0.626159632205963,
5.4));
#44419=CARTESIAN_POINT('Ctrl Pts',(-0.359788671135902,0.601398372650147,
5.4));
#44420=CARTESIAN_POINT('Ctrl Pts',(-0.367291942238808,0.551875853538513,
5.4));
#44421=CARTESIAN_POINT('',(-0.333526626229286,0.626159632205963,5.37));
#44422=CARTESIAN_POINT('',(-0.333526626229286,0.626159632205963,5.4));
#44423=CARTESIAN_POINT('Ctrl Pts',(-0.333526626229286,0.626159632205963,
5.37));
#44424=CARTESIAN_POINT('Ctrl Pts',(-0.359788671135902,0.601398372650147,
5.37));
#44425=CARTESIAN_POINT('Ctrl Pts',(-0.367291942238808,0.551875853538513,
5.37));
#44426=CARTESIAN_POINT('Ctrl Pts',(-0.267871871590614,0.65092089176178,
5.4));
#44427=CARTESIAN_POINT('Ctrl Pts',(-0.267871871590614,0.65092089176178,
5.37));
#44428=CARTESIAN_POINT('Ctrl Pts',(-0.307264819741249,0.65092089176178,
5.4));
#44429=CARTESIAN_POINT('Ctrl Pts',(-0.307264819741249,0.65092089176178,
5.37));
#44430=CARTESIAN_POINT('Ctrl Pts',(-0.333526626229286,0.626159632205963,
5.4));
#44431=CARTESIAN_POINT('Ctrl Pts',(-0.333526626229286,0.626159632205963,
5.37));
#44432=CARTESIAN_POINT('',(-0.267871871590614,0.65092089176178,5.4));
#44433=CARTESIAN_POINT('Ctrl Pts',(-0.267871871590614,0.65092089176178,
5.4));
#44434=CARTESIAN_POINT('Ctrl Pts',(-0.307264819741249,0.65092089176178,
5.4));
#44435=CARTESIAN_POINT('Ctrl Pts',(-0.333526626229286,0.626159632205963,
5.4));
#44436=CARTESIAN_POINT('',(-0.267871871590614,0.65092089176178,5.37));
#44437=CARTESIAN_POINT('',(-0.267871871590614,0.65092089176178,5.4));
#44438=CARTESIAN_POINT('Ctrl Pts',(-0.267871871590614,0.65092089176178,
5.37));
#44439=CARTESIAN_POINT('Ctrl Pts',(-0.307264819741249,0.65092089176178,
5.37));
#44440=CARTESIAN_POINT('Ctrl Pts',(-0.333526626229286,0.626159632205963,
5.37));
#44441=CARTESIAN_POINT('Ctrl Pts',(-0.202967420220375,0.626534783840179,
5.4));
#44442=CARTESIAN_POINT('Ctrl Pts',(-0.202967420220375,0.626534783840179,
5.37));
#44443=CARTESIAN_POINT('Ctrl Pts',(-0.228103652596474,0.65092089176178,
5.4));
#44444=CARTESIAN_POINT('Ctrl Pts',(-0.228103652596474,0.65092089176178,
5.37));
#44445=CARTESIAN_POINT('Ctrl Pts',(-0.267871871590614,0.65092089176178,
5.4));
#44446=CARTESIAN_POINT('Ctrl Pts',(-0.267871871590614,0.65092089176178,
5.37));
#44447=CARTESIAN_POINT('',(-0.202967420220375,0.626534783840179,5.4));
#44448=CARTESIAN_POINT('Ctrl Pts',(-0.202967420220375,0.626534783840179,
5.4));
#44449=CARTESIAN_POINT('Ctrl Pts',(-0.228103652596474,0.65092089176178,
5.4));
#44450=CARTESIAN_POINT('Ctrl Pts',(-0.267871871590614,0.65092089176178,
5.4));
#44451=CARTESIAN_POINT('',(-0.202967420220375,0.626534783840179,5.37));
#44452=CARTESIAN_POINT('',(-0.202967420220375,0.626534783840179,5.4));
#44453=CARTESIAN_POINT('Ctrl Pts',(-0.202967420220375,0.626534783840179,
5.37));
#44454=CARTESIAN_POINT('Ctrl Pts',(-0.228103652596474,0.65092089176178,
5.37));
#44455=CARTESIAN_POINT('Ctrl Pts',(-0.267871871590614,0.65092089176178,
5.37));
#44456=CARTESIAN_POINT('Ctrl Pts',(-0.177830949425697,0.565006816387177,
5.4));
#44457=CARTESIAN_POINT('Ctrl Pts',(-0.177830949425697,0.565006816387177,
5.37));
#44458=CARTESIAN_POINT('Ctrl Pts',(-0.177830949425697,0.602148675918579,
5.4));
#44459=CARTESIAN_POINT('Ctrl Pts',(-0.177830949425697,0.602148675918579,
5.37));
#44460=CARTESIAN_POINT('Ctrl Pts',(-0.202967420220375,0.626534783840179,
5.4));
#44461=CARTESIAN_POINT('Ctrl Pts',(-0.202967420220375,0.626534783840179,
5.37));
#44462=CARTESIAN_POINT('',(-0.177830949425697,0.565006816387177,5.4));
#44463=CARTESIAN_POINT('Ctrl Pts',(-0.177830949425697,0.565006816387177,
5.4));
#44464=CARTESIAN_POINT('Ctrl Pts',(-0.177830949425697,0.602148675918579,
5.4));
#44465=CARTESIAN_POINT('Ctrl Pts',(-0.202967420220375,0.626534783840179,
5.4));
#44466=CARTESIAN_POINT('',(-0.177830949425697,0.565006816387177,5.37));
#44467=CARTESIAN_POINT('',(-0.177830949425697,0.565006816387177,5.4));
#44468=CARTESIAN_POINT('Ctrl Pts',(-0.177830949425697,0.565006816387177,
5.37));
#44469=CARTESIAN_POINT('Ctrl Pts',(-0.177830949425697,0.602148675918579,
5.37));
#44470=CARTESIAN_POINT('Ctrl Pts',(-0.202967420220375,0.626534783840179,
5.37));
#44471=CARTESIAN_POINT('Ctrl Pts',(-0.212346568703651,0.495600247383118,
5.4));
#44472=CARTESIAN_POINT('Ctrl Pts',(-0.212346568703651,0.495600247383118,
5.37));
#44473=CARTESIAN_POINT('Ctrl Pts',(-0.177830949425697,0.518110477924347,
5.4));
#44474=CARTESIAN_POINT('Ctrl Pts',(-0.177830949425697,0.518110477924347,
5.37));
#44475=CARTESIAN_POINT('Ctrl Pts',(-0.177830949425697,0.565006816387177,
5.4));
#44476=CARTESIAN_POINT('Ctrl Pts',(-0.177830949425697,0.565006816387177,
5.37));
#44477=CARTESIAN_POINT('',(-0.212346568703651,0.495600247383118,5.4));
#44478=CARTESIAN_POINT('Ctrl Pts',(-0.212346568703651,0.495600247383118,
5.4));
#44479=CARTESIAN_POINT('Ctrl Pts',(-0.177830949425697,0.518110477924347,
5.4));
#44480=CARTESIAN_POINT('Ctrl Pts',(-0.177830949425697,0.565006816387177,
5.4));
#44481=CARTESIAN_POINT('',(-0.212346568703651,0.495600247383118,5.37));
#44482=CARTESIAN_POINT('',(-0.212346568703651,0.495600247383118,5.4));
#44483=CARTESIAN_POINT('Ctrl Pts',(-0.212346568703651,0.495600247383118,
5.37));
#44484=CARTESIAN_POINT('Ctrl Pts',(-0.177830949425697,0.518110477924347,
5.37));
#44485=CARTESIAN_POINT('Ctrl Pts',(-0.177830949425697,0.565006816387177,
5.37));
#44486=CARTESIAN_POINT('Ctrl Pts',(-0.290006890892982,0.473090016841888,
5.4));
#44487=CARTESIAN_POINT('Ctrl Pts',(-0.290006890892982,0.473090016841888,
5.37));
#44488=CARTESIAN_POINT('Ctrl Pts',(-0.246862187981606,0.473090016841888,
5.4));
#44489=CARTESIAN_POINT('Ctrl Pts',(-0.246862187981606,0.473090016841888,
5.37));
#44490=CARTESIAN_POINT('Ctrl Pts',(-0.212346568703651,0.495600247383118,
5.4));
#44491=CARTESIAN_POINT('Ctrl Pts',(-0.212346568703651,0.495600247383118,
5.37));
#44492=CARTESIAN_POINT('',(-0.290006890892982,0.473090016841888,5.4));
#44493=CARTESIAN_POINT('Ctrl Pts',(-0.290006890892982,0.473090016841888,
5.4));
#44494=CARTESIAN_POINT('Ctrl Pts',(-0.246862187981606,0.473090016841888,
5.4));
#44495=CARTESIAN_POINT('Ctrl Pts',(-0.212346568703651,0.495600247383118,
5.4));
#44496=CARTESIAN_POINT('',(-0.290006890892982,0.473090016841888,5.37));
#44497=CARTESIAN_POINT('',(-0.290006890892982,0.473090016841888,5.4));
#44498=CARTESIAN_POINT('Ctrl Pts',(-0.290006890892982,0.473090016841888,
5.37));
#44499=CARTESIAN_POINT('Ctrl Pts',(-0.246862187981606,0.473090016841888,
5.37));
#44500=CARTESIAN_POINT('Ctrl Pts',(-0.212346568703651,0.495600247383118,
5.37));
#44501=CARTESIAN_POINT('Ctrl Pts',(-0.300886884331703,0.473840379714966,
5.4));
#44502=CARTESIAN_POINT('Ctrl Pts',(-0.300886884331703,0.473840379714966,
5.37));
#44503=CARTESIAN_POINT('Ctrl Pts',(-0.294133678078651,0.473090016841888,
5.4));
#44504=CARTESIAN_POINT('Ctrl Pts',(-0.294133678078651,0.473090016841888,
5.37));
#44505=CARTESIAN_POINT('Ctrl Pts',(-0.290006890892982,0.473090016841888,
5.4));
#44506=CARTESIAN_POINT('Ctrl Pts',(-0.290006890892982,0.473090016841888,
5.37));
#44507=CARTESIAN_POINT('',(-0.300886884331703,0.473840379714966,5.4));
#44508=CARTESIAN_POINT('Ctrl Pts',(-0.300886884331703,0.473840379714966,
5.4));
#44509=CARTESIAN_POINT('Ctrl Pts',(-0.294133678078651,0.473090016841888,
5.4));
#44510=CARTESIAN_POINT('Ctrl Pts',(-0.290006890892982,0.473090016841888,
5.4));
#44511=CARTESIAN_POINT('',(-0.300886884331703,0.473840379714966,5.37));
#44512=CARTESIAN_POINT('',(-0.300886884331703,0.473840379714966,5.4));
#44513=CARTESIAN_POINT('Ctrl Pts',(-0.300886884331703,0.473840379714966,
5.37));
#44514=CARTESIAN_POINT('Ctrl Pts',(-0.294133678078651,0.473090016841888,
5.37));
#44515=CARTESIAN_POINT('Ctrl Pts',(-0.290006890892982,0.473090016841888,
5.37));
#44516=CARTESIAN_POINT('Origin',(-0.308390155434609,0.41456344127655,5.4));
#44517=CARTESIAN_POINT('',(-0.308390155434609,0.41456344127655,5.4));
#44518=CARTESIAN_POINT('',(-0.331782471939349,0.229760721720473,5.4));
#44519=CARTESIAN_POINT('',(-0.308390155434609,0.41456344127655,5.37));
#44520=CARTESIAN_POINT('',(-0.308390155434609,0.41456344127655,5.4));
#44521=CARTESIAN_POINT('',(-0.308390155434609,0.41456344127655,5.37));
#44522=CARTESIAN_POINT('Ctrl Pts',(-0.260743632912636,0.422066831588745,
5.4));
#44523=CARTESIAN_POINT('Ctrl Pts',(-0.260743632912636,0.422066831588745,
5.37));
#44524=CARTESIAN_POINT('Ctrl Pts',(-0.279877200722694,0.422066831588745,
5.4));
#44525=CARTESIAN_POINT('Ctrl Pts',(-0.279877200722694,0.422066831588745,
5.37));
#44526=CARTESIAN_POINT('Ctrl Pts',(-0.308390155434608,0.41456344127655,
5.4));
#44527=CARTESIAN_POINT('Ctrl Pts',(-0.308390155434608,0.41456344127655,
5.37));
#44528=CARTESIAN_POINT('',(-0.260743632912636,0.422066831588745,5.4));
#44529=CARTESIAN_POINT('Ctrl Pts',(-0.260743632912636,0.422066831588745,
5.4));
#44530=CARTESIAN_POINT('Ctrl Pts',(-0.279877200722694,0.422066831588745,
5.4));
#44531=CARTESIAN_POINT('Ctrl Pts',(-0.308390155434608,0.41456344127655,
5.4));
#44532=CARTESIAN_POINT('',(-0.260743632912636,0.422066831588745,5.37));
#44533=CARTESIAN_POINT('',(-0.260743632912636,0.422066831588745,5.4));
#44534=CARTESIAN_POINT('Ctrl Pts',(-0.260743632912636,0.422066831588745,
5.37));
#44535=CARTESIAN_POINT('Ctrl Pts',(-0.279877200722694,0.422066831588745,
5.37));
#44536=CARTESIAN_POINT('Ctrl Pts',(-0.308390155434608,0.41456344127655,
5.37));
#44537=CARTESIAN_POINT('Ctrl Pts',(-0.183458343148232,0.391865620017052,
5.4));
#44538=CARTESIAN_POINT('Ctrl Pts',(-0.183458343148232,0.391865620017052,
5.37));
#44539=CARTESIAN_POINT('Ctrl Pts',(-0.213847175240517,0.422066831588745,
5.4));
#44540=CARTESIAN_POINT('Ctrl Pts',(-0.213847175240517,0.422066831588745,
5.37));
#44541=CARTESIAN_POINT('Ctrl Pts',(-0.260743632912636,0.422066831588745,
5.4));
#44542=CARTESIAN_POINT('Ctrl Pts',(-0.260743632912636,0.422066831588745,
5.37));
#44543=CARTESIAN_POINT('',(-0.183458343148232,0.391865620017052,5.4));
#44544=CARTESIAN_POINT('Ctrl Pts',(-0.183458343148232,0.391865620017052,
5.4));
#44545=CARTESIAN_POINT('Ctrl Pts',(-0.213847175240517,0.422066831588745,
5.4));
#44546=CARTESIAN_POINT('Ctrl Pts',(-0.260743632912636,0.422066831588745,
5.4));
#44547=CARTESIAN_POINT('',(-0.183458343148232,0.391865620017052,5.37));
#44548=CARTESIAN_POINT('',(-0.183458343148232,0.391865620017052,5.4));
#44549=CARTESIAN_POINT('Ctrl Pts',(-0.183458343148232,0.391865620017052,
5.37));
#44550=CARTESIAN_POINT('Ctrl Pts',(-0.213847175240517,0.422066831588745,
5.37));
#44551=CARTESIAN_POINT('Ctrl Pts',(-0.260743632912636,0.422066831588745,
5.37));
#44552=CARTESIAN_POINT('Ctrl Pts',(-0.153069511055946,0.315143251419067,
5.4));
#44553=CARTESIAN_POINT('Ctrl Pts',(-0.153069511055946,0.315143251419067,
5.37));
#44554=CARTESIAN_POINT('Ctrl Pts',(-0.153069511055946,0.361664393544197,
5.4));
#44555=CARTESIAN_POINT('Ctrl Pts',(-0.153069511055946,0.361664393544197,
5.37));
#44556=CARTESIAN_POINT('Ctrl Pts',(-0.183458343148232,0.391865620017052,
5.4));
#44557=CARTESIAN_POINT('Ctrl Pts',(-0.183458343148232,0.391865620017052,
5.37));
#44558=CARTESIAN_POINT('',(-0.153069511055946,0.315143251419067,5.4));
#44559=CARTESIAN_POINT('Ctrl Pts',(-0.153069511055946,0.315143251419067,
5.4));
#44560=CARTESIAN_POINT('Ctrl Pts',(-0.153069511055946,0.361664393544197,
5.4));
#44561=CARTESIAN_POINT('Ctrl Pts',(-0.183458343148232,0.391865620017052,
5.4));
#44562=CARTESIAN_POINT('',(-0.153069511055946,0.315143251419067,5.37));
#44563=CARTESIAN_POINT('',(-0.153069511055946,0.315143251419067,5.4));
#44564=CARTESIAN_POINT('Ctrl Pts',(-0.153069511055946,0.315143251419067,
5.37));
#44565=CARTESIAN_POINT('Ctrl Pts',(-0.153069511055946,0.361664393544197,
5.37));
#44566=CARTESIAN_POINT('Ctrl Pts',(-0.183458343148232,0.391865620017052,
5.37));
#44567=CARTESIAN_POINT('Ctrl Pts',(-0.185897126793861,0.233356082439423,
5.4));
#44568=CARTESIAN_POINT('Ctrl Pts',(-0.185897126793861,0.233356082439423,
5.37));
#44569=CARTESIAN_POINT('Ctrl Pts',(-0.153069511055946,0.266371095180511,
5.4));
#44570=CARTESIAN_POINT('Ctrl Pts',(-0.153069511055946,0.266371095180511,
5.37));
#44571=CARTESIAN_POINT('Ctrl Pts',(-0.153069511055946,0.315143251419067,
5.4));
#44572=CARTESIAN_POINT('Ctrl Pts',(-0.153069511055946,0.315143251419067,
5.37));
#44573=CARTESIAN_POINT('',(-0.185897126793861,0.233356082439423,5.4));
#44574=CARTESIAN_POINT('Ctrl Pts',(-0.185897126793861,0.233356082439423,
5.4));
#44575=CARTESIAN_POINT('Ctrl Pts',(-0.153069511055946,0.266371095180511,
5.4));
#44576=CARTESIAN_POINT('Ctrl Pts',(-0.153069511055946,0.315143251419067,
5.4));
#44577=CARTESIAN_POINT('',(-0.185897126793861,0.233356082439423,5.37));
#44578=CARTESIAN_POINT('',(-0.185897126793861,0.233356082439423,5.4));
#44579=CARTESIAN_POINT('Ctrl Pts',(-0.185897126793861,0.233356082439423,
5.37));
#44580=CARTESIAN_POINT('Ctrl Pts',(-0.153069511055946,0.266371095180511,
5.37));
#44581=CARTESIAN_POINT('Ctrl Pts',(-0.153069511055946,0.315143251419067,
5.37));
#44582=CARTESIAN_POINT('Ctrl Pts',(-0.26637102663517,0.200341069698334,
5.4));
#44583=CARTESIAN_POINT('Ctrl Pts',(-0.26637102663517,0.200341069698334,
5.37));
#44584=CARTESIAN_POINT('Ctrl Pts',(-0.218724504113197,0.200341069698334,
5.4));
#44585=CARTESIAN_POINT('Ctrl Pts',(-0.218724504113197,0.200341069698334,
5.37));
#44586=CARTESIAN_POINT('Ctrl Pts',(-0.185897126793861,0.233356082439423,
5.4));
#44587=CARTESIAN_POINT('Ctrl Pts',(-0.185897126793861,0.233356082439423,
5.37));
#44588=CARTESIAN_POINT('',(-0.26637102663517,0.200341069698334,5.4));
#44589=CARTESIAN_POINT('Ctrl Pts',(-0.26637102663517,0.200341069698334,
5.4));
#44590=CARTESIAN_POINT('Ctrl Pts',(-0.218724504113197,0.200341069698334,
5.4));
#44591=CARTESIAN_POINT('Ctrl Pts',(-0.185897126793861,0.233356082439423,
5.4));
#44592=CARTESIAN_POINT('',(-0.26637102663517,0.200341069698334,5.37));
#44593=CARTESIAN_POINT('',(-0.26637102663517,0.200341069698334,5.4));
#44594=CARTESIAN_POINT('Ctrl Pts',(-0.26637102663517,0.200341069698334,
5.37));
#44595=CARTESIAN_POINT('Ctrl Pts',(-0.218724504113197,0.200341069698334,
5.37));
#44596=CARTESIAN_POINT('Ctrl Pts',(-0.185897126793861,0.233356082439423,
5.37));
#44597=CARTESIAN_POINT('Ctrl Pts',(-0.334464564919472,0.225665086507797,
5.4));
#44598=CARTESIAN_POINT('Ctrl Pts',(-0.334464564919472,0.225665086507797,
5.37));
#44599=CARTESIAN_POINT('Ctrl Pts',(-0.306514278054237,0.200341069698334,
5.4));
#44600=CARTESIAN_POINT('Ctrl Pts',(-0.306514278054237,0.200341069698334,
5.37));
#44601=CARTESIAN_POINT('Ctrl Pts',(-0.26637102663517,0.200341069698334,
5.4));
#44602=CARTESIAN_POINT('Ctrl Pts',(-0.26637102663517,0.200341069698334,
5.37));
#44603=CARTESIAN_POINT('',(-0.334464564919472,0.225665086507797,5.4));
#44604=CARTESIAN_POINT('Ctrl Pts',(-0.334464564919472,0.225665086507797,
5.4));
#44605=CARTESIAN_POINT('Ctrl Pts',(-0.306514278054237,0.200341069698334,
5.4));
#44606=CARTESIAN_POINT('Ctrl Pts',(-0.26637102663517,0.200341069698334,
5.4));
#44607=CARTESIAN_POINT('',(-0.334464564919472,0.225665086507797,5.37));
#44608=CARTESIAN_POINT('',(-0.334464564919472,0.225665086507797,5.4));
#44609=CARTESIAN_POINT('Ctrl Pts',(-0.334464564919472,0.225665086507797,
5.37));
#44610=CARTESIAN_POINT('Ctrl Pts',(-0.306514278054237,0.200341069698334,
5.37));
#44611=CARTESIAN_POINT('Ctrl Pts',(-0.26637102663517,0.200341069698334,
5.37));
#44612=CARTESIAN_POINT('Ctrl Pts',(-0.374045148491859,0.308390179276466,
5.4));
#44613=CARTESIAN_POINT('Ctrl Pts',(-0.374045148491859,0.308390179276466,
5.37));
#44614=CARTESIAN_POINT('Ctrl Pts',(-0.362414851784706,0.250989103317261,
5.4));
#44615=CARTESIAN_POINT('Ctrl Pts',(-0.362414851784706,0.250989103317261,
5.37));
#44616=CARTESIAN_POINT('Ctrl Pts',(-0.334464564919472,0.225665086507797,
5.4));
#44617=CARTESIAN_POINT('Ctrl Pts',(-0.334464564919472,0.225665086507797,
5.37));
#44618=CARTESIAN_POINT('',(-0.374045148491859,0.308390179276466,5.4));
#44619=CARTESIAN_POINT('Ctrl Pts',(-0.374045148491859,0.308390179276466,
5.4));
#44620=CARTESIAN_POINT('Ctrl Pts',(-0.362414851784706,0.250989103317261,
5.4));
#44621=CARTESIAN_POINT('Ctrl Pts',(-0.334464564919472,0.225665086507797,
5.4));
#44622=CARTESIAN_POINT('',(-0.374045148491859,0.308390179276466,5.37));
#44623=CARTESIAN_POINT('',(-0.374045148491859,0.308390179276466,5.4));
#44624=CARTESIAN_POINT('Ctrl Pts',(-0.374045148491859,0.308390179276466,
5.37));
#44625=CARTESIAN_POINT('Ctrl Pts',(-0.362414851784706,0.250989103317261,
5.37));
#44626=CARTESIAN_POINT('Ctrl Pts',(-0.334464564919472,0.225665086507797,
5.37));
#44627=CARTESIAN_POINT('Origin',(-0.441575780510902,0.299386093020439,5.4));
#44628=CARTESIAN_POINT('',(-0.441575780510902,0.299386093020439,5.4));
#44629=CARTESIAN_POINT('',(-0.244254895913005,0.325695550105545,5.4));
#44630=CARTESIAN_POINT('',(-0.441575780510902,0.299386093020439,5.37));
#44631=CARTESIAN_POINT('',(-0.441575780510902,0.299386093020439,5.4));
#44632=CARTESIAN_POINT('',(-0.441575780510902,0.299386093020439,5.37));
#44633=CARTESIAN_POINT('Ctrl Pts',(-0.386988416314125,0.187585258483887,
5.4));
#44634=CARTESIAN_POINT('Ctrl Pts',(-0.386988416314125,0.187585258483887,
5.37));
#44635=CARTESIAN_POINT('Ctrl Pts',(-0.43482281267643,0.230729871988297,
5.4));
#44636=CARTESIAN_POINT('Ctrl Pts',(-0.43482281267643,0.230729871988297,
5.37));
#44637=CARTESIAN_POINT('Ctrl Pts',(-0.441575780510902,0.299386093020439,
5.4));
#44638=CARTESIAN_POINT('Ctrl Pts',(-0.441575780510902,0.299386093020439,
5.37));
#44639=CARTESIAN_POINT('',(-0.386988416314125,0.187585258483887,5.4));
#44640=CARTESIAN_POINT('Ctrl Pts',(-0.386988416314125,0.187585258483887,
5.4));
#44641=CARTESIAN_POINT('Ctrl Pts',(-0.43482281267643,0.230729871988297,
5.4));
#44642=CARTESIAN_POINT('Ctrl Pts',(-0.441575780510902,0.299386093020439,
5.4));
#44643=CARTESIAN_POINT('',(-0.386988416314125,0.187585258483887,5.37));
#44644=CARTESIAN_POINT('',(-0.386988416314125,0.187585258483887,5.4));
#44645=CARTESIAN_POINT('Ctrl Pts',(-0.386988416314125,0.187585258483887,
5.37));
#44646=CARTESIAN_POINT('Ctrl Pts',(-0.43482281267643,0.230729871988297,
5.37));
#44647=CARTESIAN_POINT('Ctrl Pts',(-0.441575780510902,0.299386093020439,
5.37));
#44648=CARTESIAN_POINT('Ctrl Pts',(-0.266746297478676,0.144440674781799,
5.4));
#44649=CARTESIAN_POINT('Ctrl Pts',(-0.266746297478676,0.144440674781799,
5.37));
#44650=CARTESIAN_POINT('Ctrl Pts',(-0.339154258370399,0.144440674781799,
5.4));
#44651=CARTESIAN_POINT('Ctrl Pts',(-0.339154258370399,0.144440674781799,
5.37));
#44652=CARTESIAN_POINT('Ctrl Pts',(-0.386988416314125,0.187585258483887,
5.4));
#44653=CARTESIAN_POINT('Ctrl Pts',(-0.386988416314125,0.187585258483887,
5.37));
#44654=CARTESIAN_POINT('Ctrl Pts',(-0.266746297478676,0.144440674781799,
5.4));
#44655=CARTESIAN_POINT('Ctrl Pts',(-0.339154258370399,0.144440674781799,
5.4));
#44656=CARTESIAN_POINT('Ctrl Pts',(-0.386988416314125,0.187585258483887,
5.4));
#44657=CARTESIAN_POINT('Ctrl Pts',(-0.266746297478676,0.144440674781799,
5.37));
#44658=CARTESIAN_POINT('Ctrl Pts',(-0.339154258370399,0.144440674781799,
5.37));
#44659=CARTESIAN_POINT('Ctrl Pts',(-0.386988416314125,0.187585258483887,
5.37));
#44660=CARTESIAN_POINT('Origin',(-0.261493936181068,0.425443404912949,5.37));
#44661=CARTESIAN_POINT('Origin',(-1.13264001905918,0.387176015973091,5.4));
#44662=CARTESIAN_POINT('',(-1.13264001905918,0.387176015973091,5.4));
#44663=CARTESIAN_POINT('',(-0.925170674920082,0.387176015973091,5.4));
#44664=CARTESIAN_POINT('',(-0.566320009529591,0.387176015973091,5.4));
#44665=CARTESIAN_POINT('',(-1.13264001905918,0.387176015973091,5.37));
#44666=CARTESIAN_POINT('',(-1.13264001905918,0.387176015973091,5.4));
#44667=CARTESIAN_POINT('',(-0.925170674920082,0.387176015973091,5.37));
#44668=CARTESIAN_POINT('',(-1.13264001905918,0.387176015973091,5.37));
#44669=CARTESIAN_POINT('',(-0.925170674920082,0.387176015973091,5.4));
#44670=CARTESIAN_POINT('Origin',(-1.13264001905918,0.319270142912865,5.4));
#44671=CARTESIAN_POINT('',(-1.13264001905918,0.319270142912865,5.4));
#44672=CARTESIAN_POINT('',(-1.13264001905918,0.159635071456432,5.4));
#44673=CARTESIAN_POINT('',(-1.13264001905918,0.319270142912865,5.37));
#44674=CARTESIAN_POINT('',(-1.13264001905918,0.319270142912865,5.4));
#44675=CARTESIAN_POINT('',(-1.13264001905918,0.319270142912865,5.37));
#44676=CARTESIAN_POINT('Origin',(-0.925170674920082,0.319270142912865,5.4));
#44677=CARTESIAN_POINT('',(-0.925170674920082,0.319270142912865,5.4));
#44678=CARTESIAN_POINT('',(-0.462585337460041,0.319270142912865,5.4));
#44679=CARTESIAN_POINT('',(-0.925170674920082,0.319270142912865,5.37));
#44680=CARTESIAN_POINT('',(-0.925170674920082,0.319270142912865,5.4));
#44681=CARTESIAN_POINT('',(-0.925170674920082,0.319270142912865,5.37));
#44682=CARTESIAN_POINT('Origin',(-0.925170674920082,0.387176015973091,5.4));
#44683=CARTESIAN_POINT('',(-0.925170674920082,0.193588007986546,5.4));
#44684=CARTESIAN_POINT('',(-0.925170674920082,0.387176015973091,5.37));
#44685=CARTESIAN_POINT('Origin',(-1.02890534698963,0.353223079442978,5.37));
#44686=CARTESIAN_POINT('Ctrl Pts',(-1.93437947332859,0.646418863534927,
5.4));
#44687=CARTESIAN_POINT('Ctrl Pts',(-1.93437947332859,0.646418863534927,
5.37));
#44688=CARTESIAN_POINT('Ctrl Pts',(-1.94488431513309,0.593519800901413,
5.4));
#44689=CARTESIAN_POINT('Ctrl Pts',(-1.94488431513309,0.593519800901413,
5.37));
#44690=CARTESIAN_POINT('Ctrl Pts',(-1.96401788294315,0.541371101140976,
5.4));
#44691=CARTESIAN_POINT('Ctrl Pts',(-1.96401788294315,0.541371101140976,
5.37));
#44692=CARTESIAN_POINT('',(-1.93437947332859,0.646418863534927,5.4));
#44693=CARTESIAN_POINT('',(-1.96401788294315,0.541371101140976,5.4));
#44694=CARTESIAN_POINT('Ctrl Pts',(-1.93437947332859,0.646418863534927,
5.4));
#44695=CARTESIAN_POINT('Ctrl Pts',(-1.94488431513309,0.593519800901413,
5.4));
#44696=CARTESIAN_POINT('Ctrl Pts',(-1.96401788294315,0.541371101140976,
5.4));
#44697=CARTESIAN_POINT('',(-1.93437947332859,0.646418863534927,5.37));
#44698=CARTESIAN_POINT('',(-1.93437947332859,0.646418863534927,5.4));
#44699=CARTESIAN_POINT('',(-1.96401788294315,0.541371101140976,5.37));
#44700=CARTESIAN_POINT('Ctrl Pts',(-1.93437947332859,0.646418863534927,
5.37));
#44701=CARTESIAN_POINT('Ctrl Pts',(-1.94488431513309,0.593519800901413,
5.37));
#44702=CARTESIAN_POINT('Ctrl Pts',(-1.96401788294315,0.541371101140976,
5.37));
#44703=CARTESIAN_POINT('',(-1.96401788294315,0.541371101140976,5.4));
#44704=CARTESIAN_POINT('Ctrl Pts',(-1.89536167681217,0.532367014884949,
5.4));
#44705=CARTESIAN_POINT('Ctrl Pts',(-1.89536167681217,0.532367014884949,
5.37));
#44706=CARTESIAN_POINT('Ctrl Pts',(-1.92162372171879,0.601773554086685,
5.4));
#44707=CARTESIAN_POINT('Ctrl Pts',(-1.92162372171879,0.601773554086685,
5.37));
#44708=CARTESIAN_POINT('Ctrl Pts',(-1.93437947332859,0.646418863534927,
5.4));
#44709=CARTESIAN_POINT('Ctrl Pts',(-1.93437947332859,0.646418863534927,
5.37));
#44710=CARTESIAN_POINT('',(-1.89536167681217,0.532367014884949,5.4));
#44711=CARTESIAN_POINT('Ctrl Pts',(-1.89536167681217,0.532367014884949,
5.4));
#44712=CARTESIAN_POINT('Ctrl Pts',(-1.92162372171879,0.601773554086685,
5.4));
#44713=CARTESIAN_POINT('Ctrl Pts',(-1.93437947332859,0.646418863534927,
5.4));
#44714=CARTESIAN_POINT('',(-1.89536167681217,0.532367014884949,5.37));
#44715=CARTESIAN_POINT('',(-1.89536167681217,0.532367014884949,5.4));
#44716=CARTESIAN_POINT('Ctrl Pts',(-1.89536167681217,0.532367014884949,
5.37));
#44717=CARTESIAN_POINT('Ctrl Pts',(-1.92162372171879,0.601773554086685,
5.37));
#44718=CARTESIAN_POINT('Ctrl Pts',(-1.93437947332859,0.646418863534927,
5.37));
#44719=CARTESIAN_POINT('Origin',(-1.83796061575413,0.380047762393951,5.4));
#44720=CARTESIAN_POINT('',(-1.83796061575413,0.380047762393951,5.4));
#44721=CARTESIAN_POINT('',(-1.66097698357881,-0.089595377631381,5.4));
#44722=CARTESIAN_POINT('',(-1.83796061575413,0.380047762393951,5.37));
#44723=CARTESIAN_POINT('',(-1.83796061575413,0.380047762393951,5.4));
#44724=CARTESIAN_POINT('',(-1.83796061575413,0.380047762393951,5.37));
#44725=CARTESIAN_POINT('Origin',(-2.02442039549351,0.380047762393951,5.4));
#44726=CARTESIAN_POINT('',(-2.02442039549351,0.380047762393951,5.4));
#44727=CARTESIAN_POINT('',(-1.01221019774675,0.380047762393951,5.4));
#44728=CARTESIAN_POINT('',(-2.02442039549351,0.380047762393951,5.37));
#44729=CARTESIAN_POINT('',(-2.02442039549351,0.380047762393951,5.4));
#44730=CARTESIAN_POINT('',(-2.02442039549351,0.380047762393951,5.37));
#44731=CARTESIAN_POINT('Origin',(-1.96401788294315,0.541371101140976,5.4));
#44732=CARTESIAN_POINT('',(-1.93216564827672,0.626442212026634,5.4));
#44733=CARTESIAN_POINT('',(-1.96401788294315,0.541371101140976,5.37));
#44734=CARTESIAN_POINT('Origin',(-1.81545044481754,0.320770823955536,5.4));
#44735=CARTESIAN_POINT('',(-1.81545044481754,0.320770823955536,5.4));
#44736=CARTESIAN_POINT('',(-2.04542995989323,0.320770823955536,5.4));
#44737=CARTESIAN_POINT('',(-0.907725222408772,0.320770823955536,5.4));
#44738=CARTESIAN_POINT('',(-1.81545044481754,0.320770823955536,5.37));
#44739=CARTESIAN_POINT('',(-1.81545044481754,0.320770823955536,5.4));
#44740=CARTESIAN_POINT('',(-2.04542995989323,0.320770823955536,5.37));
#44741=CARTESIAN_POINT('',(-1.81545044481754,0.320770823955536,5.37));
#44742=CARTESIAN_POINT('',(-2.04542995989323,0.320770823955536,5.4));
#44743=CARTESIAN_POINT('Origin',(-1.75129629671574,0.154195094108582,5.4));
#44744=CARTESIAN_POINT('',(-1.75129629671574,0.154195094108582,5.4));
#44745=CARTESIAN_POINT('',(-1.61233179129081,-0.206625127169145,5.4));
#44746=CARTESIAN_POINT('',(-1.75129629671574,0.154195094108582,5.37));
#44747=CARTESIAN_POINT('',(-1.75129629671574,0.154195094108582,5.4));
#44748=CARTESIAN_POINT('',(-1.75129629671574,0.154195094108582,5.37));
#44749=CARTESIAN_POINT('Origin',(-1.6683836132288,0.154195094108582,5.4));
#44750=CARTESIAN_POINT('',(-1.6683836132288,0.154195094108582,5.4));
#44751=CARTESIAN_POINT('',(-0.834191806614399,0.154195094108582,5.4));
#44752=CARTESIAN_POINT('',(-1.6683836132288,0.154195094108582,5.37));
#44753=CARTESIAN_POINT('',(-1.6683836132288,0.154195094108582,5.4));
#44754=CARTESIAN_POINT('',(-1.6683836132288,0.154195094108582,5.37));
#44755=CARTESIAN_POINT('Origin',(-1.89348591864109,0.704195106029511,5.4));
#44756=CARTESIAN_POINT('',(-1.89348591864109,0.704195106029511,5.4));
#44757=CARTESIAN_POINT('',(-1.63422248259755,0.0707280579980082,5.4));
#44758=CARTESIAN_POINT('',(-1.89348591864109,0.704195106029511,5.37));
#44759=CARTESIAN_POINT('',(-1.89348591864109,0.704195106029511,5.4));
#44760=CARTESIAN_POINT('',(-1.89348591864109,0.704195106029511,5.37));
#44761=CARTESIAN_POINT('Origin',(-1.97189654409885,0.704195106029511,5.4));
#44762=CARTESIAN_POINT('',(-1.97189654409885,0.704195106029511,5.4));
#44763=CARTESIAN_POINT('',(-0.985948272049427,0.704195106029511,5.4));
#44764=CARTESIAN_POINT('',(-1.97189654409885,0.704195106029511,5.37));
#44765=CARTESIAN_POINT('',(-1.97189654409885,0.704195106029511,5.4));
#44766=CARTESIAN_POINT('',(-1.97189654409885,0.704195106029511,5.37));
#44767=CARTESIAN_POINT('Origin',(-2.18311752378941,0.154195094108582,5.4));
#44768=CARTESIAN_POINT('',(-2.18311752378941,0.154195094108582,5.4));
#44769=CARTESIAN_POINT('',(-2.06862327822368,0.452327583212093,5.4));
#44770=CARTESIAN_POINT('',(-2.18311752378941,0.154195094108582,5.37));
#44771=CARTESIAN_POINT('',(-2.18311752378941,0.154195094108582,5.4));
#44772=CARTESIAN_POINT('',(-2.18311752378941,0.154195094108582,5.37));
#44773=CARTESIAN_POINT('Origin',(-2.10583241283894,0.154195094108582,5.4));
#44774=CARTESIAN_POINT('',(-2.10583241283894,0.154195094108582,5.4));
#44775=CARTESIAN_POINT('',(-1.05291620641947,0.154195094108582,5.4));
#44776=CARTESIAN_POINT('',(-2.10583241283894,0.154195094108582,5.37));
#44777=CARTESIAN_POINT('',(-2.10583241283894,0.154195094108582,5.4));
#44778=CARTESIAN_POINT('',(-2.10583241283894,0.154195094108582,5.37));
#44779=CARTESIAN_POINT('Origin',(-2.04542995989323,0.320770823955536,5.4));
#44780=CARTESIAN_POINT('',(-1.97798173193314,0.506777140775716,5.4));
#44781=CARTESIAN_POINT('',(-2.04542995989323,0.320770823955536,5.37));
#44782=CARTESIAN_POINT('Origin',(-1.9257505685091,0.429195100069046,5.37));
#44783=CARTESIAN_POINT('Ctrl Pts',(-1.40051163733006,0.144815826416016,
5.4));
#44784=CARTESIAN_POINT('Ctrl Pts',(-1.40051163733006,0.144815826416016,
5.37));
#44785=CARTESIAN_POINT('Ctrl Pts',(-1.47517050802708,0.144815826416016,
5.4));
#44786=CARTESIAN_POINT('Ctrl Pts',(-1.47517050802708,0.144815826416016,
5.37));
#44787=CARTESIAN_POINT('Ctrl Pts',(-1.5256309658289,0.16657572388649,5.4));
#44788=CARTESIAN_POINT('Ctrl Pts',(-1.5256309658289,0.16657572388649,5.37));
#44789=CARTESIAN_POINT('',(-1.40051163733006,0.144815826416016,5.4));
#44790=CARTESIAN_POINT('',(-1.5256309658289,0.16657572388649,5.4));
#44791=CARTESIAN_POINT('Ctrl Pts',(-1.40051163733006,0.144815826416016,
5.4));
#44792=CARTESIAN_POINT('Ctrl Pts',(-1.47517050802708,0.144815826416016,
5.4));
#44793=CARTESIAN_POINT('Ctrl Pts',(-1.5256309658289,0.16657572388649,5.4));
#44794=CARTESIAN_POINT('',(-1.40051163733006,0.144815826416016,5.37));
#44795=CARTESIAN_POINT('',(-1.40051163733006,0.144815826416016,5.4));
#44796=CARTESIAN_POINT('',(-1.5256309658289,0.16657572388649,5.37));
#44797=CARTESIAN_POINT('Ctrl Pts',(-1.40051163733006,0.144815826416016,
5.37));
#44798=CARTESIAN_POINT('Ctrl Pts',(-1.47517050802708,0.144815826416016,
5.37));
#44799=CARTESIAN_POINT('Ctrl Pts',(-1.5256309658289,0.16657572388649,5.37));
#44800=CARTESIAN_POINT('',(-1.5256309658289,0.16657572388649,5.4));
#44801=CARTESIAN_POINT('Ctrl Pts',(-1.29452587664127,0.166388148069382,
5.4));
#44802=CARTESIAN_POINT('Ctrl Pts',(-1.29452587664127,0.166388148069382,
5.37));
#44803=CARTESIAN_POINT('Ctrl Pts',(-1.34160985052586,0.144815826416016,
5.4));
#44804=CARTESIAN_POINT('Ctrl Pts',(-1.34160985052586,0.144815826416016,
5.37));
#44805=CARTESIAN_POINT('Ctrl Pts',(-1.40051163733006,0.144815826416016,
5.4));
#44806=CARTESIAN_POINT('Ctrl Pts',(-1.40051163733006,0.144815826416016,
5.37));
#44807=CARTESIAN_POINT('',(-1.29452587664127,0.166388148069382,5.4));
#44808=CARTESIAN_POINT('Ctrl Pts',(-1.29452587664127,0.166388148069382,
5.4));
#44809=CARTESIAN_POINT('Ctrl Pts',(-1.34160985052586,0.144815826416016,
5.4));
#44810=CARTESIAN_POINT('Ctrl Pts',(-1.40051163733006,0.144815826416016,
5.4));
#44811=CARTESIAN_POINT('',(-1.29452587664127,0.166388148069382,5.37));
#44812=CARTESIAN_POINT('',(-1.29452587664127,0.166388148069382,5.4));
#44813=CARTESIAN_POINT('Ctrl Pts',(-1.29452587664127,0.166388148069382,
5.37));
#44814=CARTESIAN_POINT('Ctrl Pts',(-1.34160985052586,0.144815826416016,
5.37));
#44815=CARTESIAN_POINT('Ctrl Pts',(-1.40051163733006,0.144815826416016,
5.37));
#44816=CARTESIAN_POINT('Ctrl Pts',(-1.2223055511713,0.226790601015091,5.4));
#44817=CARTESIAN_POINT('Ctrl Pts',(-1.2223055511713,0.226790601015091,5.37));
#44818=CARTESIAN_POINT('Ctrl Pts',(-1.24744202196598,0.187960439920425,
5.4));
#44819=CARTESIAN_POINT('Ctrl Pts',(-1.24744202196598,0.187960439920425,
5.37));
#44820=CARTESIAN_POINT('Ctrl Pts',(-1.29452587664127,0.166388148069382,
5.4));
#44821=CARTESIAN_POINT('Ctrl Pts',(-1.29452587664127,0.166388148069382,
5.37));
#44822=CARTESIAN_POINT('',(-1.2223055511713,0.226790601015091,5.4));
#44823=CARTESIAN_POINT('Ctrl Pts',(-1.2223055511713,0.226790601015091,5.4));
#44824=CARTESIAN_POINT('Ctrl Pts',(-1.24744202196598,0.187960439920425,
5.4));
#44825=CARTESIAN_POINT('Ctrl Pts',(-1.29452587664127,0.166388148069382,
5.4));
#44826=CARTESIAN_POINT('',(-1.2223055511713,0.226790601015091,5.37));
#44827=CARTESIAN_POINT('',(-1.2223055511713,0.226790601015091,5.4));
#44828=CARTESIAN_POINT('Ctrl Pts',(-1.2223055511713,0.226790601015091,5.37));
#44829=CARTESIAN_POINT('Ctrl Pts',(-1.24744202196598,0.187960439920425,
5.37));
#44830=CARTESIAN_POINT('Ctrl Pts',(-1.29452587664127,0.166388148069382,
5.37));
#44831=CARTESIAN_POINT('Ctrl Pts',(-1.19716919958591,0.30951569378376,5.4));
#44832=CARTESIAN_POINT('Ctrl Pts',(-1.19716919958591,0.30951569378376,5.37));
#44833=CARTESIAN_POINT('Ctrl Pts',(-1.19716919958591,0.265620732307434,
5.4));
#44834=CARTESIAN_POINT('Ctrl Pts',(-1.19716919958591,0.265620732307434,
5.37));
#44835=CARTESIAN_POINT('Ctrl Pts',(-1.2223055511713,0.226790601015091,5.4));
#44836=CARTESIAN_POINT('Ctrl Pts',(-1.2223055511713,0.226790601015091,5.37));
#44837=CARTESIAN_POINT('',(-1.19716919958591,0.30951569378376,5.4));
#44838=CARTESIAN_POINT('Ctrl Pts',(-1.19716919958591,0.30951569378376,5.4));
#44839=CARTESIAN_POINT('Ctrl Pts',(-1.19716919958591,0.265620732307434,
5.4));
#44840=CARTESIAN_POINT('Ctrl Pts',(-1.2223055511713,0.226790601015091,5.4));
#44841=CARTESIAN_POINT('',(-1.19716919958591,0.30951569378376,5.37));
#44842=CARTESIAN_POINT('',(-1.19716919958591,0.30951569378376,5.4));
#44843=CARTESIAN_POINT('Ctrl Pts',(-1.19716919958591,0.30951569378376,5.37));
#44844=CARTESIAN_POINT('Ctrl Pts',(-1.19716919958591,0.265620732307434,
5.37));
#44845=CARTESIAN_POINT('Ctrl Pts',(-1.2223055511713,0.226790601015091,5.37));
#44846=CARTESIAN_POINT('Ctrl Pts',(-1.220054641366,0.387738758325577,5.4));
#44847=CARTESIAN_POINT('Ctrl Pts',(-1.220054641366,0.387738758325577,5.37));
#44848=CARTESIAN_POINT('Ctrl Pts',(-1.19716919958591,0.353785821795464,
5.4));
#44849=CARTESIAN_POINT('Ctrl Pts',(-1.19716919958591,0.353785821795464,
5.37));
#44850=CARTESIAN_POINT('Ctrl Pts',(-1.19716919958591,0.30951569378376,5.4));
#44851=CARTESIAN_POINT('Ctrl Pts',(-1.19716919958591,0.30951569378376,5.37));
#44852=CARTESIAN_POINT('',(-1.220054641366,0.387738758325577,5.4));
#44853=CARTESIAN_POINT('Ctrl Pts',(-1.220054641366,0.387738758325577,5.4));
#44854=CARTESIAN_POINT('Ctrl Pts',(-1.19716919958591,0.353785821795464,
5.4));
#44855=CARTESIAN_POINT('Ctrl Pts',(-1.19716919958591,0.30951569378376,5.4));
#44856=CARTESIAN_POINT('',(-1.220054641366,0.387738758325577,5.37));
#44857=CARTESIAN_POINT('',(-1.220054641366,0.387738758325577,5.4));
#44858=CARTESIAN_POINT('Ctrl Pts',(-1.220054641366,0.387738758325577,5.37));
#44859=CARTESIAN_POINT('Ctrl Pts',(-1.19716919958591,0.353785821795464,
5.37));
#44860=CARTESIAN_POINT('Ctrl Pts',(-1.19716919958591,0.30951569378376,5.37));
#44861=CARTESIAN_POINT('Ctrl Pts',(-1.29096175730228,0.443826758861542,
5.4));
#44862=CARTESIAN_POINT('Ctrl Pts',(-1.29096175730228,0.443826758861542,
5.37));
#44863=CARTESIAN_POINT('Ctrl Pts',(-1.24293996393681,0.421691679954529,
5.4));
#44864=CARTESIAN_POINT('Ctrl Pts',(-1.24293996393681,0.421691679954529,
5.37));
#44865=CARTESIAN_POINT('Ctrl Pts',(-1.220054641366,0.387738758325577,5.4));
#44866=CARTESIAN_POINT('Ctrl Pts',(-1.220054641366,0.387738758325577,5.37));
#44867=CARTESIAN_POINT('',(-1.29096175730228,0.443826758861542,5.4));
#44868=CARTESIAN_POINT('Ctrl Pts',(-1.29096175730228,0.443826758861542,
5.4));
#44869=CARTESIAN_POINT('Ctrl Pts',(-1.24293996393681,0.421691679954529,
5.4));
#44870=CARTESIAN_POINT('Ctrl Pts',(-1.220054641366,0.387738758325577,5.4));
#44871=CARTESIAN_POINT('',(-1.29096175730228,0.443826758861542,5.37));
#44872=CARTESIAN_POINT('',(-1.29096175730228,0.443826758861542,5.4));
#44873=CARTESIAN_POINT('Ctrl Pts',(-1.29096175730228,0.443826758861542,
5.37));
#44874=CARTESIAN_POINT('Ctrl Pts',(-1.24293996393681,0.421691679954529,
5.37));
#44875=CARTESIAN_POINT('Ctrl Pts',(-1.220054641366,0.387738758325577,5.37));
#44876=CARTESIAN_POINT('Ctrl Pts',(-1.41270472109318,0.478905194997787,
5.4));
#44877=CARTESIAN_POINT('Ctrl Pts',(-1.41270472109318,0.478905194997787,
5.37));
#44878=CARTESIAN_POINT('Ctrl Pts',(-1.32397677004337,0.458833569288254,
5.4));
#44879=CARTESIAN_POINT('Ctrl Pts',(-1.32397677004337,0.458833569288254,
5.37));
#44880=CARTESIAN_POINT('Ctrl Pts',(-1.29096175730228,0.443826758861542,
5.4));
#44881=CARTESIAN_POINT('Ctrl Pts',(-1.29096175730228,0.443826758861542,
5.37));
#44882=CARTESIAN_POINT('',(-1.41270472109318,0.478905194997787,5.4));
#44883=CARTESIAN_POINT('Ctrl Pts',(-1.41270472109318,0.478905194997787,
5.4));
#44884=CARTESIAN_POINT('Ctrl Pts',(-1.32397677004337,0.458833569288254,
5.4));
#44885=CARTESIAN_POINT('Ctrl Pts',(-1.29096175730228,0.443826758861542,
5.4));
#44886=CARTESIAN_POINT('',(-1.41270472109318,0.478905194997787,5.37));
#44887=CARTESIAN_POINT('',(-1.41270472109318,0.478905194997787,5.4));
#44888=CARTESIAN_POINT('Ctrl Pts',(-1.41270472109318,0.478905194997787,
5.37));
#44889=CARTESIAN_POINT('Ctrl Pts',(-1.32397677004337,0.458833569288254,
5.37));
#44890=CARTESIAN_POINT('Ctrl Pts',(-1.29096175730228,0.443826758861542,
5.37));
#44891=CARTESIAN_POINT('Ctrl Pts',(-1.52244199812412,0.518110537528992,
5.4));
#44892=CARTESIAN_POINT('Ctrl Pts',(-1.52244199812412,0.518110537528992,
5.37));
#44893=CARTESIAN_POINT('Ctrl Pts',(-1.5014324337244,0.498976820707321,5.4));
#44894=CARTESIAN_POINT('Ctrl Pts',(-1.5014324337244,0.498976820707321,5.37));
#44895=CARTESIAN_POINT('Ctrl Pts',(-1.41270472109318,0.478905194997787,
5.4));
#44896=CARTESIAN_POINT('Ctrl Pts',(-1.41270472109318,0.478905194997787,
5.37));
#44897=CARTESIAN_POINT('',(-1.52244199812412,0.518110537528992,5.4));
#44898=CARTESIAN_POINT('Ctrl Pts',(-1.52244199812412,0.518110537528992,
5.4));
#44899=CARTESIAN_POINT('Ctrl Pts',(-1.5014324337244,0.498976820707321,5.4));
#44900=CARTESIAN_POINT('Ctrl Pts',(-1.41270472109318,0.478905194997787,
5.4));
#44901=CARTESIAN_POINT('',(-1.52244199812412,0.518110537528992,5.37));
#44902=CARTESIAN_POINT('',(-1.52244199812412,0.518110537528992,5.4));
#44903=CARTESIAN_POINT('Ctrl Pts',(-1.52244199812412,0.518110537528992,
5.37));
#44904=CARTESIAN_POINT('Ctrl Pts',(-1.5014324337244,0.498976820707321,5.37));
#44905=CARTESIAN_POINT('Ctrl Pts',(-1.41270472109318,0.478905194997787,
5.37));
#44906=CARTESIAN_POINT('Ctrl Pts',(-1.54382671415806,0.566882693767548,
5.4));
#44907=CARTESIAN_POINT('Ctrl Pts',(-1.54382671415806,0.566882693767548,
5.37));
#44908=CARTESIAN_POINT('Ctrl Pts',(-1.54382671415806,0.53724422454834,5.4));
#44909=CARTESIAN_POINT('Ctrl Pts',(-1.54382671415806,0.53724422454834,5.37));
#44910=CARTESIAN_POINT('Ctrl Pts',(-1.52244199812412,0.518110537528992,
5.4));
#44911=CARTESIAN_POINT('Ctrl Pts',(-1.52244199812412,0.518110537528992,
5.37));
#44912=CARTESIAN_POINT('',(-1.54382671415806,0.566882693767548,5.4));
#44913=CARTESIAN_POINT('Ctrl Pts',(-1.54382671415806,0.566882693767548,
5.4));
#44914=CARTESIAN_POINT('Ctrl Pts',(-1.54382671415806,0.53724422454834,5.4));
#44915=CARTESIAN_POINT('Ctrl Pts',(-1.52244199812412,0.518110537528992,
5.4));
#44916=CARTESIAN_POINT('',(-1.54382671415806,0.566882693767548,5.37));
#44917=CARTESIAN_POINT('',(-1.54382671415806,0.566882693767548,5.4));
#44918=CARTESIAN_POINT('Ctrl Pts',(-1.54382671415806,0.566882693767548,
5.37));
#44919=CARTESIAN_POINT('Ctrl Pts',(-1.54382671415806,0.53724422454834,5.37));
#44920=CARTESIAN_POINT('Ctrl Pts',(-1.52244199812412,0.518110537528992,
5.37));
#44921=CARTESIAN_POINT('Ctrl Pts',(-1.51362551748753,0.6252217233181,5.4));
#44922=CARTESIAN_POINT('Ctrl Pts',(-1.51362551748753,0.6252217233181,5.37));
#44923=CARTESIAN_POINT('Ctrl Pts',(-1.54382671415806,0.60102322101593,5.4));
#44924=CARTESIAN_POINT('Ctrl Pts',(-1.54382671415806,0.60102322101593,5.37));
#44925=CARTESIAN_POINT('Ctrl Pts',(-1.54382671415806,0.566882693767548,
5.4));
#44926=CARTESIAN_POINT('Ctrl Pts',(-1.54382671415806,0.566882693767548,
5.37));
#44927=CARTESIAN_POINT('',(-1.51362551748753,0.6252217233181,5.4));
#44928=CARTESIAN_POINT('Ctrl Pts',(-1.51362551748753,0.6252217233181,5.4));
#44929=CARTESIAN_POINT('Ctrl Pts',(-1.54382671415806,0.60102322101593,5.4));
#44930=CARTESIAN_POINT('Ctrl Pts',(-1.54382671415806,0.566882693767548,
5.4));
#44931=CARTESIAN_POINT('',(-1.51362551748753,0.6252217233181,5.37));
#44932=CARTESIAN_POINT('',(-1.51362551748753,0.6252217233181,5.4));
#44933=CARTESIAN_POINT('Ctrl Pts',(-1.51362551748753,0.6252217233181,5.37));
#44934=CARTESIAN_POINT('Ctrl Pts',(-1.54382671415806,0.60102322101593,5.37));
#44935=CARTESIAN_POINT('Ctrl Pts',(-1.54382671415806,0.566882693767548,
5.37));
#44936=CARTESIAN_POINT('Ctrl Pts',(-1.41739429533482,0.64942022562027,5.4));
#44937=CARTESIAN_POINT('Ctrl Pts',(-1.41739429533482,0.64942022562027,5.37));
#44938=CARTESIAN_POINT('Ctrl Pts',(-1.48342432081699,0.64942022562027,5.4));
#44939=CARTESIAN_POINT('Ctrl Pts',(-1.48342432081699,0.64942022562027,5.37));
#44940=CARTESIAN_POINT('Ctrl Pts',(-1.51362551748753,0.6252217233181,5.4));
#44941=CARTESIAN_POINT('Ctrl Pts',(-1.51362551748753,0.6252217233181,5.37));
#44942=CARTESIAN_POINT('',(-1.41739429533482,0.64942022562027,5.4));
#44943=CARTESIAN_POINT('Ctrl Pts',(-1.41739429533482,0.64942022562027,5.4));
#44944=CARTESIAN_POINT('Ctrl Pts',(-1.48342432081699,0.64942022562027,5.4));
#44945=CARTESIAN_POINT('Ctrl Pts',(-1.51362551748753,0.6252217233181,5.4));
#44946=CARTESIAN_POINT('',(-1.41739429533482,0.64942022562027,5.37));
#44947=CARTESIAN_POINT('',(-1.41739429533482,0.64942022562027,5.4));
#44948=CARTESIAN_POINT('Ctrl Pts',(-1.41739429533482,0.64942022562027,5.37));
#44949=CARTESIAN_POINT('Ctrl Pts',(-1.48342432081699,0.64942022562027,5.37));
#44950=CARTESIAN_POINT('Ctrl Pts',(-1.51362551748753,0.6252217233181,5.37));
#44951=CARTESIAN_POINT('Ctrl Pts',(-1.32153822481632,0.622783118486404,
5.4));
#44952=CARTESIAN_POINT('Ctrl Pts',(-1.32153822481632,0.622783118486404,
5.37));
#44953=CARTESIAN_POINT('Ctrl Pts',(-1.35399045050144,0.64942022562027,5.4));
#44954=CARTESIAN_POINT('Ctrl Pts',(-1.35399045050144,0.64942022562027,5.37));
#44955=CARTESIAN_POINT('Ctrl Pts',(-1.41739429533482,0.64942022562027,5.4));
#44956=CARTESIAN_POINT('Ctrl Pts',(-1.41739429533482,0.64942022562027,5.37));
#44957=CARTESIAN_POINT('',(-1.32153822481632,0.622783118486404,5.4));
#44958=CARTESIAN_POINT('Ctrl Pts',(-1.32153822481632,0.622783118486404,
5.4));
#44959=CARTESIAN_POINT('Ctrl Pts',(-1.35399045050144,0.64942022562027,5.4));
#44960=CARTESIAN_POINT('Ctrl Pts',(-1.41739429533482,0.64942022562027,5.4));
#44961=CARTESIAN_POINT('',(-1.32153822481632,0.622783118486404,5.37));
#44962=CARTESIAN_POINT('',(-1.32153822481632,0.622783118486404,5.4));
#44963=CARTESIAN_POINT('Ctrl Pts',(-1.32153822481632,0.622783118486404,
5.37));
#44964=CARTESIAN_POINT('Ctrl Pts',(-1.35399045050144,0.64942022562027,5.37));
#44965=CARTESIAN_POINT('Ctrl Pts',(-1.41739429533482,0.64942022562027,5.37));
#44966=CARTESIAN_POINT('Ctrl Pts',(-1.28345836699009,0.54399728178978,5.4));
#44967=CARTESIAN_POINT('Ctrl Pts',(-1.28345836699009,0.54399728178978,5.37));
#44968=CARTESIAN_POINT('Ctrl Pts',(-1.2890859991312,0.596146011352539,5.4));
#44969=CARTESIAN_POINT('Ctrl Pts',(-1.2890859991312,0.596146011352539,5.37));
#44970=CARTESIAN_POINT('Ctrl Pts',(-1.32153822481632,0.622783118486404,
5.4));
#44971=CARTESIAN_POINT('Ctrl Pts',(-1.32153822481632,0.622783118486404,
5.37));
#44972=CARTESIAN_POINT('',(-1.28345836699009,0.54399728178978,5.4));
#44973=CARTESIAN_POINT('Ctrl Pts',(-1.28345836699009,0.54399728178978,5.4));
#44974=CARTESIAN_POINT('Ctrl Pts',(-1.2890859991312,0.596146011352539,5.4));
#44975=CARTESIAN_POINT('Ctrl Pts',(-1.32153822481632,0.622783118486404,
5.4));
#44976=CARTESIAN_POINT('',(-1.28345836699009,0.54399728178978,5.37));
#44977=CARTESIAN_POINT('',(-1.28345836699009,0.54399728178978,5.4));
#44978=CARTESIAN_POINT('Ctrl Pts',(-1.28345836699009,0.54399728178978,5.37));
#44979=CARTESIAN_POINT('Ctrl Pts',(-1.2890859991312,0.596146011352539,5.37));
#44980=CARTESIAN_POINT('Ctrl Pts',(-1.32153822481632,0.622783118486404,
5.37));
#44981=CARTESIAN_POINT('Origin',(-1.21367670595646,0.549249672889709,5.4));
#44982=CARTESIAN_POINT('',(-1.21367670595646,0.549249672889709,5.4));
#44983=CARTESIAN_POINT('',(-0.630811244176041,0.59312133370381,5.4));
#44984=CARTESIAN_POINT('',(-1.21367670595646,0.549249672889709,5.37));
#44985=CARTESIAN_POINT('',(-1.21367670595646,0.549249672889709,5.4));
#44986=CARTESIAN_POINT('',(-1.21367670595646,0.549249672889709,5.37));
#44987=CARTESIAN_POINT('Ctrl Pts',(-1.24068893492222,0.635914081335068,
5.4));
#44988=CARTESIAN_POINT('Ctrl Pts',(-1.24068893492222,0.635914081335068,
5.37));
#44989=CARTESIAN_POINT('Ctrl Pts',(-1.21555258333683,0.597646677494049,
5.4));
#44990=CARTESIAN_POINT('Ctrl Pts',(-1.21555258333683,0.597646677494049,
5.37));
#44991=CARTESIAN_POINT('Ctrl Pts',(-1.21367670595646,0.549249672889709,
5.4));
#44992=CARTESIAN_POINT('Ctrl Pts',(-1.21367670595646,0.549249672889709,
5.37));
#44993=CARTESIAN_POINT('',(-1.24068893492222,0.635914081335068,5.4));
#44994=CARTESIAN_POINT('Ctrl Pts',(-1.24068893492222,0.635914081335068,
5.4));
#44995=CARTESIAN_POINT('Ctrl Pts',(-1.21555258333683,0.597646677494049,
5.4));
#44996=CARTESIAN_POINT('Ctrl Pts',(-1.21367670595646,0.549249672889709,
5.4));
#44997=CARTESIAN_POINT('',(-1.24068893492222,0.635914081335068,5.37));
#44998=CARTESIAN_POINT('',(-1.24068893492222,0.635914081335068,5.4));
#44999=CARTESIAN_POINT('Ctrl Pts',(-1.24068893492222,0.635914081335068,
5.37));
#45000=CARTESIAN_POINT('Ctrl Pts',(-1.21555258333683,0.597646677494049,
5.37));
#45001=CARTESIAN_POINT('Ctrl Pts',(-1.21367670595646,0.549249672889709,
5.37));
#45002=CARTESIAN_POINT('Ctrl Pts',(-1.31253410875797,0.693877899646759,
5.4));
#45003=CARTESIAN_POINT('Ctrl Pts',(-1.31253410875797,0.693877899646759,
5.37));
#45004=CARTESIAN_POINT('Ctrl Pts',(-1.2658254057169,0.674181485176086,5.4));
#45005=CARTESIAN_POINT('Ctrl Pts',(-1.2658254057169,0.674181485176086,5.37));
#45006=CARTESIAN_POINT('Ctrl Pts',(-1.24068893492222,0.635914081335068,
5.4));
#45007=CARTESIAN_POINT('Ctrl Pts',(-1.24068893492222,0.635914081335068,
5.37));
#45008=CARTESIAN_POINT('',(-1.31253410875797,0.693877899646759,5.4));
#45009=CARTESIAN_POINT('Ctrl Pts',(-1.31253410875797,0.693877899646759,
5.4));
#45010=CARTESIAN_POINT('Ctrl Pts',(-1.2658254057169,0.674181485176086,5.4));
#45011=CARTESIAN_POINT('Ctrl Pts',(-1.24068893492222,0.635914081335068,
5.4));
#45012=CARTESIAN_POINT('',(-1.31253410875797,0.693877899646759,5.37));
#45013=CARTESIAN_POINT('',(-1.31253410875797,0.693877899646759,5.4));
#45014=CARTESIAN_POINT('Ctrl Pts',(-1.31253410875797,0.693877899646759,
5.37));
#45015=CARTESIAN_POINT('Ctrl Pts',(-1.2658254057169,0.674181485176086,5.37));
#45016=CARTESIAN_POINT('Ctrl Pts',(-1.24068893492222,0.635914081335068,
5.37));
#45017=CARTESIAN_POINT('Ctrl Pts',(-1.42039562761784,0.713574373722076,
5.4));
#45018=CARTESIAN_POINT('Ctrl Pts',(-1.42039562761784,0.713574373722076,
5.37));
#45019=CARTESIAN_POINT('Ctrl Pts',(-1.35924281179905,0.713574373722076,
5.4));
#45020=CARTESIAN_POINT('Ctrl Pts',(-1.35924281179905,0.713574373722076,
5.37));
#45021=CARTESIAN_POINT('Ctrl Pts',(-1.31253410875797,0.693877899646759,
5.4));
#45022=CARTESIAN_POINT('Ctrl Pts',(-1.31253410875797,0.693877899646759,
5.37));
#45023=CARTESIAN_POINT('',(-1.42039562761784,0.713574373722076,5.4));
#45024=CARTESIAN_POINT('Ctrl Pts',(-1.42039562761784,0.713574373722076,
5.4));
#45025=CARTESIAN_POINT('Ctrl Pts',(-1.35924281179905,0.713574373722076,
5.4));
#45026=CARTESIAN_POINT('Ctrl Pts',(-1.31253410875797,0.693877899646759,
5.4));
#45027=CARTESIAN_POINT('',(-1.42039562761784,0.713574373722076,5.37));
#45028=CARTESIAN_POINT('',(-1.42039562761784,0.713574373722076,5.4));
#45029=CARTESIAN_POINT('Ctrl Pts',(-1.42039562761784,0.713574373722076,
5.37));
#45030=CARTESIAN_POINT('Ctrl Pts',(-1.35924281179905,0.713574373722076,
5.37));
#45031=CARTESIAN_POINT('Ctrl Pts',(-1.31253410875797,0.693877899646759,
5.37));
#45032=CARTESIAN_POINT('Ctrl Pts',(-1.52131654322147,0.694815838336945,
5.4));
#45033=CARTESIAN_POINT('Ctrl Pts',(-1.52131654322147,0.694815838336945,
5.37));
#45034=CARTESIAN_POINT('Ctrl Pts',(-1.4759209305048,0.713574373722076,5.4));
#45035=CARTESIAN_POINT('Ctrl Pts',(-1.4759209305048,0.713574373722076,5.37));
#45036=CARTESIAN_POINT('Ctrl Pts',(-1.42039562761784,0.713574373722076,
5.4));
#45037=CARTESIAN_POINT('Ctrl Pts',(-1.42039562761784,0.713574373722076,
5.37));
#45038=CARTESIAN_POINT('',(-1.52131654322147,0.694815838336945,5.4));
#45039=CARTESIAN_POINT('Ctrl Pts',(-1.52131654322147,0.694815838336945,
5.4));
#45040=CARTESIAN_POINT('Ctrl Pts',(-1.4759209305048,0.713574373722076,5.4));
#45041=CARTESIAN_POINT('Ctrl Pts',(-1.42039562761784,0.713574373722076,
5.4));
#45042=CARTESIAN_POINT('',(-1.52131654322147,0.694815838336945,5.37));
#45043=CARTESIAN_POINT('',(-1.52131654322147,0.694815838336945,5.4));
#45044=CARTESIAN_POINT('Ctrl Pts',(-1.52131654322147,0.694815838336945,
5.37));
#45045=CARTESIAN_POINT('Ctrl Pts',(-1.4759209305048,0.713574373722076,5.37));
#45046=CARTESIAN_POINT('Ctrl Pts',(-1.42039562761784,0.713574373722076,
5.37));
#45047=CARTESIAN_POINT('Ctrl Pts',(-1.59034790098667,0.639853382110596,
5.4));
#45048=CARTESIAN_POINT('Ctrl Pts',(-1.59034790098667,0.639853382110596,
5.37));
#45049=CARTESIAN_POINT('Ctrl Pts',(-1.56671215593815,0.676057302951813,
5.4));
#45050=CARTESIAN_POINT('Ctrl Pts',(-1.56671215593815,0.676057302951813,
5.37));
#45051=CARTESIAN_POINT('Ctrl Pts',(-1.52131654322147,0.694815838336945,
5.4));
#45052=CARTESIAN_POINT('Ctrl Pts',(-1.52131654322147,0.694815838336945,
5.37));
#45053=CARTESIAN_POINT('',(-1.59034790098667,0.639853382110596,5.4));
#45054=CARTESIAN_POINT('Ctrl Pts',(-1.59034790098667,0.639853382110596,
5.4));
#45055=CARTESIAN_POINT('Ctrl Pts',(-1.56671215593815,0.676057302951813,
5.4));
#45056=CARTESIAN_POINT('Ctrl Pts',(-1.52131654322147,0.694815838336945,
5.4));
#45057=CARTESIAN_POINT('',(-1.59034790098667,0.639853382110596,5.37));
#45058=CARTESIAN_POINT('',(-1.59034790098667,0.639853382110596,5.4));
#45059=CARTESIAN_POINT('Ctrl Pts',(-1.59034790098667,0.639853382110596,
5.37));
#45060=CARTESIAN_POINT('Ctrl Pts',(-1.56671215593815,0.676057302951813,
5.37));
#45061=CARTESIAN_POINT('Ctrl Pts',(-1.52131654322147,0.694815838336945,
5.37));
#45062=CARTESIAN_POINT('Ctrl Pts',(-1.61398364603519,0.562005484104157,
5.4));
#45063=CARTESIAN_POINT('Ctrl Pts',(-1.61398364603519,0.562005484104157,
5.37));
#45064=CARTESIAN_POINT('Ctrl Pts',(-1.61398364603519,0.603649401664734,
5.4));
#45065=CARTESIAN_POINT('Ctrl Pts',(-1.61398364603519,0.603649401664734,
5.37));
#45066=CARTESIAN_POINT('Ctrl Pts',(-1.59034790098667,0.639853382110596,
5.4));
#45067=CARTESIAN_POINT('Ctrl Pts',(-1.59034790098667,0.639853382110596,
5.37));
#45068=CARTESIAN_POINT('',(-1.61398364603519,0.562005484104157,5.4));
#45069=CARTESIAN_POINT('Ctrl Pts',(-1.61398364603519,0.562005484104157,
5.4));
#45070=CARTESIAN_POINT('Ctrl Pts',(-1.61398364603519,0.603649401664734,
5.4));
#45071=CARTESIAN_POINT('Ctrl Pts',(-1.59034790098667,0.639853382110596,
5.4));
#45072=CARTESIAN_POINT('',(-1.61398364603519,0.562005484104157,5.37));
#45073=CARTESIAN_POINT('',(-1.61398364603519,0.562005484104157,5.4));
#45074=CARTESIAN_POINT('Ctrl Pts',(-1.61398364603519,0.562005484104157,
5.37));
#45075=CARTESIAN_POINT('Ctrl Pts',(-1.61398364603519,0.603649401664734,
5.37));
#45076=CARTESIAN_POINT('Ctrl Pts',(-1.59034790098667,0.639853382110596,
5.37));
#45077=CARTESIAN_POINT('Ctrl Pts',(-1.59466232359409,0.493536853790283,
5.4));
#45078=CARTESIAN_POINT('Ctrl Pts',(-1.59466232359409,0.493536853790283,
5.37));
#45079=CARTESIAN_POINT('Ctrl Pts',(-1.61398364603519,0.524113261699677,
5.4));
#45080=CARTESIAN_POINT('Ctrl Pts',(-1.61398364603519,0.524113261699677,
5.37));
#45081=CARTESIAN_POINT('Ctrl Pts',(-1.61398364603519,0.562005484104157,
5.4));
#45082=CARTESIAN_POINT('Ctrl Pts',(-1.61398364603519,0.562005484104157,
5.37));
#45083=CARTESIAN_POINT('',(-1.59466232359409,0.493536853790283,5.4));
#45084=CARTESIAN_POINT('Ctrl Pts',(-1.59466232359409,0.493536853790283,
5.4));
#45085=CARTESIAN_POINT('Ctrl Pts',(-1.61398364603519,0.524113261699677,
5.4));
#45086=CARTESIAN_POINT('Ctrl Pts',(-1.61398364603519,0.562005484104157,
5.4));
#45087=CARTESIAN_POINT('',(-1.59466232359409,0.493536853790283,5.37));
#45088=CARTESIAN_POINT('',(-1.59466232359409,0.493536853790283,5.4));
#45089=CARTESIAN_POINT('Ctrl Pts',(-1.59466232359409,0.493536853790283,
5.37));
#45090=CARTESIAN_POINT('Ctrl Pts',(-1.61398364603519,0.524113261699677,
5.37));
#45091=CARTESIAN_POINT('Ctrl Pts',(-1.61398364603519,0.562005484104157,
5.37));
#45092=CARTESIAN_POINT('Ctrl Pts',(-1.53594817221165,0.442326062917709,
5.4));
#45093=CARTESIAN_POINT('Ctrl Pts',(-1.53594817221165,0.442326062917709,
5.37));
#45094=CARTESIAN_POINT('Ctrl Pts',(-1.57534112036228,0.46296044588089,5.4));
#45095=CARTESIAN_POINT('Ctrl Pts',(-1.57534112036228,0.46296044588089,5.37));
#45096=CARTESIAN_POINT('Ctrl Pts',(-1.59466232359409,0.493536853790283,
5.4));
#45097=CARTESIAN_POINT('Ctrl Pts',(-1.59466232359409,0.493536853790283,
5.37));
#45098=CARTESIAN_POINT('',(-1.53594817221165,0.442326062917709,5.4));
#45099=CARTESIAN_POINT('Ctrl Pts',(-1.53594817221165,0.442326062917709,
5.4));
#45100=CARTESIAN_POINT('Ctrl Pts',(-1.57534112036228,0.46296044588089,5.4));
#45101=CARTESIAN_POINT('Ctrl Pts',(-1.59466232359409,0.493536853790283,
5.4));
#45102=CARTESIAN_POINT('',(-1.53594817221165,0.442326062917709,5.37));
#45103=CARTESIAN_POINT('',(-1.53594817221165,0.442326062917709,5.4));
#45104=CARTESIAN_POINT('Ctrl Pts',(-1.53594817221165,0.442326062917709,
5.37));
#45105=CARTESIAN_POINT('Ctrl Pts',(-1.57534112036228,0.46296044588089,5.37));
#45106=CARTESIAN_POINT('Ctrl Pts',(-1.59466232359409,0.493536853790283,
5.37));
#45107=CARTESIAN_POINT('Ctrl Pts',(-1.4297748953104,0.407997959852219,5.4));
#45108=CARTESIAN_POINT('Ctrl Pts',(-1.4297748953104,0.407997959852219,5.37));
#45109=CARTESIAN_POINT('Ctrl Pts',(-1.50555934011936,0.426193737983704,
5.4));
#45110=CARTESIAN_POINT('Ctrl Pts',(-1.50555934011936,0.426193737983704,
5.37));
#45111=CARTESIAN_POINT('Ctrl Pts',(-1.53594817221165,0.442326062917709,
5.4));
#45112=CARTESIAN_POINT('Ctrl Pts',(-1.53594817221165,0.442326062917709,
5.37));
#45113=CARTESIAN_POINT('',(-1.4297748953104,0.407997959852219,5.4));
#45114=CARTESIAN_POINT('Ctrl Pts',(-1.4297748953104,0.407997959852219,5.4));
#45115=CARTESIAN_POINT('Ctrl Pts',(-1.50555934011936,0.426193737983704,
5.4));
#45116=CARTESIAN_POINT('Ctrl Pts',(-1.53594817221165,0.442326062917709,
5.4));
#45117=CARTESIAN_POINT('',(-1.4297748953104,0.407997959852219,5.37));
#45118=CARTESIAN_POINT('',(-1.4297748953104,0.407997959852219,5.4));
#45119=CARTESIAN_POINT('Ctrl Pts',(-1.4297748953104,0.407997959852219,5.37));
#45120=CARTESIAN_POINT('Ctrl Pts',(-1.50555934011936,0.426193737983704,
5.37));
#45121=CARTESIAN_POINT('Ctrl Pts',(-1.53594817221165,0.442326062917709,
5.37));
#45122=CARTESIAN_POINT('Ctrl Pts',(-1.33185543119907,0.381173276901245,
5.4));
#45123=CARTESIAN_POINT('Ctrl Pts',(-1.33185543119907,0.381173276901245,
5.37));
#45124=CARTESIAN_POINT('Ctrl Pts',(-1.35399045050144,0.389802196621895,
5.4));
#45125=CARTESIAN_POINT('Ctrl Pts',(-1.35399045050144,0.389802196621895,
5.37));
#45126=CARTESIAN_POINT('Ctrl Pts',(-1.4297748953104,0.407997959852219,5.4));
#45127=CARTESIAN_POINT('Ctrl Pts',(-1.4297748953104,0.407997959852219,5.37));
#45128=CARTESIAN_POINT('',(-1.33185543119907,0.381173276901245,5.4));
#45129=CARTESIAN_POINT('Ctrl Pts',(-1.33185543119907,0.381173276901245,
5.4));
#45130=CARTESIAN_POINT('Ctrl Pts',(-1.35399045050144,0.389802196621895,
5.4));
#45131=CARTESIAN_POINT('Ctrl Pts',(-1.4297748953104,0.407997959852219,5.4));
#45132=CARTESIAN_POINT('',(-1.33185543119907,0.381173276901245,5.37));
#45133=CARTESIAN_POINT('',(-1.33185543119907,0.381173276901245,5.4));
#45134=CARTESIAN_POINT('Ctrl Pts',(-1.33185543119907,0.381173276901245,
5.37));
#45135=CARTESIAN_POINT('Ctrl Pts',(-1.35399045050144,0.389802196621895,
5.37));
#45136=CARTESIAN_POINT('Ctrl Pts',(-1.4297748953104,0.407997959852219,5.37));
#45137=CARTESIAN_POINT('Ctrl Pts',(-1.28233291208744,0.348721021413803,
5.4));
#45138=CARTESIAN_POINT('Ctrl Pts',(-1.28233291208744,0.348721021413803,
5.37));
#45139=CARTESIAN_POINT('Ctrl Pts',(-1.29733969271183,0.368042299151421,
5.4));
#45140=CARTESIAN_POINT('Ctrl Pts',(-1.29733969271183,0.368042299151421,
5.37));
#45141=CARTESIAN_POINT('Ctrl Pts',(-1.33185543119907,0.381173276901245,
5.4));
#45142=CARTESIAN_POINT('Ctrl Pts',(-1.33185543119907,0.381173276901245,
5.37));
#45143=CARTESIAN_POINT('',(-1.28233291208744,0.348721021413803,5.4));
#45144=CARTESIAN_POINT('Ctrl Pts',(-1.28233291208744,0.348721021413803,
5.4));
#45145=CARTESIAN_POINT('Ctrl Pts',(-1.29733969271183,0.368042299151421,
5.4));
#45146=CARTESIAN_POINT('Ctrl Pts',(-1.33185543119907,0.381173276901245,
5.4));
#45147=CARTESIAN_POINT('',(-1.28233291208744,0.348721021413803,5.37));
#45148=CARTESIAN_POINT('',(-1.28233291208744,0.348721021413803,5.4));
#45149=CARTESIAN_POINT('Ctrl Pts',(-1.28233291208744,0.348721021413803,
5.37));
#45150=CARTESIAN_POINT('Ctrl Pts',(-1.29733969271183,0.368042299151421,
5.37));
#45151=CARTESIAN_POINT('Ctrl Pts',(-1.33185543119907,0.381173276901245,
5.37));
#45152=CARTESIAN_POINT('Ctrl Pts',(-1.26732613146305,0.303512969613075,
5.4));
#45153=CARTESIAN_POINT('Ctrl Pts',(-1.26732613146305,0.303512969613075,
5.37));
#45154=CARTESIAN_POINT('Ctrl Pts',(-1.26732613146305,0.329399743676186,
5.4));
#45155=CARTESIAN_POINT('Ctrl Pts',(-1.26732613146305,0.329399743676186,
5.37));
#45156=CARTESIAN_POINT('Ctrl Pts',(-1.28233291208744,0.348721021413803,
5.4));
#45157=CARTESIAN_POINT('Ctrl Pts',(-1.28233291208744,0.348721021413803,
5.37));
#45158=CARTESIAN_POINT('',(-1.26732613146305,0.303512969613075,5.4));
#45159=CARTESIAN_POINT('Ctrl Pts',(-1.26732613146305,0.303512969613075,
5.4));
#45160=CARTESIAN_POINT('Ctrl Pts',(-1.26732613146305,0.329399743676186,
5.4));
#45161=CARTESIAN_POINT('Ctrl Pts',(-1.28233291208744,0.348721021413803,
5.4));
#45162=CARTESIAN_POINT('',(-1.26732613146305,0.303512969613075,5.37));
#45163=CARTESIAN_POINT('',(-1.26732613146305,0.303512969613075,5.4));
#45164=CARTESIAN_POINT('Ctrl Pts',(-1.26732613146305,0.303512969613075,
5.37));
#45165=CARTESIAN_POINT('Ctrl Pts',(-1.26732613146305,0.329399743676186,
5.37));
#45166=CARTESIAN_POINT('Ctrl Pts',(-1.28233291208744,0.348721021413803,
5.37));
#45167=CARTESIAN_POINT('Ctrl Pts',(-1.28289557993412,0.256429070234299,
5.4));
#45168=CARTESIAN_POINT('Ctrl Pts',(-1.28289557993412,0.256429070234299,
5.37));
#45169=CARTESIAN_POINT('Ctrl Pts',(-1.26732613146305,0.278001391887665,
5.4));
#45170=CARTESIAN_POINT('Ctrl Pts',(-1.26732613146305,0.278001391887665,
5.37));
#45171=CARTESIAN_POINT('Ctrl Pts',(-1.26732613146305,0.303512969613075,
5.4));
#45172=CARTESIAN_POINT('Ctrl Pts',(-1.26732613146305,0.303512969613075,
5.37));
#45173=CARTESIAN_POINT('',(-1.28289557993412,0.256429070234299,5.4));
#45174=CARTESIAN_POINT('Ctrl Pts',(-1.28289557993412,0.256429070234299,
5.4));
#45175=CARTESIAN_POINT('Ctrl Pts',(-1.26732613146305,0.278001391887665,
5.4));
#45176=CARTESIAN_POINT('Ctrl Pts',(-1.26732613146305,0.303512969613075,
5.4));
#45177=CARTESIAN_POINT('',(-1.28289557993412,0.256429070234299,5.37));
#45178=CARTESIAN_POINT('',(-1.28289557993412,0.256429070234299,5.4));
#45179=CARTESIAN_POINT('Ctrl Pts',(-1.28289557993412,0.256429070234299,
5.37));
#45180=CARTESIAN_POINT('Ctrl Pts',(-1.26732613146305,0.278001391887665,
5.37));
#45181=CARTESIAN_POINT('Ctrl Pts',(-1.26732613146305,0.303512969613075,
5.37));
#45182=CARTESIAN_POINT('Ctrl Pts',(-1.33035470545292,0.222476148605347,
5.4));
#45183=CARTESIAN_POINT('Ctrl Pts',(-1.33035470545292,0.222476148605347,
5.37));
#45184=CARTESIAN_POINT('Ctrl Pts',(-1.29846526682377,0.234856748580933,
5.4));
#45185=CARTESIAN_POINT('Ctrl Pts',(-1.29846526682377,0.234856748580933,
5.37));
#45186=CARTESIAN_POINT('Ctrl Pts',(-1.28289557993412,0.256429070234299,
5.4));
#45187=CARTESIAN_POINT('Ctrl Pts',(-1.28289557993412,0.256429070234299,
5.37));
#45188=CARTESIAN_POINT('',(-1.33035470545292,0.222476148605347,5.4));
#45189=CARTESIAN_POINT('Ctrl Pts',(-1.33035470545292,0.222476148605347,
5.4));
#45190=CARTESIAN_POINT('Ctrl Pts',(-1.29846526682377,0.234856748580933,
5.4));
#45191=CARTESIAN_POINT('Ctrl Pts',(-1.28289557993412,0.256429070234299,
5.4));
#45192=CARTESIAN_POINT('',(-1.33035470545292,0.222476148605347,5.37));
#45193=CARTESIAN_POINT('',(-1.33035470545292,0.222476148605347,5.4));
#45194=CARTESIAN_POINT('Ctrl Pts',(-1.33035470545292,0.222476148605347,
5.37));
#45195=CARTESIAN_POINT('Ctrl Pts',(-1.29846526682377,0.234856748580933,
5.37));
#45196=CARTESIAN_POINT('Ctrl Pts',(-1.28289557993412,0.256429070234299,
5.37));
#45197=CARTESIAN_POINT('Ctrl Pts',(-1.40388812124729,0.210095518827438,
5.4));
#45198=CARTESIAN_POINT('Ctrl Pts',(-1.40388812124729,0.210095518827438,
5.37));
#45199=CARTESIAN_POINT('Ctrl Pts',(-1.36224426329136,0.210095518827438,
5.4));
#45200=CARTESIAN_POINT('Ctrl Pts',(-1.36224426329136,0.210095518827438,
5.37));
#45201=CARTESIAN_POINT('Ctrl Pts',(-1.33035470545292,0.222476148605347,
5.4));
#45202=CARTESIAN_POINT('Ctrl Pts',(-1.33035470545292,0.222476148605347,
5.37));
#45203=CARTESIAN_POINT('',(-1.40388812124729,0.210095518827438,5.4));
#45204=CARTESIAN_POINT('Ctrl Pts',(-1.40388812124729,0.210095518827438,
5.4));
#45205=CARTESIAN_POINT('Ctrl Pts',(-1.36224426329136,0.210095518827438,
5.4));
#45206=CARTESIAN_POINT('Ctrl Pts',(-1.33035470545292,0.222476148605347,
5.4));
#45207=CARTESIAN_POINT('',(-1.40388812124729,0.210095518827438,5.37));
#45208=CARTESIAN_POINT('',(-1.40388812124729,0.210095518827438,5.4));
#45209=CARTESIAN_POINT('Ctrl Pts',(-1.40388812124729,0.210095518827438,
5.37));
#45210=CARTESIAN_POINT('Ctrl Pts',(-1.36224426329136,0.210095518827438,
5.37));
#45211=CARTESIAN_POINT('Ctrl Pts',(-1.33035470545292,0.222476148605347,
5.37));
#45212=CARTESIAN_POINT('Ctrl Pts',(-1.48830153048038,0.226415419578552,
5.4));
#45213=CARTESIAN_POINT('Ctrl Pts',(-1.48830153048038,0.226415419578552,
5.37));
#45214=CARTESIAN_POINT('Ctrl Pts',(-1.45078445971012,0.210095518827438,
5.4));
#45215=CARTESIAN_POINT('Ctrl Pts',(-1.45078445971012,0.210095518827438,
5.37));
#45216=CARTESIAN_POINT('Ctrl Pts',(-1.40388812124729,0.210095518827438,
5.4));
#45217=CARTESIAN_POINT('Ctrl Pts',(-1.40388812124729,0.210095518827438,
5.37));
#45218=CARTESIAN_POINT('',(-1.48830153048038,0.226415419578552,5.4));
#45219=CARTESIAN_POINT('Ctrl Pts',(-1.48830153048038,0.226415419578552,
5.4));
#45220=CARTESIAN_POINT('Ctrl Pts',(-1.45078445971012,0.210095518827438,
5.4));
#45221=CARTESIAN_POINT('Ctrl Pts',(-1.40388812124729,0.210095518827438,
5.4));
#45222=CARTESIAN_POINT('',(-1.48830153048038,0.226415419578552,5.37));
#45223=CARTESIAN_POINT('',(-1.48830153048038,0.226415419578552,5.4));
#45224=CARTESIAN_POINT('Ctrl Pts',(-1.48830153048038,0.226415419578552,
5.37));
#45225=CARTESIAN_POINT('Ctrl Pts',(-1.45078445971012,0.210095518827438,
5.37));
#45226=CARTESIAN_POINT('Ctrl Pts',(-1.40388812124729,0.210095518827438,
5.37));
#45227=CARTESIAN_POINT('Ctrl Pts',(-1.54363919794559,0.269184851646423,
5.4));
#45228=CARTESIAN_POINT('Ctrl Pts',(-1.54363919794559,0.269184851646423,
5.37));
#45229=CARTESIAN_POINT('Ctrl Pts',(-1.52581860125065,0.242735350131989,
5.4));
#45230=CARTESIAN_POINT('Ctrl Pts',(-1.52581860125065,0.242735350131989,
5.37));
#45231=CARTESIAN_POINT('Ctrl Pts',(-1.48830153048038,0.226415419578552,
5.4));
#45232=CARTESIAN_POINT('Ctrl Pts',(-1.48830153048038,0.226415419578552,
5.37));
#45233=CARTESIAN_POINT('',(-1.54363919794559,0.269184851646423,5.4));
#45234=CARTESIAN_POINT('Ctrl Pts',(-1.54363919794559,0.269184851646423,
5.4));
#45235=CARTESIAN_POINT('Ctrl Pts',(-1.52581860125065,0.242735350131989,
5.4));
#45236=CARTESIAN_POINT('Ctrl Pts',(-1.48830153048038,0.226415419578552,
5.4));
#45237=CARTESIAN_POINT('',(-1.54363919794559,0.269184851646423,5.37));
#45238=CARTESIAN_POINT('',(-1.54363919794559,0.269184851646423,5.4));
#45239=CARTESIAN_POINT('Ctrl Pts',(-1.54363919794559,0.269184851646423,
5.37));
#45240=CARTESIAN_POINT('Ctrl Pts',(-1.52581860125065,0.242735350131989,
5.37));
#45241=CARTESIAN_POINT('Ctrl Pts',(-1.48830153048038,0.226415419578552,
5.37));
#45242=CARTESIAN_POINT('Ctrl Pts',(-1.56633700430393,0.336903148889542,
5.4));
#45243=CARTESIAN_POINT('Ctrl Pts',(-1.56633700430393,0.336903148889542,
5.37));
#45244=CARTESIAN_POINT('Ctrl Pts',(-1.56145979464054,0.295634382963181,
5.4));
#45245=CARTESIAN_POINT('Ctrl Pts',(-1.56145979464054,0.295634382963181,
5.37));
#45246=CARTESIAN_POINT('Ctrl Pts',(-1.54363919794559,0.269184851646423,
5.4));
#45247=CARTESIAN_POINT('Ctrl Pts',(-1.54363919794559,0.269184851646423,
5.37));
#45248=CARTESIAN_POINT('',(-1.56633700430393,0.336903148889542,5.4));
#45249=CARTESIAN_POINT('Ctrl Pts',(-1.56633700430393,0.336903148889542,
5.4));
#45250=CARTESIAN_POINT('Ctrl Pts',(-1.56145979464054,0.295634382963181,
5.4));
#45251=CARTESIAN_POINT('Ctrl Pts',(-1.54363919794559,0.269184851646423,
5.4));
#45252=CARTESIAN_POINT('',(-1.56633700430393,0.336903148889542,5.37));
#45253=CARTESIAN_POINT('',(-1.56633700430393,0.336903148889542,5.4));
#45254=CARTESIAN_POINT('Ctrl Pts',(-1.56633700430393,0.336903148889542,
5.37));
#45255=CARTESIAN_POINT('Ctrl Pts',(-1.56145979464054,0.295634382963181,
5.37));
#45256=CARTESIAN_POINT('Ctrl Pts',(-1.54363919794559,0.269184851646423,
5.37));
#45257=CARTESIAN_POINT('Origin',(-1.63499321043491,0.330900424718857,5.4));
#45258=CARTESIAN_POINT('',(-1.63499321043491,0.330900424718857,5.4));
#45259=CARTESIAN_POINT('',(-0.838054220366137,0.400578101477175,5.4));
#45260=CARTESIAN_POINT('',(-1.63499321043491,0.330900424718857,5.37));
#45261=CARTESIAN_POINT('',(-1.63499321043491,0.330900424718857,5.4));
#45262=CARTESIAN_POINT('',(-1.63499321043491,0.330900424718857,5.37));
#45263=CARTESIAN_POINT('Ctrl Pts',(-1.60479201376438,0.232042992115021,
5.4));
#45264=CARTESIAN_POINT('Ctrl Pts',(-1.60479201376438,0.232042992115021,
5.37));
#45265=CARTESIAN_POINT('Ctrl Pts',(-1.63349248468876,0.275750362873077,
5.4));
#45266=CARTESIAN_POINT('Ctrl Pts',(-1.63349248468876,0.275750362873077,
5.37));
#45267=CARTESIAN_POINT('Ctrl Pts',(-1.63499321043491,0.330900424718857,
5.4));
#45268=CARTESIAN_POINT('Ctrl Pts',(-1.63499321043491,0.330900424718857,
5.37));
#45269=CARTESIAN_POINT('',(-1.60479201376438,0.232042992115021,5.4));
#45270=CARTESIAN_POINT('Ctrl Pts',(-1.60479201376438,0.232042992115021,
5.4));
#45271=CARTESIAN_POINT('Ctrl Pts',(-1.63349248468876,0.275750362873077,
5.4));
#45272=CARTESIAN_POINT('Ctrl Pts',(-1.63499321043491,0.330900424718857,
5.4));
#45273=CARTESIAN_POINT('',(-1.60479201376438,0.232042992115021,5.37));
#45274=CARTESIAN_POINT('',(-1.60479201376438,0.232042992115021,5.4));
#45275=CARTESIAN_POINT('Ctrl Pts',(-1.60479201376438,0.232042992115021,
5.37));
#45276=CARTESIAN_POINT('Ctrl Pts',(-1.63349248468876,0.275750362873077,
5.37));
#45277=CARTESIAN_POINT('Ctrl Pts',(-1.63499321043491,0.330900424718857,
5.37));
#45278=CARTESIAN_POINT('Ctrl Pts',(-1.5256309658289,0.16657572388649,5.4));
#45279=CARTESIAN_POINT('Ctrl Pts',(-1.5256309658289,0.16657572388649,5.37));
#45280=CARTESIAN_POINT('Ctrl Pts',(-1.57609142363071,0.188335621356964,
5.4));
#45281=CARTESIAN_POINT('Ctrl Pts',(-1.57609142363071,0.188335621356964,
5.37));
#45282=CARTESIAN_POINT('Ctrl Pts',(-1.60479201376438,0.232042992115021,
5.4));
#45283=CARTESIAN_POINT('Ctrl Pts',(-1.60479201376438,0.232042992115021,
5.37));
#45284=CARTESIAN_POINT('Ctrl Pts',(-1.5256309658289,0.16657572388649,5.4));
#45285=CARTESIAN_POINT('Ctrl Pts',(-1.57609142363071,0.188335621356964,
5.4));
#45286=CARTESIAN_POINT('Ctrl Pts',(-1.60479201376438,0.232042992115021,
5.4));
#45287=CARTESIAN_POINT('Ctrl Pts',(-1.5256309658289,0.16657572388649,5.37));
#45288=CARTESIAN_POINT('Ctrl Pts',(-1.57609142363071,0.188335621356964,
5.37));
#45289=CARTESIAN_POINT('Ctrl Pts',(-1.60479201376438,0.232042992115021,
5.37));
#45290=CARTESIAN_POINT('Origin',(-1.41608120501041,0.429195100069046,5.37));
#45291=CARTESIAN_POINT('Ctrl Pts',(-0.561255231499672,0.194525921344757,
5.4));
#45292=CARTESIAN_POINT('Ctrl Pts',(-0.561255231499672,0.194525921344757,
5.37));
#45293=CARTESIAN_POINT('Ctrl Pts',(-0.613779082894325,0.144440674781799,
5.4));
#45294=CARTESIAN_POINT('Ctrl Pts',(-0.613779082894325,0.144440674781799,
5.37));
#45295=CARTESIAN_POINT('Ctrl Pts',(-0.69406558573246,0.144440674781799,
5.4));
#45296=CARTESIAN_POINT('Ctrl Pts',(-0.69406558573246,0.144440674781799,
5.37));
#45297=CARTESIAN_POINT('',(-0.561255231499672,0.194525921344757,5.4));
#45298=CARTESIAN_POINT('',(-0.69406558573246,0.144440674781799,5.4));
#45299=CARTESIAN_POINT('Ctrl Pts',(-0.561255231499672,0.194525921344757,
5.4));
#45300=CARTESIAN_POINT('Ctrl Pts',(-0.613779082894325,0.144440674781799,
5.4));
#45301=CARTESIAN_POINT('Ctrl Pts',(-0.69406558573246,0.144440674781799,
5.4));
#45302=CARTESIAN_POINT('',(-0.561255231499672,0.194525921344757,5.37));
#45303=CARTESIAN_POINT('',(-0.561255231499672,0.194525921344757,5.4));
#45304=CARTESIAN_POINT('',(-0.69406558573246,0.144440674781799,5.37));
#45305=CARTESIAN_POINT('Ctrl Pts',(-0.561255231499672,0.194525921344757,
5.37));
#45306=CARTESIAN_POINT('Ctrl Pts',(-0.613779082894325,0.144440674781799,
5.37));
#45307=CARTESIAN_POINT('Ctrl Pts',(-0.69406558573246,0.144440674781799,
5.37));
#45308=CARTESIAN_POINT('',(-0.69406558573246,0.144440674781799,5.4));
#45309=CARTESIAN_POINT('Ctrl Pts',(-0.508731380105019,0.316643932461739,
5.4));
#45310=CARTESIAN_POINT('Ctrl Pts',(-0.508731380105019,0.316643932461739,
5.37));
#45311=CARTESIAN_POINT('Ctrl Pts',(-0.508731380105019,0.244611197710037,
5.4));
#45312=CARTESIAN_POINT('Ctrl Pts',(-0.508731380105019,0.244611197710037,
5.37));
#45313=CARTESIAN_POINT('Ctrl Pts',(-0.561255231499672,0.194525921344757,
5.4));
#45314=CARTESIAN_POINT('Ctrl Pts',(-0.561255231499672,0.194525921344757,
5.37));
#45315=CARTESIAN_POINT('',(-0.508731380105019,0.316643932461739,5.4));
#45316=CARTESIAN_POINT('Ctrl Pts',(-0.508731380105019,0.316643932461739,
5.4));
#45317=CARTESIAN_POINT('Ctrl Pts',(-0.508731380105019,0.244611197710037,
5.4));
#45318=CARTESIAN_POINT('Ctrl Pts',(-0.561255231499672,0.194525921344757,
5.4));
#45319=CARTESIAN_POINT('',(-0.508731380105019,0.316643932461739,5.37));
#45320=CARTESIAN_POINT('',(-0.508731380105019,0.316643932461739,5.4));
#45321=CARTESIAN_POINT('Ctrl Pts',(-0.508731380105019,0.316643932461739,
5.37));
#45322=CARTESIAN_POINT('Ctrl Pts',(-0.508731380105019,0.244611197710037,
5.37));
#45323=CARTESIAN_POINT('Ctrl Pts',(-0.561255231499672,0.194525921344757,
5.37));
#45324=CARTESIAN_POINT('Ctrl Pts',(-0.535743728280067,0.405371749401093,
5.4));
#45325=CARTESIAN_POINT('Ctrl Pts',(-0.535743728280067,0.405371749401093,
5.37));
#45326=CARTESIAN_POINT('Ctrl Pts',(-0.508731380105019,0.369918146729469,
5.4));
#45327=CARTESIAN_POINT('Ctrl Pts',(-0.508731380105019,0.369918146729469,
5.37));
#45328=CARTESIAN_POINT('Ctrl Pts',(-0.508731380105019,0.316643932461739,
5.4));
#45329=CARTESIAN_POINT('Ctrl Pts',(-0.508731380105019,0.316643932461739,
5.37));
#45330=CARTESIAN_POINT('',(-0.535743728280067,0.405371749401093,5.4));
#45331=CARTESIAN_POINT('Ctrl Pts',(-0.535743728280067,0.405371749401093,
5.4));
#45332=CARTESIAN_POINT('Ctrl Pts',(-0.508731380105019,0.369918146729469,
5.4));
#45333=CARTESIAN_POINT('Ctrl Pts',(-0.508731380105019,0.316643932461739,
5.4));
#45334=CARTESIAN_POINT('',(-0.535743728280067,0.405371749401093,5.37));
#45335=CARTESIAN_POINT('',(-0.535743728280067,0.405371749401093,5.4));
#45336=CARTESIAN_POINT('Ctrl Pts',(-0.535743728280067,0.405371749401093,
5.37));
#45337=CARTESIAN_POINT('Ctrl Pts',(-0.508731380105019,0.369918146729469,
5.37));
#45338=CARTESIAN_POINT('Ctrl Pts',(-0.508731380105019,0.316643932461739,
5.37));
#45339=CARTESIAN_POINT('Ctrl Pts',(-0.611528173089027,0.452080512046814,
5.4));
#45340=CARTESIAN_POINT('Ctrl Pts',(-0.611528173089027,0.452080512046814,
5.37));
#45341=CARTESIAN_POINT('Ctrl Pts',(-0.562755838036537,0.440825366973877,
5.4));
#45342=CARTESIAN_POINT('Ctrl Pts',(-0.562755838036537,0.440825366973877,
5.37));
#45343=CARTESIAN_POINT('Ctrl Pts',(-0.535743728280067,0.405371749401093,
5.4));
#45344=CARTESIAN_POINT('Ctrl Pts',(-0.535743728280067,0.405371749401093,
5.37));
#45345=CARTESIAN_POINT('',(-0.611528173089027,0.452080512046814,5.4));
#45346=CARTESIAN_POINT('Ctrl Pts',(-0.611528173089027,0.452080512046814,
5.4));
#45347=CARTESIAN_POINT('Ctrl Pts',(-0.562755838036537,0.440825366973877,
5.4));
#45348=CARTESIAN_POINT('Ctrl Pts',(-0.535743728280067,0.405371749401093,
5.4));
#45349=CARTESIAN_POINT('',(-0.611528173089027,0.452080512046814,5.37));
#45350=CARTESIAN_POINT('',(-0.611528173089027,0.452080512046814,5.4));
#45351=CARTESIAN_POINT('Ctrl Pts',(-0.611528173089027,0.452080512046814,
5.37));
#45352=CARTESIAN_POINT('Ctrl Pts',(-0.562755838036537,0.440825366973877,
5.37));
#45353=CARTESIAN_POINT('Ctrl Pts',(-0.535743728280067,0.405371749401093,
5.37));
#45354=CARTESIAN_POINT('Ctrl Pts',(-0.554877296090126,0.498601639270782,
5.4));
#45355=CARTESIAN_POINT('Ctrl Pts',(-0.554877296090126,0.498601639270782,
5.37));
#45356=CARTESIAN_POINT('Ctrl Pts',(-0.574011102318764,0.469338321685791,
5.4));
#45357=CARTESIAN_POINT('Ctrl Pts',(-0.574011102318764,0.469338321685791,
5.37));
#45358=CARTESIAN_POINT('Ctrl Pts',(-0.611528173089027,0.452080512046814,
5.4));
#45359=CARTESIAN_POINT('Ctrl Pts',(-0.611528173089027,0.452080512046814,
5.37));
#45360=CARTESIAN_POINT('',(-0.554877296090126,0.498601639270782,5.4));
#45361=CARTESIAN_POINT('Ctrl Pts',(-0.554877296090126,0.498601639270782,
5.4));
#45362=CARTESIAN_POINT('Ctrl Pts',(-0.574011102318764,0.469338321685791,
5.4));
#45363=CARTESIAN_POINT('Ctrl Pts',(-0.611528173089027,0.452080512046814,
5.4));
#45364=CARTESIAN_POINT('',(-0.554877296090126,0.498601639270782,5.37));
#45365=CARTESIAN_POINT('',(-0.554877296090126,0.498601639270782,5.4));
#45366=CARTESIAN_POINT('Ctrl Pts',(-0.554877296090126,0.498601639270782,
5.37));
#45367=CARTESIAN_POINT('Ctrl Pts',(-0.574011102318764,0.469338321685791,
5.37));
#45368=CARTESIAN_POINT('Ctrl Pts',(-0.611528173089027,0.452080512046814,
5.37));
#45369=CARTESIAN_POINT('Ctrl Pts',(-0.535743728280067,0.563506150245667,
5.4));
#45370=CARTESIAN_POINT('Ctrl Pts',(-0.535743728280067,0.563506150245667,
5.37));
#45371=CARTESIAN_POINT('Ctrl Pts',(-0.535743728280067,0.527864956855774,
5.4));
#45372=CARTESIAN_POINT('Ctrl Pts',(-0.535743728280067,0.527864956855774,
5.37));
#45373=CARTESIAN_POINT('Ctrl Pts',(-0.554877296090126,0.498601639270782,
5.4));
#45374=CARTESIAN_POINT('Ctrl Pts',(-0.554877296090126,0.498601639270782,
5.37));
#45375=CARTESIAN_POINT('',(-0.535743728280067,0.563506150245667,5.4));
#45376=CARTESIAN_POINT('Ctrl Pts',(-0.535743728280067,0.563506150245667,
5.4));
#45377=CARTESIAN_POINT('Ctrl Pts',(-0.535743728280067,0.527864956855774,
5.4));
#45378=CARTESIAN_POINT('Ctrl Pts',(-0.554877296090126,0.498601639270782,
5.4));
#45379=CARTESIAN_POINT('',(-0.535743728280067,0.563506150245667,5.37));
#45380=CARTESIAN_POINT('',(-0.535743728280067,0.563506150245667,5.4));
#45381=CARTESIAN_POINT('Ctrl Pts',(-0.535743728280067,0.563506150245667,
5.37));
#45382=CARTESIAN_POINT('Ctrl Pts',(-0.535743728280067,0.527864956855774,
5.37));
#45383=CARTESIAN_POINT('Ctrl Pts',(-0.554877296090126,0.498601639270782,
5.37));
#45384=CARTESIAN_POINT('Ctrl Pts',(-0.555815234780312,0.634413385391235,
5.4));
#45385=CARTESIAN_POINT('Ctrl Pts',(-0.555815234780312,0.634413385391235,
5.37));
#45386=CARTESIAN_POINT('Ctrl Pts',(-0.535743728280067,0.601023161411285,
5.4));
#45387=CARTESIAN_POINT('Ctrl Pts',(-0.535743728280067,0.601023161411285,
5.37));
#45388=CARTESIAN_POINT('Ctrl Pts',(-0.535743728280067,0.563506150245667,
5.4));
#45389=CARTESIAN_POINT('Ctrl Pts',(-0.535743728280067,0.563506150245667,
5.37));
#45390=CARTESIAN_POINT('',(-0.555815234780312,0.634413385391235,5.4));
#45391=CARTESIAN_POINT('Ctrl Pts',(-0.555815234780312,0.634413385391235,
5.4));
#45392=CARTESIAN_POINT('Ctrl Pts',(-0.535743728280067,0.601023161411285,
5.4));
#45393=CARTESIAN_POINT('Ctrl Pts',(-0.535743728280067,0.563506150245667,
5.4));
#45394=CARTESIAN_POINT('',(-0.555815234780312,0.634413385391235,5.37));
#45395=CARTESIAN_POINT('',(-0.555815234780312,0.634413385391235,5.4));
#45396=CARTESIAN_POINT('Ctrl Pts',(-0.555815234780312,0.634413385391235,
5.37));
#45397=CARTESIAN_POINT('Ctrl Pts',(-0.535743728280067,0.601023161411285,
5.37));
#45398=CARTESIAN_POINT('Ctrl Pts',(-0.535743728280067,0.563506150245667,
5.37));
#45399=CARTESIAN_POINT('Ctrl Pts',(-0.613779082894325,0.687124812602997,
5.4));
#45400=CARTESIAN_POINT('Ctrl Pts',(-0.613779082894325,0.687124812602997,
5.37));
#45401=CARTESIAN_POINT('Ctrl Pts',(-0.575886741280556,0.667803549766541,
5.4));
#45402=CARTESIAN_POINT('Ctrl Pts',(-0.575886741280556,0.667803549766541,
5.37));
#45403=CARTESIAN_POINT('Ctrl Pts',(-0.555815234780312,0.634413385391235,
5.4));
#45404=CARTESIAN_POINT('Ctrl Pts',(-0.555815234780312,0.634413385391235,
5.37));
#45405=CARTESIAN_POINT('',(-0.613779082894325,0.687124812602997,5.4));
#45406=CARTESIAN_POINT('Ctrl Pts',(-0.613779082894325,0.687124812602997,
5.4));
#45407=CARTESIAN_POINT('Ctrl Pts',(-0.575886741280556,0.667803549766541,
5.4));
#45408=CARTESIAN_POINT('Ctrl Pts',(-0.555815234780312,0.634413385391235,
5.4));
#45409=CARTESIAN_POINT('',(-0.613779082894325,0.687124812602997,5.37));
#45410=CARTESIAN_POINT('',(-0.613779082894325,0.687124812602997,5.4));
#45411=CARTESIAN_POINT('Ctrl Pts',(-0.613779082894325,0.687124812602997,
5.37));
#45412=CARTESIAN_POINT('Ctrl Pts',(-0.575886741280556,0.667803549766541,
5.37));
#45413=CARTESIAN_POINT('Ctrl Pts',(-0.555815234780312,0.634413385391235,
5.37));
#45414=CARTESIAN_POINT('Ctrl Pts',(-0.696691766381264,0.706446135044098,
5.4));
#45415=CARTESIAN_POINT('Ctrl Pts',(-0.696691766381264,0.706446135044098,
5.37));
#45416=CARTESIAN_POINT('Ctrl Pts',(-0.651671424508095,0.706446135044098,
5.4));
#45417=CARTESIAN_POINT('Ctrl Pts',(-0.651671424508095,0.706446135044098,
5.37));
#45418=CARTESIAN_POINT('Ctrl Pts',(-0.613779082894325,0.687124812602997,
5.4));
#45419=CARTESIAN_POINT('Ctrl Pts',(-0.613779082894325,0.687124812602997,
5.37));
#45420=CARTESIAN_POINT('',(-0.696691766381264,0.706446135044098,5.4));
#45421=CARTESIAN_POINT('Ctrl Pts',(-0.696691766381264,0.706446135044098,
5.4));
#45422=CARTESIAN_POINT('Ctrl Pts',(-0.651671424508095,0.706446135044098,
5.4));
#45423=CARTESIAN_POINT('Ctrl Pts',(-0.613779082894325,0.687124812602997,
5.4));
#45424=CARTESIAN_POINT('',(-0.696691766381264,0.706446135044098,5.37));
#45425=CARTESIAN_POINT('',(-0.696691766381264,0.706446135044098,5.4));
#45426=CARTESIAN_POINT('Ctrl Pts',(-0.696691766381264,0.706446135044098,
5.37));
#45427=CARTESIAN_POINT('Ctrl Pts',(-0.651671424508095,0.706446135044098,
5.37));
#45428=CARTESIAN_POINT('Ctrl Pts',(-0.613779082894325,0.687124812602997,
5.37));
#45429=CARTESIAN_POINT('Ctrl Pts',(-0.805866494774818,0.669116640090942,
5.4));
#45430=CARTESIAN_POINT('Ctrl Pts',(-0.805866494774818,0.669116640090942,
5.37));
#45431=CARTESIAN_POINT('Ctrl Pts',(-0.761971488595009,0.706446135044098,
5.4));
#45432=CARTESIAN_POINT('Ctrl Pts',(-0.761971488595009,0.706446135044098,
5.37));
#45433=CARTESIAN_POINT('Ctrl Pts',(-0.696691766381264,0.706446135044098,
5.4));
#45434=CARTESIAN_POINT('Ctrl Pts',(-0.696691766381264,0.706446135044098,
5.37));
#45435=CARTESIAN_POINT('',(-0.805866494774818,0.669116640090942,5.4));
#45436=CARTESIAN_POINT('Ctrl Pts',(-0.805866494774818,0.669116640090942,
5.4));
#45437=CARTESIAN_POINT('Ctrl Pts',(-0.761971488595009,0.706446135044098,
5.4));
#45438=CARTESIAN_POINT('Ctrl Pts',(-0.696691766381264,0.706446135044098,
5.4));
#45439=CARTESIAN_POINT('',(-0.805866494774818,0.669116640090942,5.37));
#45440=CARTESIAN_POINT('',(-0.805866494774818,0.669116640090942,5.4));
#45441=CARTESIAN_POINT('Ctrl Pts',(-0.805866494774818,0.669116640090942,
5.37));
#45442=CARTESIAN_POINT('Ctrl Pts',(-0.761971488595009,0.706446135044098,
5.37));
#45443=CARTESIAN_POINT('Ctrl Pts',(-0.696691766381264,0.706446135044098,
5.37));
#45444=CARTESIAN_POINT('Ctrl Pts',(-0.862142100930214,0.563881301879883,
5.4));
#45445=CARTESIAN_POINT('Ctrl Pts',(-0.862142100930214,0.563881301879883,
5.37));
#45446=CARTESIAN_POINT('Ctrl Pts',(-0.849761500954628,0.631787145137787,
5.4));
#45447=CARTESIAN_POINT('Ctrl Pts',(-0.849761500954628,0.631787145137787,
5.37));
#45448=CARTESIAN_POINT('Ctrl Pts',(-0.805866494774818,0.669116640090942,
5.4));
#45449=CARTESIAN_POINT('Ctrl Pts',(-0.805866494774818,0.669116640090942,
5.37));
#45450=CARTESIAN_POINT('',(-0.862142100930214,0.563881301879883,5.4));
#45451=CARTESIAN_POINT('Ctrl Pts',(-0.862142100930214,0.563881301879883,
5.4));
#45452=CARTESIAN_POINT('Ctrl Pts',(-0.849761500954628,0.631787145137787,
5.4));
#45453=CARTESIAN_POINT('Ctrl Pts',(-0.805866494774818,0.669116640090942,
5.4));
#45454=CARTESIAN_POINT('',(-0.862142100930214,0.563881301879883,5.37));
#45455=CARTESIAN_POINT('',(-0.862142100930214,0.563881301879883,5.4));
#45456=CARTESIAN_POINT('Ctrl Pts',(-0.862142100930214,0.563881301879883,
5.37));
#45457=CARTESIAN_POINT('Ctrl Pts',(-0.849761500954628,0.631787145137787,
5.37));
#45458=CARTESIAN_POINT('Ctrl Pts',(-0.805866494774818,0.669116640090942,
5.37));
#45459=CARTESIAN_POINT('Origin',(-0.794611230492592,0.551875853538513,5.4));
#45460=CARTESIAN_POINT('',(-0.794611230492592,0.551875853538513,5.4));
#45461=CARTESIAN_POINT('',(-0.361925074901606,0.474954124922981,5.4));
#45462=CARTESIAN_POINT('',(-0.794611230492592,0.551875853538513,5.37));
#45463=CARTESIAN_POINT('',(-0.794611230492592,0.551875853538513,5.4));
#45464=CARTESIAN_POINT('',(-0.794611230492592,0.551875853538513,5.37));
#45465=CARTESIAN_POINT('Ctrl Pts',(-0.76084591448307,0.626159632205963,
5.4));
#45466=CARTESIAN_POINT('Ctrl Pts',(-0.76084591448307,0.626159632205963,
5.37));
#45467=CARTESIAN_POINT('Ctrl Pts',(-0.787107959389687,0.601398372650147,
5.4));
#45468=CARTESIAN_POINT('Ctrl Pts',(-0.787107959389687,0.601398372650147,
5.37));
#45469=CARTESIAN_POINT('Ctrl Pts',(-0.794611230492592,0.551875853538513,
5.4));
#45470=CARTESIAN_POINT('Ctrl Pts',(-0.794611230492592,0.551875853538513,
5.37));
#45471=CARTESIAN_POINT('',(-0.76084591448307,0.626159632205963,5.4));
#45472=CARTESIAN_POINT('Ctrl Pts',(-0.76084591448307,0.626159632205963,
5.4));
#45473=CARTESIAN_POINT('Ctrl Pts',(-0.787107959389687,0.601398372650147,
5.4));
#45474=CARTESIAN_POINT('Ctrl Pts',(-0.794611230492592,0.551875853538513,
5.4));
#45475=CARTESIAN_POINT('',(-0.76084591448307,0.626159632205963,5.37));
#45476=CARTESIAN_POINT('',(-0.76084591448307,0.626159632205963,5.4));
#45477=CARTESIAN_POINT('Ctrl Pts',(-0.76084591448307,0.626159632205963,
5.37));
#45478=CARTESIAN_POINT('Ctrl Pts',(-0.787107959389687,0.601398372650147,
5.37));
#45479=CARTESIAN_POINT('Ctrl Pts',(-0.794611230492592,0.551875853538513,
5.37));
#45480=CARTESIAN_POINT('Ctrl Pts',(-0.695191159844398,0.65092089176178,
5.4));
#45481=CARTESIAN_POINT('Ctrl Pts',(-0.695191159844398,0.65092089176178,
5.37));
#45482=CARTESIAN_POINT('Ctrl Pts',(-0.734584107995033,0.65092089176178,
5.4));
#45483=CARTESIAN_POINT('Ctrl Pts',(-0.734584107995033,0.65092089176178,
5.37));
#45484=CARTESIAN_POINT('Ctrl Pts',(-0.76084591448307,0.626159632205963,
5.4));
#45485=CARTESIAN_POINT('Ctrl Pts',(-0.76084591448307,0.626159632205963,
5.37));
#45486=CARTESIAN_POINT('',(-0.695191159844398,0.65092089176178,5.4));
#45487=CARTESIAN_POINT('Ctrl Pts',(-0.695191159844398,0.65092089176178,
5.4));
#45488=CARTESIAN_POINT('Ctrl Pts',(-0.734584107995033,0.65092089176178,
5.4));
#45489=CARTESIAN_POINT('Ctrl Pts',(-0.76084591448307,0.626159632205963,
5.4));
#45490=CARTESIAN_POINT('',(-0.695191159844398,0.65092089176178,5.37));
#45491=CARTESIAN_POINT('',(-0.695191159844398,0.65092089176178,5.4));
#45492=CARTESIAN_POINT('Ctrl Pts',(-0.695191159844398,0.65092089176178,
5.37));
#45493=CARTESIAN_POINT('Ctrl Pts',(-0.734584107995033,0.65092089176178,
5.37));
#45494=CARTESIAN_POINT('Ctrl Pts',(-0.76084591448307,0.626159632205963,
5.37));
#45495=CARTESIAN_POINT('Ctrl Pts',(-0.630286708474159,0.626534783840179,
5.4));
#45496=CARTESIAN_POINT('Ctrl Pts',(-0.630286708474159,0.626534783840179,
5.37));
#45497=CARTESIAN_POINT('Ctrl Pts',(-0.655422940850258,0.65092089176178,
5.4));
#45498=CARTESIAN_POINT('Ctrl Pts',(-0.655422940850258,0.65092089176178,
5.37));
#45499=CARTESIAN_POINT('Ctrl Pts',(-0.695191159844398,0.65092089176178,
5.4));
#45500=CARTESIAN_POINT('Ctrl Pts',(-0.695191159844398,0.65092089176178,
5.37));
#45501=CARTESIAN_POINT('',(-0.630286708474159,0.626534783840179,5.4));
#45502=CARTESIAN_POINT('Ctrl Pts',(-0.630286708474159,0.626534783840179,
5.4));
#45503=CARTESIAN_POINT('Ctrl Pts',(-0.655422940850258,0.65092089176178,
5.4));
#45504=CARTESIAN_POINT('Ctrl Pts',(-0.695191159844398,0.65092089176178,
5.4));
#45505=CARTESIAN_POINT('',(-0.630286708474159,0.626534783840179,5.37));
#45506=CARTESIAN_POINT('',(-0.630286708474159,0.626534783840179,5.4));
#45507=CARTESIAN_POINT('Ctrl Pts',(-0.630286708474159,0.626534783840179,
5.37));
#45508=CARTESIAN_POINT('Ctrl Pts',(-0.655422940850258,0.65092089176178,
5.37));
#45509=CARTESIAN_POINT('Ctrl Pts',(-0.695191159844398,0.65092089176178,
5.37));
#45510=CARTESIAN_POINT('Ctrl Pts',(-0.605150237679482,0.565006816387177,
5.4));
#45511=CARTESIAN_POINT('Ctrl Pts',(-0.605150237679482,0.565006816387177,
5.37));
#45512=CARTESIAN_POINT('Ctrl Pts',(-0.605150237679482,0.602148675918579,
5.4));
#45513=CARTESIAN_POINT('Ctrl Pts',(-0.605150237679482,0.602148675918579,
5.37));
#45514=CARTESIAN_POINT('Ctrl Pts',(-0.630286708474159,0.626534783840179,
5.4));
#45515=CARTESIAN_POINT('Ctrl Pts',(-0.630286708474159,0.626534783840179,
5.37));
#45516=CARTESIAN_POINT('',(-0.605150237679482,0.565006816387177,5.4));
#45517=CARTESIAN_POINT('Ctrl Pts',(-0.605150237679482,0.565006816387177,
5.4));
#45518=CARTESIAN_POINT('Ctrl Pts',(-0.605150237679482,0.602148675918579,
5.4));
#45519=CARTESIAN_POINT('Ctrl Pts',(-0.630286708474159,0.626534783840179,
5.4));
#45520=CARTESIAN_POINT('',(-0.605150237679482,0.565006816387177,5.37));
#45521=CARTESIAN_POINT('',(-0.605150237679482,0.565006816387177,5.4));
#45522=CARTESIAN_POINT('Ctrl Pts',(-0.605150237679482,0.565006816387177,
5.37));
#45523=CARTESIAN_POINT('Ctrl Pts',(-0.605150237679482,0.602148675918579,
5.37));
#45524=CARTESIAN_POINT('Ctrl Pts',(-0.630286708474159,0.626534783840179,
5.37));
#45525=CARTESIAN_POINT('Ctrl Pts',(-0.639665856957436,0.495600247383118,
5.4));
#45526=CARTESIAN_POINT('Ctrl Pts',(-0.639665856957436,0.495600247383118,
5.37));
#45527=CARTESIAN_POINT('Ctrl Pts',(-0.605150237679482,0.518110477924347,
5.4));
#45528=CARTESIAN_POINT('Ctrl Pts',(-0.605150237679482,0.518110477924347,
5.37));
#45529=CARTESIAN_POINT('Ctrl Pts',(-0.605150237679482,0.565006816387177,
5.4));
#45530=CARTESIAN_POINT('Ctrl Pts',(-0.605150237679482,0.565006816387177,
5.37));
#45531=CARTESIAN_POINT('',(-0.639665856957436,0.495600247383118,5.4));
#45532=CARTESIAN_POINT('Ctrl Pts',(-0.639665856957436,0.495600247383118,
5.4));
#45533=CARTESIAN_POINT('Ctrl Pts',(-0.605150237679482,0.518110477924347,
5.4));
#45534=CARTESIAN_POINT('Ctrl Pts',(-0.605150237679482,0.565006816387177,
5.4));
#45535=CARTESIAN_POINT('',(-0.639665856957436,0.495600247383118,5.37));
#45536=CARTESIAN_POINT('',(-0.639665856957436,0.495600247383118,5.4));
#45537=CARTESIAN_POINT('Ctrl Pts',(-0.639665856957436,0.495600247383118,
5.37));
#45538=CARTESIAN_POINT('Ctrl Pts',(-0.605150237679482,0.518110477924347,
5.37));
#45539=CARTESIAN_POINT('Ctrl Pts',(-0.605150237679482,0.565006816387177,
5.37));
#45540=CARTESIAN_POINT('Ctrl Pts',(-0.717326179146767,0.473090016841888,
5.4));
#45541=CARTESIAN_POINT('Ctrl Pts',(-0.717326179146767,0.473090016841888,
5.37));
#45542=CARTESIAN_POINT('Ctrl Pts',(-0.67418147623539,0.473090016841888,
5.4));
#45543=CARTESIAN_POINT('Ctrl Pts',(-0.67418147623539,0.473090016841888,
5.37));
#45544=CARTESIAN_POINT('Ctrl Pts',(-0.639665856957436,0.495600247383118,
5.4));
#45545=CARTESIAN_POINT('Ctrl Pts',(-0.639665856957436,0.495600247383118,
5.37));
#45546=CARTESIAN_POINT('',(-0.717326179146767,0.473090016841888,5.4));
#45547=CARTESIAN_POINT('Ctrl Pts',(-0.717326179146767,0.473090016841888,
5.4));
#45548=CARTESIAN_POINT('Ctrl Pts',(-0.67418147623539,0.473090016841888,
5.4));
#45549=CARTESIAN_POINT('Ctrl Pts',(-0.639665856957436,0.495600247383118,
5.4));
#45550=CARTESIAN_POINT('',(-0.717326179146767,0.473090016841888,5.37));
#45551=CARTESIAN_POINT('',(-0.717326179146767,0.473090016841888,5.4));
#45552=CARTESIAN_POINT('Ctrl Pts',(-0.717326179146767,0.473090016841888,
5.37));
#45553=CARTESIAN_POINT('Ctrl Pts',(-0.67418147623539,0.473090016841888,
5.37));
#45554=CARTESIAN_POINT('Ctrl Pts',(-0.639665856957436,0.495600247383118,
5.37));
#45555=CARTESIAN_POINT('Ctrl Pts',(-0.728206172585487,0.473840379714966,
5.4));
#45556=CARTESIAN_POINT('Ctrl Pts',(-0.728206172585487,0.473840379714966,
5.37));
#45557=CARTESIAN_POINT('Ctrl Pts',(-0.721452966332436,0.473090016841888,
5.4));
#45558=CARTESIAN_POINT('Ctrl Pts',(-0.721452966332436,0.473090016841888,
5.37));
#45559=CARTESIAN_POINT('Ctrl Pts',(-0.717326179146767,0.473090016841888,
5.4));
#45560=CARTESIAN_POINT('Ctrl Pts',(-0.717326179146767,0.473090016841888,
5.37));
#45561=CARTESIAN_POINT('',(-0.728206172585487,0.473840379714966,5.4));
#45562=CARTESIAN_POINT('Ctrl Pts',(-0.728206172585487,0.473840379714966,
5.4));
#45563=CARTESIAN_POINT('Ctrl Pts',(-0.721452966332436,0.473090016841888,
5.4));
#45564=CARTESIAN_POINT('Ctrl Pts',(-0.717326179146767,0.473090016841888,
5.4));
#45565=CARTESIAN_POINT('',(-0.728206172585487,0.473840379714966,5.37));
#45566=CARTESIAN_POINT('',(-0.728206172585487,0.473840379714966,5.4));
#45567=CARTESIAN_POINT('Ctrl Pts',(-0.728206172585487,0.473840379714966,
5.37));
#45568=CARTESIAN_POINT('Ctrl Pts',(-0.721452966332436,0.473090016841888,
5.37));
#45569=CARTESIAN_POINT('Ctrl Pts',(-0.717326179146767,0.473090016841888,
5.37));
#45570=CARTESIAN_POINT('Origin',(-0.735709443688393,0.41456344127655,5.4));
#45571=CARTESIAN_POINT('',(-0.735709443688393,0.41456344127655,5.4));
#45572=CARTESIAN_POINT('',(-0.755732388442078,0.256379251042444,5.4));
#45573=CARTESIAN_POINT('',(-0.735709443688393,0.41456344127655,5.37));
#45574=CARTESIAN_POINT('',(-0.735709443688393,0.41456344127655,5.4));
#45575=CARTESIAN_POINT('',(-0.735709443688393,0.41456344127655,5.37));
#45576=CARTESIAN_POINT('Ctrl Pts',(-0.68806292116642,0.422066831588745,
5.4));
#45577=CARTESIAN_POINT('Ctrl Pts',(-0.68806292116642,0.422066831588745,
5.37));
#45578=CARTESIAN_POINT('Ctrl Pts',(-0.707196488976479,0.422066831588745,
5.4));
#45579=CARTESIAN_POINT('Ctrl Pts',(-0.707196488976479,0.422066831588745,
5.37));
#45580=CARTESIAN_POINT('Ctrl Pts',(-0.735709443688393,0.41456344127655,
5.4));
#45581=CARTESIAN_POINT('Ctrl Pts',(-0.735709443688393,0.41456344127655,
5.37));
#45582=CARTESIAN_POINT('',(-0.68806292116642,0.422066831588745,5.4));
#45583=CARTESIAN_POINT('Ctrl Pts',(-0.68806292116642,0.422066831588745,
5.4));
#45584=CARTESIAN_POINT('Ctrl Pts',(-0.707196488976479,0.422066831588745,
5.4));
#45585=CARTESIAN_POINT('Ctrl Pts',(-0.735709443688393,0.41456344127655,
5.4));
#45586=CARTESIAN_POINT('',(-0.68806292116642,0.422066831588745,5.37));
#45587=CARTESIAN_POINT('',(-0.68806292116642,0.422066831588745,5.4));
#45588=CARTESIAN_POINT('Ctrl Pts',(-0.68806292116642,0.422066831588745,
5.37));
#45589=CARTESIAN_POINT('Ctrl Pts',(-0.707196488976479,0.422066831588745,
5.37));
#45590=CARTESIAN_POINT('Ctrl Pts',(-0.735709443688393,0.41456344127655,
5.37));
#45591=CARTESIAN_POINT('Ctrl Pts',(-0.610777631402016,0.391865620017052,
5.4));
#45592=CARTESIAN_POINT('Ctrl Pts',(-0.610777631402016,0.391865620017052,
5.37));
#45593=CARTESIAN_POINT('Ctrl Pts',(-0.641166463494301,0.422066831588745,
5.4));
#45594=CARTESIAN_POINT('Ctrl Pts',(-0.641166463494301,0.422066831588745,
5.37));
#45595=CARTESIAN_POINT('Ctrl Pts',(-0.68806292116642,0.422066831588745,
5.4));
#45596=CARTESIAN_POINT('Ctrl Pts',(-0.68806292116642,0.422066831588745,
5.37));
#45597=CARTESIAN_POINT('',(-0.610777631402016,0.391865620017052,5.4));
#45598=CARTESIAN_POINT('Ctrl Pts',(-0.610777631402016,0.391865620017052,
5.4));
#45599=CARTESIAN_POINT('Ctrl Pts',(-0.641166463494301,0.422066831588745,
5.4));
#45600=CARTESIAN_POINT('Ctrl Pts',(-0.68806292116642,0.422066831588745,
5.4));
#45601=CARTESIAN_POINT('',(-0.610777631402016,0.391865620017052,5.37));
#45602=CARTESIAN_POINT('',(-0.610777631402016,0.391865620017052,5.4));
#45603=CARTESIAN_POINT('Ctrl Pts',(-0.610777631402016,0.391865620017052,
5.37));
#45604=CARTESIAN_POINT('Ctrl Pts',(-0.641166463494301,0.422066831588745,
5.37));
#45605=CARTESIAN_POINT('Ctrl Pts',(-0.68806292116642,0.422066831588745,
5.37));
#45606=CARTESIAN_POINT('Ctrl Pts',(-0.58038903772831,0.315143251419067,
5.4));
#45607=CARTESIAN_POINT('Ctrl Pts',(-0.58038903772831,0.315143251419067,
5.37));
#45608=CARTESIAN_POINT('Ctrl Pts',(-0.58038903772831,0.361664393544197,
5.4));
#45609=CARTESIAN_POINT('Ctrl Pts',(-0.58038903772831,0.361664393544197,
5.37));
#45610=CARTESIAN_POINT('Ctrl Pts',(-0.610777631402016,0.391865620017052,
5.4));
#45611=CARTESIAN_POINT('Ctrl Pts',(-0.610777631402016,0.391865620017052,
5.37));
#45612=CARTESIAN_POINT('',(-0.58038903772831,0.315143251419067,5.4));
#45613=CARTESIAN_POINT('Ctrl Pts',(-0.58038903772831,0.315143251419067,
5.4));
#45614=CARTESIAN_POINT('Ctrl Pts',(-0.58038903772831,0.361664393544197,
5.4));
#45615=CARTESIAN_POINT('Ctrl Pts',(-0.610777631402016,0.391865620017052,
5.4));
#45616=CARTESIAN_POINT('',(-0.58038903772831,0.315143251419067,5.37));
#45617=CARTESIAN_POINT('',(-0.58038903772831,0.315143251419067,5.4));
#45618=CARTESIAN_POINT('Ctrl Pts',(-0.58038903772831,0.315143251419067,
5.37));
#45619=CARTESIAN_POINT('Ctrl Pts',(-0.58038903772831,0.361664393544197,
5.37));
#45620=CARTESIAN_POINT('Ctrl Pts',(-0.610777631402016,0.391865620017052,
5.37));
#45621=CARTESIAN_POINT('Ctrl Pts',(-0.613216415047646,0.233356082439423,
5.4));
#45622=CARTESIAN_POINT('Ctrl Pts',(-0.613216415047646,0.233356082439423,
5.37));
#45623=CARTESIAN_POINT('Ctrl Pts',(-0.58038903772831,0.266371095180511,
5.4));
#45624=CARTESIAN_POINT('Ctrl Pts',(-0.58038903772831,0.266371095180511,
5.37));
#45625=CARTESIAN_POINT('Ctrl Pts',(-0.58038903772831,0.315143251419067,
5.4));
#45626=CARTESIAN_POINT('Ctrl Pts',(-0.58038903772831,0.315143251419067,
5.37));
#45627=CARTESIAN_POINT('',(-0.613216415047646,0.233356082439423,5.4));
#45628=CARTESIAN_POINT('Ctrl Pts',(-0.613216415047646,0.233356082439423,
5.4));
#45629=CARTESIAN_POINT('Ctrl Pts',(-0.58038903772831,0.266371095180511,
5.4));
#45630=CARTESIAN_POINT('Ctrl Pts',(-0.58038903772831,0.315143251419067,
5.4));
#45631=CARTESIAN_POINT('',(-0.613216415047646,0.233356082439423,5.37));
#45632=CARTESIAN_POINT('',(-0.613216415047646,0.233356082439423,5.4));
#45633=CARTESIAN_POINT('Ctrl Pts',(-0.613216415047646,0.233356082439423,
5.37));
#45634=CARTESIAN_POINT('Ctrl Pts',(-0.58038903772831,0.266371095180511,
5.37));
#45635=CARTESIAN_POINT('Ctrl Pts',(-0.58038903772831,0.315143251419067,
5.37));
#45636=CARTESIAN_POINT('Ctrl Pts',(-0.693690314888954,0.200341069698334,
5.4));
#45637=CARTESIAN_POINT('Ctrl Pts',(-0.693690314888954,0.200341069698334,
5.37));
#45638=CARTESIAN_POINT('Ctrl Pts',(-0.646043792366982,0.200341069698334,
5.4));
#45639=CARTESIAN_POINT('Ctrl Pts',(-0.646043792366982,0.200341069698334,
5.37));
#45640=CARTESIAN_POINT('Ctrl Pts',(-0.613216415047646,0.233356082439423,
5.4));
#45641=CARTESIAN_POINT('Ctrl Pts',(-0.613216415047646,0.233356082439423,
5.37));
#45642=CARTESIAN_POINT('',(-0.693690314888954,0.200341069698334,5.4));
#45643=CARTESIAN_POINT('Ctrl Pts',(-0.693690314888954,0.200341069698334,
5.4));
#45644=CARTESIAN_POINT('Ctrl Pts',(-0.646043792366982,0.200341069698334,
5.4));
#45645=CARTESIAN_POINT('Ctrl Pts',(-0.613216415047646,0.233356082439423,
5.4));
#45646=CARTESIAN_POINT('',(-0.693690314888954,0.200341069698334,5.37));
#45647=CARTESIAN_POINT('',(-0.693690314888954,0.200341069698334,5.4));
#45648=CARTESIAN_POINT('Ctrl Pts',(-0.693690314888954,0.200341069698334,
5.37));
#45649=CARTESIAN_POINT('Ctrl Pts',(-0.646043792366982,0.200341069698334,
5.37));
#45650=CARTESIAN_POINT('Ctrl Pts',(-0.613216415047646,0.233356082439423,
5.37));
#45651=CARTESIAN_POINT('Ctrl Pts',(-0.761783853173256,0.225665086507797,
5.4));
#45652=CARTESIAN_POINT('Ctrl Pts',(-0.761783853173256,0.225665086507797,
5.37));
#45653=CARTESIAN_POINT('Ctrl Pts',(-0.733833566308022,0.200341069698334,
5.4));
#45654=CARTESIAN_POINT('Ctrl Pts',(-0.733833566308022,0.200341069698334,
5.37));
#45655=CARTESIAN_POINT('Ctrl Pts',(-0.693690314888954,0.200341069698334,
5.4));
#45656=CARTESIAN_POINT('Ctrl Pts',(-0.693690314888954,0.200341069698334,
5.37));
#45657=CARTESIAN_POINT('',(-0.761783853173256,0.225665086507797,5.4));
#45658=CARTESIAN_POINT('Ctrl Pts',(-0.761783853173256,0.225665086507797,
5.4));
#45659=CARTESIAN_POINT('Ctrl Pts',(-0.733833566308022,0.200341069698334,
5.4));
#45660=CARTESIAN_POINT('Ctrl Pts',(-0.693690314888954,0.200341069698334,
5.4));
#45661=CARTESIAN_POINT('',(-0.761783853173256,0.225665086507797,5.37));
#45662=CARTESIAN_POINT('',(-0.761783853173256,0.225665086507797,5.4));
#45663=CARTESIAN_POINT('Ctrl Pts',(-0.761783853173256,0.225665086507797,
5.37));
#45664=CARTESIAN_POINT('Ctrl Pts',(-0.733833566308022,0.200341069698334,
5.37));
#45665=CARTESIAN_POINT('Ctrl Pts',(-0.693690314888954,0.200341069698334,
5.37));
#45666=CARTESIAN_POINT('Ctrl Pts',(-0.801364436745644,0.308390179276466,
5.4));
#45667=CARTESIAN_POINT('Ctrl Pts',(-0.801364436745644,0.308390179276466,
5.37));
#45668=CARTESIAN_POINT('Ctrl Pts',(-0.78973414003849,0.250989103317261,
5.4));
#45669=CARTESIAN_POINT('Ctrl Pts',(-0.78973414003849,0.250989103317261,
5.37));
#45670=CARTESIAN_POINT('Ctrl Pts',(-0.761783853173256,0.225665086507797,
5.4));
#45671=CARTESIAN_POINT('Ctrl Pts',(-0.761783853173256,0.225665086507797,
5.37));
#45672=CARTESIAN_POINT('',(-0.801364436745644,0.308390179276466,5.4));
#45673=CARTESIAN_POINT('Ctrl Pts',(-0.801364436745644,0.308390179276466,
5.4));
#45674=CARTESIAN_POINT('Ctrl Pts',(-0.78973414003849,0.250989103317261,
5.4));
#45675=CARTESIAN_POINT('Ctrl Pts',(-0.761783853173256,0.225665086507797,
5.4));
#45676=CARTESIAN_POINT('',(-0.801364436745644,0.308390179276466,5.37));
#45677=CARTESIAN_POINT('',(-0.801364436745644,0.308390179276466,5.4));
#45678=CARTESIAN_POINT('Ctrl Pts',(-0.801364436745644,0.308390179276466,
5.37));
#45679=CARTESIAN_POINT('Ctrl Pts',(-0.78973414003849,0.250989103317261,
5.37));
#45680=CARTESIAN_POINT('Ctrl Pts',(-0.761783853173256,0.225665086507797,
5.37));
#45681=CARTESIAN_POINT('Origin',(-0.868895068764687,0.299386093020439,5.4));
#45682=CARTESIAN_POINT('',(-0.868895068764687,0.299386093020439,5.4));
#45683=CARTESIAN_POINT('',(-0.461646587843761,0.353685902458237,5.4));
#45684=CARTESIAN_POINT('',(-0.868895068764687,0.299386093020439,5.37));
#45685=CARTESIAN_POINT('',(-0.868895068764687,0.299386093020439,5.4));
#45686=CARTESIAN_POINT('',(-0.868895068764687,0.299386093020439,5.37));
#45687=CARTESIAN_POINT('Ctrl Pts',(-0.814307704567909,0.187585258483887,
5.4));
#45688=CARTESIAN_POINT('Ctrl Pts',(-0.814307704567909,0.187585258483887,
5.37));
#45689=CARTESIAN_POINT('Ctrl Pts',(-0.862142100930214,0.230729871988297,
5.4));
#45690=CARTESIAN_POINT('Ctrl Pts',(-0.862142100930214,0.230729871988297,
5.37));
#45691=CARTESIAN_POINT('Ctrl Pts',(-0.868895068764687,0.299386093020439,
5.4));
#45692=CARTESIAN_POINT('Ctrl Pts',(-0.868895068764687,0.299386093020439,
5.37));
#45693=CARTESIAN_POINT('',(-0.814307704567909,0.187585258483887,5.4));
#45694=CARTESIAN_POINT('Ctrl Pts',(-0.814307704567909,0.187585258483887,
5.4));
#45695=CARTESIAN_POINT('Ctrl Pts',(-0.862142100930214,0.230729871988297,
5.4));
#45696=CARTESIAN_POINT('Ctrl Pts',(-0.868895068764687,0.299386093020439,
5.4));
#45697=CARTESIAN_POINT('',(-0.814307704567909,0.187585258483887,5.37));
#45698=CARTESIAN_POINT('',(-0.814307704567909,0.187585258483887,5.4));
#45699=CARTESIAN_POINT('Ctrl Pts',(-0.814307704567909,0.187585258483887,
5.37));
#45700=CARTESIAN_POINT('Ctrl Pts',(-0.862142100930214,0.230729871988297,
5.37));
#45701=CARTESIAN_POINT('Ctrl Pts',(-0.868895068764687,0.299386093020439,
5.37));
#45702=CARTESIAN_POINT('Ctrl Pts',(-0.69406558573246,0.144440674781799,
5.4));
#45703=CARTESIAN_POINT('Ctrl Pts',(-0.69406558573246,0.144440674781799,
5.37));
#45704=CARTESIAN_POINT('Ctrl Pts',(-0.766473546624184,0.144440674781799,
5.4));
#45705=CARTESIAN_POINT('Ctrl Pts',(-0.766473546624184,0.144440674781799,
5.37));
#45706=CARTESIAN_POINT('Ctrl Pts',(-0.814307704567909,0.187585258483887,
5.4));
#45707=CARTESIAN_POINT('Ctrl Pts',(-0.814307704567909,0.187585258483887,
5.37));
#45708=CARTESIAN_POINT('Ctrl Pts',(-0.69406558573246,0.144440674781799,
5.4));
#45709=CARTESIAN_POINT('Ctrl Pts',(-0.766473546624184,0.144440674781799,
5.4));
#45710=CARTESIAN_POINT('Ctrl Pts',(-0.814307704567909,0.187585258483887,
5.4));
#45711=CARTESIAN_POINT('Ctrl Pts',(-0.69406558573246,0.144440674781799,
5.37));
#45712=CARTESIAN_POINT('Ctrl Pts',(-0.766473546624184,0.144440674781799,
5.37));
#45713=CARTESIAN_POINT('Ctrl Pts',(-0.814307704567909,0.187585258483887,
5.37));
#45714=CARTESIAN_POINT('Origin',(-0.688813224434853,0.425443404912949,5.37));
#45715=CARTESIAN_POINT('Ctrl Pts',(0.177080616354942,0.324897700548172,
5.4));
#45716=CARTESIAN_POINT('Ctrl Pts',(0.177080616354942,0.324897700548172,
5.37));
#45717=CARTESIAN_POINT('Ctrl Pts',(0.116302952170372,0.273874485492706,
5.4));
#45718=CARTESIAN_POINT('Ctrl Pts',(0.116302952170372,0.273874485492706,
5.37));
#45719=CARTESIAN_POINT('Ctrl Pts',(0.0990450233221054,0.255678737163544,
5.4));
#45720=CARTESIAN_POINT('Ctrl Pts',(0.0990450233221054,0.255678737163544,
5.37));
#45721=CARTESIAN_POINT('',(0.177080616354942,0.324897700548172,5.4));
#45722=CARTESIAN_POINT('',(0.0990450233221054,0.255678737163544,5.4));
#45723=CARTESIAN_POINT('Ctrl Pts',(0.177080616354942,0.324897700548172,
5.4));
#45724=CARTESIAN_POINT('Ctrl Pts',(0.116302952170372,0.273874485492706,
5.4));
#45725=CARTESIAN_POINT('Ctrl Pts',(0.0990450233221054,0.255678737163544,
5.4));
#45726=CARTESIAN_POINT('',(0.177080616354942,0.324897700548172,5.37));
#45727=CARTESIAN_POINT('',(0.177080616354942,0.324897700548172,5.4));
#45728=CARTESIAN_POINT('',(0.0990450233221054,0.255678737163544,5.37));
#45729=CARTESIAN_POINT('Ctrl Pts',(0.177080616354942,0.324897700548172,
5.37));
#45730=CARTESIAN_POINT('Ctrl Pts',(0.116302952170372,0.273874485492706,
5.37));
#45731=CARTESIAN_POINT('Ctrl Pts',(0.0990450233221054,0.255678737163544,
5.37));
#45732=CARTESIAN_POINT('',(0.0990450233221054,0.255678737163544,5.4));
#45733=CARTESIAN_POINT('Ctrl Pts',(0.281190380454063,0.421691709756851,
5.4));
#45734=CARTESIAN_POINT('Ctrl Pts',(0.281190380454063,0.421691709756851,
5.37));
#45735=CARTESIAN_POINT('Ctrl Pts',(0.249863609671593,0.386425668001175,
5.4));
#45736=CARTESIAN_POINT('Ctrl Pts',(0.249863609671593,0.386425668001175,
5.37));
#45737=CARTESIAN_POINT('Ctrl Pts',(0.177080616354942,0.324897700548172,
5.4));
#45738=CARTESIAN_POINT('Ctrl Pts',(0.177080616354942,0.324897700548172,
5.37));
#45739=CARTESIAN_POINT('',(0.281190380454063,0.421691709756851,5.4));
#45740=CARTESIAN_POINT('Ctrl Pts',(0.281190380454063,0.421691709756851,
5.4));
#45741=CARTESIAN_POINT('Ctrl Pts',(0.249863609671593,0.386425668001175,
5.4));
#45742=CARTESIAN_POINT('Ctrl Pts',(0.177080616354942,0.324897700548172,
5.4));
#45743=CARTESIAN_POINT('',(0.281190380454063,0.421691709756851,5.37));
#45744=CARTESIAN_POINT('',(0.281190380454063,0.421691709756851,5.4));
#45745=CARTESIAN_POINT('Ctrl Pts',(0.281190380454063,0.421691709756851,
5.37));
#45746=CARTESIAN_POINT('Ctrl Pts',(0.249863609671593,0.386425668001175,
5.37));
#45747=CARTESIAN_POINT('Ctrl Pts',(0.177080616354942,0.324897700548172,
5.37));
#45748=CARTESIAN_POINT('Ctrl Pts',(0.326023086905479,0.488847219944,5.4));
#45749=CARTESIAN_POINT('Ctrl Pts',(0.326023086905479,0.488847219944,5.37));
#45750=CARTESIAN_POINT('Ctrl Pts',(0.312517151236534,0.456957721710205,
5.4));
#45751=CARTESIAN_POINT('Ctrl Pts',(0.312517151236534,0.456957721710205,
5.37));
#45752=CARTESIAN_POINT('Ctrl Pts',(0.281190380454063,0.421691709756851,
5.4));
#45753=CARTESIAN_POINT('Ctrl Pts',(0.281190380454063,0.421691709756851,
5.37));
#45754=CARTESIAN_POINT('',(0.326023086905479,0.488847219944,5.4));
#45755=CARTESIAN_POINT('Ctrl Pts',(0.326023086905479,0.488847219944,5.4));
#45756=CARTESIAN_POINT('Ctrl Pts',(0.312517151236534,0.456957721710205,
5.4));
#45757=CARTESIAN_POINT('Ctrl Pts',(0.281190380454063,0.421691709756851,
5.4));
#45758=CARTESIAN_POINT('',(0.326023086905479,0.488847219944,5.37));
#45759=CARTESIAN_POINT('',(0.326023086905479,0.488847219944,5.4));
#45760=CARTESIAN_POINT('Ctrl Pts',(0.326023086905479,0.488847219944,5.37));
#45761=CARTESIAN_POINT('Ctrl Pts',(0.312517151236534,0.456957721710205,
5.37));
#45762=CARTESIAN_POINT('Ctrl Pts',(0.281190380454063,0.421691709756851,
5.37));
#45763=CARTESIAN_POINT('Ctrl Pts',(0.339529260993004,0.553751730918884,
5.4));
#45764=CARTESIAN_POINT('Ctrl Pts',(0.339529260993004,0.553751730918884,
5.37));
#45765=CARTESIAN_POINT('Ctrl Pts',(0.339529260993004,0.520736718177795,
5.4));
#45766=CARTESIAN_POINT('Ctrl Pts',(0.339529260993004,0.520736718177795,
5.37));
#45767=CARTESIAN_POINT('Ctrl Pts',(0.326023086905479,0.488847219944,5.4));
#45768=CARTESIAN_POINT('Ctrl Pts',(0.326023086905479,0.488847219944,5.37));
#45769=CARTESIAN_POINT('',(0.339529260993004,0.553751730918884,5.4));
#45770=CARTESIAN_POINT('Ctrl Pts',(0.339529260993004,0.553751730918884,
5.4));
#45771=CARTESIAN_POINT('Ctrl Pts',(0.339529260993004,0.520736718177795,
5.4));
#45772=CARTESIAN_POINT('Ctrl Pts',(0.326023086905479,0.488847219944,5.4));
#45773=CARTESIAN_POINT('',(0.339529260993004,0.553751730918884,5.37));
#45774=CARTESIAN_POINT('',(0.339529260993004,0.553751730918884,5.4));
#45775=CARTESIAN_POINT('Ctrl Pts',(0.339529260993004,0.553751730918884,
5.37));
#45776=CARTESIAN_POINT('Ctrl Pts',(0.339529260993004,0.520736718177795,
5.37));
#45777=CARTESIAN_POINT('Ctrl Pts',(0.326023086905479,0.488847219944,5.37));
#45778=CARTESIAN_POINT('Ctrl Pts',(0.293383345007896,0.662551188468933,
5.4));
#45779=CARTESIAN_POINT('Ctrl Pts',(0.293383345007896,0.662551188468933,
5.37));
#45780=CARTESIAN_POINT('Ctrl Pts',(0.339529260993004,0.618656241893768,
5.4));
#45781=CARTESIAN_POINT('Ctrl Pts',(0.339529260993004,0.618656241893768,
5.37));
#45782=CARTESIAN_POINT('Ctrl Pts',(0.339529260993004,0.553751730918884,
5.4));
#45783=CARTESIAN_POINT('Ctrl Pts',(0.339529260993004,0.553751730918884,
5.37));
#45784=CARTESIAN_POINT('',(0.293383345007896,0.662551188468933,5.4));
#45785=CARTESIAN_POINT('Ctrl Pts',(0.293383345007896,0.662551188468933,
5.4));
#45786=CARTESIAN_POINT('Ctrl Pts',(0.339529260993004,0.618656241893768,
5.4));
#45787=CARTESIAN_POINT('Ctrl Pts',(0.339529260993004,0.553751730918884,
5.4));
#45788=CARTESIAN_POINT('',(0.293383345007896,0.662551188468933,5.37));
#45789=CARTESIAN_POINT('',(0.293383345007896,0.662551188468933,5.4));
#45790=CARTESIAN_POINT('Ctrl Pts',(0.293383345007896,0.662551188468933,
5.37));
#45791=CARTESIAN_POINT('Ctrl Pts',(0.339529260993004,0.618656241893768,
5.37));
#45792=CARTESIAN_POINT('Ctrl Pts',(0.339529260993004,0.553751730918884,
5.37));
#45793=CARTESIAN_POINT('Ctrl Pts',(0.168076500296593,0.706446135044098,
5.4));
#45794=CARTESIAN_POINT('Ctrl Pts',(0.168076500296593,0.706446135044098,
5.37));
#45795=CARTESIAN_POINT('Ctrl Pts',(0.247237429022789,0.706446135044098,
5.4));
#45796=CARTESIAN_POINT('Ctrl Pts',(0.247237429022789,0.706446135044098,
5.37));
#45797=CARTESIAN_POINT('Ctrl Pts',(0.293383345007896,0.662551188468933,
5.4));
#45798=CARTESIAN_POINT('Ctrl Pts',(0.293383345007896,0.662551188468933,
5.37));
#45799=CARTESIAN_POINT('',(0.168076500296593,0.706446135044098,5.4));
#45800=CARTESIAN_POINT('Ctrl Pts',(0.168076500296593,0.706446135044098,
5.4));
#45801=CARTESIAN_POINT('Ctrl Pts',(0.247237429022789,0.706446135044098,
5.4));
#45802=CARTESIAN_POINT('Ctrl Pts',(0.293383345007896,0.662551188468933,
5.4));
#45803=CARTESIAN_POINT('',(0.168076500296593,0.706446135044098,5.37));
#45804=CARTESIAN_POINT('',(0.168076500296593,0.706446135044098,5.4));
#45805=CARTESIAN_POINT('Ctrl Pts',(0.168076500296593,0.706446135044098,
5.37));
#45806=CARTESIAN_POINT('Ctrl Pts',(0.247237429022789,0.706446135044098,
5.37));
#45807=CARTESIAN_POINT('Ctrl Pts',(0.293383345007896,0.662551188468933,
5.37));
#45808=CARTESIAN_POINT('Ctrl Pts',(0.0431446880102158,0.665740156173706,
5.4));
#45809=CARTESIAN_POINT('Ctrl Pts',(0.0431446880102158,0.665740156173706,
5.37));
#45810=CARTESIAN_POINT('Ctrl Pts',(0.089665874838829,0.706446135044098,
5.4));
#45811=CARTESIAN_POINT('Ctrl Pts',(0.089665874838829,0.706446135044098,
5.37));
#45812=CARTESIAN_POINT('Ctrl Pts',(0.168076500296593,0.706446135044098,
5.4));
#45813=CARTESIAN_POINT('Ctrl Pts',(0.168076500296593,0.706446135044098,
5.37));
#45814=CARTESIAN_POINT('',(0.0431446880102158,0.665740156173706,5.4));
#45815=CARTESIAN_POINT('Ctrl Pts',(0.0431446880102158,0.665740156173706,
5.4));
#45816=CARTESIAN_POINT('Ctrl Pts',(0.089665874838829,0.706446135044098,
5.4));
#45817=CARTESIAN_POINT('Ctrl Pts',(0.168076500296593,0.706446135044098,
5.4));
#45818=CARTESIAN_POINT('',(0.0431446880102158,0.665740156173706,5.37));
#45819=CARTESIAN_POINT('',(0.0431446880102158,0.665740156173706,5.4));
#45820=CARTESIAN_POINT('Ctrl Pts',(0.0431446880102158,0.665740156173706,
5.37));
#45821=CARTESIAN_POINT('Ctrl Pts',(0.089665874838829,0.706446135044098,
5.37));
#45822=CARTESIAN_POINT('Ctrl Pts',(0.168076500296593,0.706446135044098,
5.37));
#45823=CARTESIAN_POINT('Ctrl Pts',(-0.010504737496376,0.547373825311661,
5.4));
#45824=CARTESIAN_POINT('Ctrl Pts',(-0.010504737496376,0.547373825311661,
5.37));
#45825=CARTESIAN_POINT('Ctrl Pts',(-0.00337649881839752,0.625034147500992,
5.4));
#45826=CARTESIAN_POINT('Ctrl Pts',(-0.00337649881839752,0.625034147500992,
5.37));
#45827=CARTESIAN_POINT('Ctrl Pts',(0.0431446880102158,0.665740156173706,
5.4));
#45828=CARTESIAN_POINT('Ctrl Pts',(0.0431446880102158,0.665740156173706,
5.37));
#45829=CARTESIAN_POINT('',(-0.010504737496376,0.547373825311661,5.4));
#45830=CARTESIAN_POINT('Ctrl Pts',(-0.010504737496376,0.547373825311661,
5.4));
#45831=CARTESIAN_POINT('Ctrl Pts',(-0.00337649881839752,0.625034147500992,
5.4));
#45832=CARTESIAN_POINT('Ctrl Pts',(0.0431446880102158,0.665740156173706,
5.4));
#45833=CARTESIAN_POINT('',(-0.010504737496376,0.547373825311661,5.37));
#45834=CARTESIAN_POINT('',(-0.010504737496376,0.547373825311661,5.4));
#45835=CARTESIAN_POINT('Ctrl Pts',(-0.010504737496376,0.547373825311661,
5.37));
#45836=CARTESIAN_POINT('Ctrl Pts',(-0.00337649881839752,0.625034147500992,
5.37));
#45837=CARTESIAN_POINT('Ctrl Pts',(0.0431446880102158,0.665740156173706,
5.37));
#45838=CARTESIAN_POINT('Origin',(0.058901771903038,0.540245586633682,5.4));
#45839=CARTESIAN_POINT('',(0.058901771903038,0.540245586633682,5.4));
#45840=CARTESIAN_POINT('',(0.0572110701908508,0.540419226331774,5.4));
#45841=CARTESIAN_POINT('',(0.058901771903038,0.540245586633682,5.37));
#45842=CARTESIAN_POINT('',(0.058901771903038,0.540245586633682,5.4));
#45843=CARTESIAN_POINT('',(0.058901771903038,0.540245586633682,5.37));
#45844=CARTESIAN_POINT('Ctrl Pts',(0.0885403007268906,0.621282422542572,
5.4));
#45845=CARTESIAN_POINT('Ctrl Pts',(0.0885403007268906,0.621282422542572,
5.37));
#45846=CARTESIAN_POINT('Ctrl Pts',(0.0592770427465439,0.592019134759903,
5.4));
#45847=CARTESIAN_POINT('Ctrl Pts',(0.0592770427465439,0.592019134759903,
5.37));
#45848=CARTESIAN_POINT('Ctrl Pts',(0.058901771903038,0.540245586633682,
5.4));
#45849=CARTESIAN_POINT('Ctrl Pts',(0.058901771903038,0.540245586633682,
5.37));
#45850=CARTESIAN_POINT('',(0.0885403007268906,0.621282422542572,5.4));
#45851=CARTESIAN_POINT('Ctrl Pts',(0.0885403007268906,0.621282422542572,
5.4));
#45852=CARTESIAN_POINT('Ctrl Pts',(0.0592770427465439,0.592019134759903,
5.4));
#45853=CARTESIAN_POINT('Ctrl Pts',(0.058901771903038,0.540245586633682,
5.4));
#45854=CARTESIAN_POINT('',(0.0885403007268906,0.621282422542572,5.37));
#45855=CARTESIAN_POINT('',(0.0885403007268906,0.621282422542572,5.4));
#45856=CARTESIAN_POINT('Ctrl Pts',(0.0885403007268906,0.621282422542572,
5.37));
#45857=CARTESIAN_POINT('Ctrl Pts',(0.0592770427465439,0.592019134759903,
5.37));
#45858=CARTESIAN_POINT('Ctrl Pts',(0.058901771903038,0.540245586633682,
5.37));
#45859=CARTESIAN_POINT('Ctrl Pts',(0.166575655341148,0.650545740127563,
5.4));
#45860=CARTESIAN_POINT('Ctrl Pts',(0.166575655341148,0.650545740127563,
5.37));
#45861=CARTESIAN_POINT('Ctrl Pts',(0.117803558707237,0.650545740127563,
5.4));
#45862=CARTESIAN_POINT('Ctrl Pts',(0.117803558707237,0.650545740127563,
5.37));
#45863=CARTESIAN_POINT('Ctrl Pts',(0.0885403007268906,0.621282422542572,
5.4));
#45864=CARTESIAN_POINT('Ctrl Pts',(0.0885403007268906,0.621282422542572,
5.37));
#45865=CARTESIAN_POINT('',(0.166575655341148,0.650545740127563,5.4));
#45866=CARTESIAN_POINT('Ctrl Pts',(0.166575655341148,0.650545740127563,
5.4));
#45867=CARTESIAN_POINT('Ctrl Pts',(0.117803558707237,0.650545740127563,
5.4));
#45868=CARTESIAN_POINT('Ctrl Pts',(0.0885403007268906,0.621282422542572,
5.4));
#45869=CARTESIAN_POINT('',(0.166575655341148,0.650545740127563,5.37));
#45870=CARTESIAN_POINT('',(0.166575655341148,0.650545740127563,5.4));
#45871=CARTESIAN_POINT('Ctrl Pts',(0.166575655341148,0.650545740127563,
5.37));
#45872=CARTESIAN_POINT('Ctrl Pts',(0.117803558707237,0.650545740127563,
5.37));
#45873=CARTESIAN_POINT('Ctrl Pts',(0.0885403007268906,0.621282422542572,
5.37));
#45874=CARTESIAN_POINT('Ctrl Pts',(0.241422161459923,0.622970694303513,
5.4));
#45875=CARTESIAN_POINT('Ctrl Pts',(0.241422161459923,0.622970694303513,
5.37));
#45876=CARTESIAN_POINT('Ctrl Pts',(0.212721809744835,0.650545740127563,
5.4));
#45877=CARTESIAN_POINT('Ctrl Pts',(0.212721809744835,0.650545740127563,
5.37));
#45878=CARTESIAN_POINT('Ctrl Pts',(0.166575655341148,0.650545740127563,
5.4));
#45879=CARTESIAN_POINT('Ctrl Pts',(0.166575655341148,0.650545740127563,
5.37));
#45880=CARTESIAN_POINT('',(0.241422161459923,0.622970694303513,5.4));
#45881=CARTESIAN_POINT('Ctrl Pts',(0.241422161459923,0.622970694303513,
5.4));
#45882=CARTESIAN_POINT('Ctrl Pts',(0.212721809744835,0.650545740127563,
5.4));
#45883=CARTESIAN_POINT('Ctrl Pts',(0.166575655341148,0.650545740127563,
5.4));
#45884=CARTESIAN_POINT('',(0.241422161459923,0.622970694303513,5.37));
#45885=CARTESIAN_POINT('',(0.241422161459923,0.622970694303513,5.4));
#45886=CARTESIAN_POINT('Ctrl Pts',(0.241422161459923,0.622970694303513,
5.37));
#45887=CARTESIAN_POINT('Ctrl Pts',(0.212721809744835,0.650545740127563,
5.37));
#45888=CARTESIAN_POINT('Ctrl Pts',(0.166575655341148,0.650545740127563,
5.37));
#45889=CARTESIAN_POINT('Ctrl Pts',(0.27012275159359,0.555252426862717,5.4));
#45890=CARTESIAN_POINT('Ctrl Pts',(0.27012275159359,0.555252426862717,5.37));
#45891=CARTESIAN_POINT('Ctrl Pts',(0.27012275159359,0.595395648479462,5.4));
#45892=CARTESIAN_POINT('Ctrl Pts',(0.27012275159359,0.595395648479462,5.37));
#45893=CARTESIAN_POINT('Ctrl Pts',(0.241422161459923,0.622970694303513,
5.4));
#45894=CARTESIAN_POINT('Ctrl Pts',(0.241422161459923,0.622970694303513,
5.37));
#45895=CARTESIAN_POINT('',(0.27012275159359,0.555252426862717,5.4));
#45896=CARTESIAN_POINT('Ctrl Pts',(0.27012275159359,0.555252426862717,5.4));
#45897=CARTESIAN_POINT('Ctrl Pts',(0.27012275159359,0.595395648479462,5.4));
#45898=CARTESIAN_POINT('Ctrl Pts',(0.241422161459923,0.622970694303513,
5.4));
#45899=CARTESIAN_POINT('',(0.27012275159359,0.555252426862717,5.37));
#45900=CARTESIAN_POINT('',(0.27012275159359,0.555252426862717,5.4));
#45901=CARTESIAN_POINT('Ctrl Pts',(0.27012275159359,0.555252426862717,5.37));
#45902=CARTESIAN_POINT('Ctrl Pts',(0.27012275159359,0.595395648479462,5.37));
#45903=CARTESIAN_POINT('Ctrl Pts',(0.241422161459923,0.622970694303513,
5.37));
#45904=CARTESIAN_POINT('Ctrl Pts',(0.238608345389366,0.474027985334396,
5.4));
#45905=CARTESIAN_POINT('Ctrl Pts',(0.238608345389366,0.474027985334396,
5.37));
#45906=CARTESIAN_POINT('Ctrl Pts',(0.27012275159359,0.516985023021698,5.4));
#45907=CARTESIAN_POINT('Ctrl Pts',(0.27012275159359,0.516985023021698,5.37));
#45908=CARTESIAN_POINT('Ctrl Pts',(0.27012275159359,0.555252426862717,5.4));
#45909=CARTESIAN_POINT('Ctrl Pts',(0.27012275159359,0.555252426862717,5.37));
#45910=CARTESIAN_POINT('',(0.238608345389366,0.474027985334396,5.4));
#45911=CARTESIAN_POINT('Ctrl Pts',(0.238608345389366,0.474027985334396,
5.4));
#45912=CARTESIAN_POINT('Ctrl Pts',(0.27012275159359,0.516985023021698,5.4));
#45913=CARTESIAN_POINT('Ctrl Pts',(0.27012275159359,0.555252426862717,5.4));
#45914=CARTESIAN_POINT('',(0.238608345389366,0.474027985334396,5.37));
#45915=CARTESIAN_POINT('',(0.238608345389366,0.474027985334396,5.4));
#45916=CARTESIAN_POINT('Ctrl Pts',(0.238608345389366,0.474027985334396,
5.37));
#45917=CARTESIAN_POINT('Ctrl Pts',(0.27012275159359,0.516985023021698,5.37));
#45918=CARTESIAN_POINT('Ctrl Pts',(0.27012275159359,0.555252426862717,5.37));
#45919=CARTESIAN_POINT('Ctrl Pts',(0.117428287863731,0.357537531852722,
5.4));
#45920=CARTESIAN_POINT('Ctrl Pts',(0.117428287863731,0.357537531852722,
5.37));
#45921=CARTESIAN_POINT('Ctrl Pts',(0.207094177603722,0.431070947647095,
5.4));
#45922=CARTESIAN_POINT('Ctrl Pts',(0.207094177603722,0.431070947647095,
5.37));
#45923=CARTESIAN_POINT('Ctrl Pts',(0.238608345389366,0.474027985334396,
5.4));
#45924=CARTESIAN_POINT('Ctrl Pts',(0.238608345389366,0.474027985334396,
5.37));
#45925=CARTESIAN_POINT('',(0.117428287863731,0.357537531852722,5.4));
#45926=CARTESIAN_POINT('Ctrl Pts',(0.117428287863731,0.357537531852722,
5.4));
#45927=CARTESIAN_POINT('Ctrl Pts',(0.207094177603722,0.431070947647095,
5.4));
#45928=CARTESIAN_POINT('Ctrl Pts',(0.238608345389366,0.474027985334396,
5.4));
#45929=CARTESIAN_POINT('',(0.117428287863731,0.357537531852722,5.37));
#45930=CARTESIAN_POINT('',(0.117428287863731,0.357537531852722,5.4));
#45931=CARTESIAN_POINT('Ctrl Pts',(0.117428287863731,0.357537531852722,
5.37));
#45932=CARTESIAN_POINT('Ctrl Pts',(0.207094177603722,0.431070947647095,
5.37));
#45933=CARTESIAN_POINT('Ctrl Pts',(0.238608345389366,0.474027985334396,
5.37));
#45934=CARTESIAN_POINT('Ctrl Pts',(0.0290756076574326,0.274249666929245,
5.4));
#45935=CARTESIAN_POINT('Ctrl Pts',(0.0290756076574326,0.274249666929245,
5.37));
#45936=CARTESIAN_POINT('Ctrl Pts',(0.0596520751714706,0.310266041755676,
5.4));
#45937=CARTESIAN_POINT('Ctrl Pts',(0.0596520751714706,0.310266041755676,
5.37));
#45938=CARTESIAN_POINT('Ctrl Pts',(0.117428287863731,0.357537531852722,
5.4));
#45939=CARTESIAN_POINT('Ctrl Pts',(0.117428287863731,0.357537531852722,
5.37));
#45940=CARTESIAN_POINT('',(0.0290756076574326,0.274249666929245,5.4));
#45941=CARTESIAN_POINT('Ctrl Pts',(0.0290756076574326,0.274249666929245,
5.4));
#45942=CARTESIAN_POINT('Ctrl Pts',(0.0596520751714706,0.310266041755676,
5.4));
#45943=CARTESIAN_POINT('Ctrl Pts',(0.117428287863731,0.357537531852722,
5.4));
#45944=CARTESIAN_POINT('',(0.0290756076574326,0.274249666929245,5.37));
#45945=CARTESIAN_POINT('',(0.0290756076574326,0.274249666929245,5.4));
#45946=CARTESIAN_POINT('Ctrl Pts',(0.0290756076574326,0.274249666929245,
5.37));
#45947=CARTESIAN_POINT('Ctrl Pts',(0.0596520751714706,0.310266041755676,
5.37));
#45948=CARTESIAN_POINT('Ctrl Pts',(0.117428287863731,0.357537531852722,
5.37));
#45949=CARTESIAN_POINT('Ctrl Pts',(-0.0153820663690567,0.201091402769089,
5.4));
#45950=CARTESIAN_POINT('Ctrl Pts',(-0.0153820663690567,0.201091402769089,
5.37));
#45951=CARTESIAN_POINT('Ctrl Pts',(-0.00150062143802643,0.238233292102814,
5.4));
#45952=CARTESIAN_POINT('Ctrl Pts',(-0.00150062143802643,0.238233292102814,
5.37));
#45953=CARTESIAN_POINT('Ctrl Pts',(0.0290756076574326,0.274249666929245,
5.4));
#45954=CARTESIAN_POINT('Ctrl Pts',(0.0290756076574326,0.274249666929245,
5.37));
#45955=CARTESIAN_POINT('',(-0.0153820663690567,0.201091402769089,5.4));
#45956=CARTESIAN_POINT('Ctrl Pts',(-0.0153820663690567,0.201091402769089,
5.4));
#45957=CARTESIAN_POINT('Ctrl Pts',(-0.00150062143802643,0.238233292102814,
5.4));
#45958=CARTESIAN_POINT('Ctrl Pts',(0.0290756076574326,0.274249666929245,
5.4));
#45959=CARTESIAN_POINT('',(-0.0153820663690567,0.201091402769089,5.37));
#45960=CARTESIAN_POINT('',(-0.0153820663690567,0.201091402769089,5.4));
#45961=CARTESIAN_POINT('Ctrl Pts',(-0.0153820663690567,0.201091402769089,
5.37));
#45962=CARTESIAN_POINT('Ctrl Pts',(-0.00150062143802643,0.238233292102814,
5.37));
#45963=CARTESIAN_POINT('Ctrl Pts',(0.0290756076574326,0.274249666929245,
5.37));
#45964=CARTESIAN_POINT('Ctrl Pts',(-0.0232606083154678,0.154195094108582,
5.4));
#45965=CARTESIAN_POINT('Ctrl Pts',(-0.0232606083154678,0.154195094108582,
5.37));
#45966=CARTESIAN_POINT('Ctrl Pts',(-0.0240109115839005,0.17858117222786,
5.4));
#45967=CARTESIAN_POINT('Ctrl Pts',(-0.0240109115839005,0.17858117222786,
5.37));
#45968=CARTESIAN_POINT('Ctrl Pts',(-0.0153820663690567,0.201091402769089,
5.4));
#45969=CARTESIAN_POINT('Ctrl Pts',(-0.0153820663690567,0.201091402769089,
5.37));
#45970=CARTESIAN_POINT('',(-0.0232606083154678,0.154195094108582,5.4));
#45971=CARTESIAN_POINT('Ctrl Pts',(-0.0232606083154678,0.154195094108582,
5.4));
#45972=CARTESIAN_POINT('Ctrl Pts',(-0.0240109115839005,0.17858117222786,
5.4));
#45973=CARTESIAN_POINT('Ctrl Pts',(-0.0153820663690567,0.201091402769089,
5.4));
#45974=CARTESIAN_POINT('',(-0.0232606083154678,0.154195094108582,5.37));
#45975=CARTESIAN_POINT('',(-0.0232606083154678,0.154195094108582,5.4));
#45976=CARTESIAN_POINT('Ctrl Pts',(-0.0232606083154678,0.154195094108582,
5.37));
#45977=CARTESIAN_POINT('Ctrl Pts',(-0.0240109115839005,0.17858117222786,
5.37));
#45978=CARTESIAN_POINT('Ctrl Pts',(-0.0153820663690567,0.201091402769089,
5.37));
#45979=CARTESIAN_POINT('Origin',(0.340279564261436,0.154195094108582,5.4));
#45980=CARTESIAN_POINT('',(0.340279564261436,0.154195094108582,5.4));
#45981=CARTESIAN_POINT('',(0.170139782130718,0.154195094108582,5.4));
#45982=CARTESIAN_POINT('',(0.340279564261436,0.154195094108582,5.37));
#45983=CARTESIAN_POINT('',(0.340279564261436,0.154195094108582,5.4));
#45984=CARTESIAN_POINT('',(0.340279564261436,0.154195094108582,5.37));
#45985=CARTESIAN_POINT('Origin',(0.340279564261436,0.219099605083466,5.4));
#45986=CARTESIAN_POINT('',(0.340279564261436,0.219099605083466,5.4));
#45987=CARTESIAN_POINT('',(0.340279564261436,0.109549802541733,5.4));
#45988=CARTESIAN_POINT('',(0.340279564261436,0.219099605083466,5.37));
#45989=CARTESIAN_POINT('',(0.340279564261436,0.219099605083466,5.4));
#45990=CARTESIAN_POINT('',(0.340279564261436,0.219099605083466,5.37));
#45991=CARTESIAN_POINT('Origin',(0.0705320686101913,0.219099605083466,5.4));
#45992=CARTESIAN_POINT('',(0.0705320686101913,0.219099605083466,5.4));
#45993=CARTESIAN_POINT('',(0.0352660343050957,0.219099605083466,5.4));
#45994=CARTESIAN_POINT('',(0.0705320686101913,0.219099605083466,5.37));
#45995=CARTESIAN_POINT('',(0.0705320686101913,0.219099605083466,5.4));
#45996=CARTESIAN_POINT('',(0.0705320686101913,0.219099605083466,5.37));
#45997=CARTESIAN_POINT('Ctrl Pts',(0.0990450233221054,0.255678737163544,
5.4));
#45998=CARTESIAN_POINT('Ctrl Pts',(0.0990450233221054,0.255678737163544,
5.37));
#45999=CARTESIAN_POINT('Ctrl Pts',(0.0817870944738388,0.237482959032059,
5.4));
#46000=CARTESIAN_POINT('Ctrl Pts',(0.0817870944738388,0.237482959032059,
5.37));
#46001=CARTESIAN_POINT('Ctrl Pts',(0.0705320686101913,0.219099605083466,
5.4));
#46002=CARTESIAN_POINT('Ctrl Pts',(0.0705320686101913,0.219099605083466,
5.37));
#46003=CARTESIAN_POINT('Ctrl Pts',(0.0990450233221054,0.255678737163544,
5.4));
#46004=CARTESIAN_POINT('Ctrl Pts',(0.0817870944738388,0.237482959032059,
5.4));
#46005=CARTESIAN_POINT('Ctrl Pts',(0.0705320686101913,0.219099605083466,
5.4));
#46006=CARTESIAN_POINT('Ctrl Pts',(0.0990450233221054,0.255678737163544,
5.37));
#46007=CARTESIAN_POINT('Ctrl Pts',(0.0817870944738388,0.237482959032059,
5.37));
#46008=CARTESIAN_POINT('Ctrl Pts',(0.0705320686101913,0.219099605083466,
5.37));
#46009=CARTESIAN_POINT('Origin',(0.158134326338768,0.43032061457634,5.37));
#46010=CARTESIAN_POINT('Origin',(1.08049105107784,0.639290624856949,5.4));
#46011=CARTESIAN_POINT('',(1.08049105107784,0.639290624856949,5.4));
#46012=CARTESIAN_POINT('',(0.939802154898643,0.639290624856949,5.4));
#46013=CARTESIAN_POINT('',(0.540245525538921,0.639290624856949,5.4));
#46014=CARTESIAN_POINT('',(1.08049105107784,0.639290624856949,5.37));
#46015=CARTESIAN_POINT('',(1.08049105107784,0.639290624856949,5.4));
#46016=CARTESIAN_POINT('',(0.939802154898643,0.639290624856949,5.37));
#46017=CARTESIAN_POINT('',(1.08049105107784,0.639290624856949,5.37));
#46018=CARTESIAN_POINT('',(0.939802154898643,0.639290624856949,5.4));
#46019=CARTESIAN_POINT('Ctrl Pts',(1.14839695394039,0.634413385391235,5.4));
#46020=CARTESIAN_POINT('Ctrl Pts',(1.14839695394039,0.634413385391235,5.37));
#46021=CARTESIAN_POINT('Ctrl Pts',(1.13001345098019,0.639290624856949,5.4));
#46022=CARTESIAN_POINT('Ctrl Pts',(1.13001345098019,0.639290624856949,5.37));
#46023=CARTESIAN_POINT('Ctrl Pts',(1.08049105107784,0.639290624856949,5.4));
#46024=CARTESIAN_POINT('Ctrl Pts',(1.08049105107784,0.639290624856949,5.37));
#46025=CARTESIAN_POINT('',(1.14839695394039,0.634413385391235,5.4));
#46026=CARTESIAN_POINT('Ctrl Pts',(1.14839695394039,0.634413385391235,5.4));
#46027=CARTESIAN_POINT('Ctrl Pts',(1.13001345098019,0.639290624856949,5.4));
#46028=CARTESIAN_POINT('Ctrl Pts',(1.08049105107784,0.639290624856949,5.4));
#46029=CARTESIAN_POINT('',(1.14839695394039,0.634413385391235,5.37));
#46030=CARTESIAN_POINT('',(1.14839695394039,0.634413385391235,5.4));
#46031=CARTESIAN_POINT('Ctrl Pts',(1.14839695394039,0.634413385391235,5.37));
#46032=CARTESIAN_POINT('Ctrl Pts',(1.13001345098019,0.639290624856949,5.37));
#46033=CARTESIAN_POINT('Ctrl Pts',(1.08049105107784,0.639290624856949,5.37));
#46034=CARTESIAN_POINT('Ctrl Pts',(1.19435547292233,0.601961159706116,5.4));
#46035=CARTESIAN_POINT('Ctrl Pts',(1.19435547292233,0.601961159706116,5.37));
#46036=CARTESIAN_POINT('Ctrl Pts',(1.17690990865231,0.626534813642502,5.4));
#46037=CARTESIAN_POINT('Ctrl Pts',(1.17690990865231,0.626534813642502,5.37));
#46038=CARTESIAN_POINT('Ctrl Pts',(1.14839695394039,0.634413385391235,5.4));
#46039=CARTESIAN_POINT('Ctrl Pts',(1.14839695394039,0.634413385391235,5.37));
#46040=CARTESIAN_POINT('',(1.19435547292233,0.601961159706116,5.4));
#46041=CARTESIAN_POINT('Ctrl Pts',(1.19435547292233,0.601961159706116,5.4));
#46042=CARTESIAN_POINT('Ctrl Pts',(1.17690990865231,0.626534813642502,5.4));
#46043=CARTESIAN_POINT('Ctrl Pts',(1.14839695394039,0.634413385391235,5.4));
#46044=CARTESIAN_POINT('',(1.19435547292233,0.601961159706116,5.37));
#46045=CARTESIAN_POINT('',(1.19435547292233,0.601961159706116,5.4));
#46046=CARTESIAN_POINT('Ctrl Pts',(1.19435547292233,0.601961159706116,5.37));
#46047=CARTESIAN_POINT('Ctrl Pts',(1.17690990865231,0.626534813642502,5.37));
#46048=CARTESIAN_POINT('Ctrl Pts',(1.14839695394039,0.634413385391235,5.37));
#46049=CARTESIAN_POINT('Ctrl Pts',(1.21180103719234,0.542871797084808,5.4));
#46050=CARTESIAN_POINT('Ctrl Pts',(1.21180103719234,0.542871797084808,5.37));
#46051=CARTESIAN_POINT('Ctrl Pts',(1.21180103719234,0.577387475967407,5.4));
#46052=CARTESIAN_POINT('Ctrl Pts',(1.21180103719234,0.577387475967407,5.37));
#46053=CARTESIAN_POINT('Ctrl Pts',(1.19435547292233,0.601961159706116,5.4));
#46054=CARTESIAN_POINT('Ctrl Pts',(1.19435547292233,0.601961159706116,5.37));
#46055=CARTESIAN_POINT('',(1.21180103719234,0.542871797084808,5.4));
#46056=CARTESIAN_POINT('Ctrl Pts',(1.21180103719234,0.542871797084808,5.4));
#46057=CARTESIAN_POINT('Ctrl Pts',(1.21180103719234,0.577387475967407,5.4));
#46058=CARTESIAN_POINT('Ctrl Pts',(1.19435547292233,0.601961159706116,5.4));
#46059=CARTESIAN_POINT('',(1.21180103719234,0.542871797084808,5.37));
#46060=CARTESIAN_POINT('',(1.21180103719234,0.542871797084808,5.4));
#46061=CARTESIAN_POINT('Ctrl Pts',(1.21180103719234,0.542871797084808,5.37));
#46062=CARTESIAN_POINT('Ctrl Pts',(1.21180103719234,0.577387475967407,5.37));
#46063=CARTESIAN_POINT('Ctrl Pts',(1.19435547292233,0.601961159706116,5.37));
#46064=CARTESIAN_POINT('Ctrl Pts',(1.18216226994991,0.468963199853897,5.4));
#46065=CARTESIAN_POINT('Ctrl Pts',(1.18216226994991,0.468963199853897,5.37));
#46066=CARTESIAN_POINT('Ctrl Pts',(1.21180103719234,0.495225125551224,5.4));
#46067=CARTESIAN_POINT('Ctrl Pts',(1.21180103719234,0.495225125551224,5.37));
#46068=CARTESIAN_POINT('Ctrl Pts',(1.21180103719234,0.542871797084808,5.4));
#46069=CARTESIAN_POINT('Ctrl Pts',(1.21180103719234,0.542871797084808,5.37));
#46070=CARTESIAN_POINT('',(1.18216226994991,0.468963199853897,5.4));
#46071=CARTESIAN_POINT('Ctrl Pts',(1.18216226994991,0.468963199853897,5.4));
#46072=CARTESIAN_POINT('Ctrl Pts',(1.21180103719234,0.495225125551224,5.4));
#46073=CARTESIAN_POINT('Ctrl Pts',(1.21180103719234,0.542871797084808,5.4));
#46074=CARTESIAN_POINT('',(1.18216226994991,0.468963199853897,5.37));
#46075=CARTESIAN_POINT('',(1.18216226994991,0.468963199853897,5.4));
#46076=CARTESIAN_POINT('Ctrl Pts',(1.18216226994991,0.468963199853897,5.37));
#46077=CARTESIAN_POINT('Ctrl Pts',(1.21180103719234,0.495225125551224,5.37));
#46078=CARTESIAN_POINT('Ctrl Pts',(1.21180103719234,0.542871797084808,5.37));
#46079=CARTESIAN_POINT('Ctrl Pts',(1.08199213445187,0.442701244354248,5.4));
#46080=CARTESIAN_POINT('Ctrl Pts',(1.08199213445187,0.442701244354248,5.37));
#46081=CARTESIAN_POINT('Ctrl Pts',(1.15252397954464,0.442701244354248,5.4));
#46082=CARTESIAN_POINT('Ctrl Pts',(1.15252397954464,0.442701244354248,5.37));
#46083=CARTESIAN_POINT('Ctrl Pts',(1.18216226994991,0.468963199853897,5.4));
#46084=CARTESIAN_POINT('Ctrl Pts',(1.18216226994991,0.468963199853897,5.37));
#46085=CARTESIAN_POINT('',(1.08199213445187,0.442701244354248,5.4));
#46086=CARTESIAN_POINT('Ctrl Pts',(1.08199213445187,0.442701244354248,5.4));
#46087=CARTESIAN_POINT('Ctrl Pts',(1.15252397954464,0.442701244354248,5.4));
#46088=CARTESIAN_POINT('Ctrl Pts',(1.18216226994991,0.468963199853897,5.4));
#46089=CARTESIAN_POINT('',(1.08199213445187,0.442701244354248,5.37));
#46090=CARTESIAN_POINT('',(1.08199213445187,0.442701244354248,5.4));
#46091=CARTESIAN_POINT('Ctrl Pts',(1.08199213445187,0.442701244354248,5.37));
#46092=CARTESIAN_POINT('Ctrl Pts',(1.15252397954464,0.442701244354248,5.37));
#46093=CARTESIAN_POINT('Ctrl Pts',(1.18216226994991,0.468963199853897,5.37));
#46094=CARTESIAN_POINT('Origin',(0.939802154898643,0.442701244354248,5.4));
#46095=CARTESIAN_POINT('',(0.939802154898643,0.442701244354248,5.4));
#46096=CARTESIAN_POINT('',(0.469901077449322,0.442701244354248,5.4));
#46097=CARTESIAN_POINT('',(0.939802154898643,0.442701244354248,5.37));
#46098=CARTESIAN_POINT('',(0.939802154898643,0.442701244354248,5.4));
#46099=CARTESIAN_POINT('',(0.939802154898643,0.442701244354248,5.37));
#46100=CARTESIAN_POINT('Origin',(0.939802154898643,0.639290624856949,5.4));
#46101=CARTESIAN_POINT('',(0.939802154898643,0.319645312428474,5.4));
#46102=CARTESIAN_POINT('',(0.939802154898643,0.639290624856949,5.37));
#46103=CARTESIAN_POINT('Origin',(1.08086632192135,0.377796748280525,5.4));
#46104=CARTESIAN_POINT('',(1.08086632192135,0.377796748280525,5.4));
#46105=CARTESIAN_POINT('',(0.939802154898643,0.377796748280525,5.4));
#46106=CARTESIAN_POINT('',(0.540433160960674,0.377796748280525,5.4));
#46107=CARTESIAN_POINT('',(1.08086632192135,0.377796748280525,5.37));
#46108=CARTESIAN_POINT('',(1.08086632192135,0.377796748280525,5.4));
#46109=CARTESIAN_POINT('',(0.939802154898643,0.377796748280525,5.37));
#46110=CARTESIAN_POINT('',(1.08086632192135,0.377796748280525,5.37));
#46111=CARTESIAN_POINT('',(0.939802154898643,0.377796748280525,5.4));
#46112=CARTESIAN_POINT('Ctrl Pts',(1.24218986928463,0.426381343603134,5.4));
#46113=CARTESIAN_POINT('Ctrl Pts',(1.24218986928463,0.426381343603134,5.37));
#46114=CARTESIAN_POINT('Ctrl Pts',(1.19754455983639,0.377796748280525,5.4));
#46115=CARTESIAN_POINT('Ctrl Pts',(1.19754455983639,0.377796748280525,5.37));
#46116=CARTESIAN_POINT('Ctrl Pts',(1.08086632192135,0.377796748280525,5.4));
#46117=CARTESIAN_POINT('Ctrl Pts',(1.08086632192135,0.377796748280525,5.37));
#46118=CARTESIAN_POINT('',(1.24218986928463,0.426381343603134,5.4));
#46119=CARTESIAN_POINT('Ctrl Pts',(1.24218986928463,0.426381343603134,5.4));
#46120=CARTESIAN_POINT('Ctrl Pts',(1.19754455983639,0.377796748280525,5.4));
#46121=CARTESIAN_POINT('Ctrl Pts',(1.08086632192135,0.377796748280525,5.4));
#46122=CARTESIAN_POINT('',(1.24218986928463,0.426381343603134,5.37));
#46123=CARTESIAN_POINT('',(1.24218986928463,0.426381343603134,5.4));
#46124=CARTESIAN_POINT('Ctrl Pts',(1.24218986928463,0.426381343603134,5.37));
#46125=CARTESIAN_POINT('Ctrl Pts',(1.19754455983639,0.377796748280525,5.37));
#46126=CARTESIAN_POINT('Ctrl Pts',(1.08086632192135,0.377796748280525,5.37));
#46127=CARTESIAN_POINT('Ctrl Pts',(1.28683517873287,0.545122796297073,5.4));
#46128=CARTESIAN_POINT('Ctrl Pts',(1.28683517873287,0.545122796297073,5.37));
#46129=CARTESIAN_POINT('Ctrl Pts',(1.28683517873287,0.474965924024582,5.4));
#46130=CARTESIAN_POINT('Ctrl Pts',(1.28683517873287,0.474965924024582,5.37));
#46131=CARTESIAN_POINT('Ctrl Pts',(1.24218986928463,0.426381343603134,5.4));
#46132=CARTESIAN_POINT('Ctrl Pts',(1.24218986928463,0.426381343603134,5.37));
#46133=CARTESIAN_POINT('',(1.28683517873287,0.545122796297073,5.4));
#46134=CARTESIAN_POINT('Ctrl Pts',(1.28683517873287,0.545122796297073,5.4));
#46135=CARTESIAN_POINT('Ctrl Pts',(1.28683517873287,0.474965924024582,5.4));
#46136=CARTESIAN_POINT('Ctrl Pts',(1.24218986928463,0.426381343603134,5.4));
#46137=CARTESIAN_POINT('',(1.28683517873287,0.545122796297073,5.37));
#46138=CARTESIAN_POINT('',(1.28683517873287,0.545122796297073,5.4));
#46139=CARTESIAN_POINT('Ctrl Pts',(1.28683517873287,0.545122796297073,5.37));
#46140=CARTESIAN_POINT('Ctrl Pts',(1.28683517873287,0.474965924024582,5.37));
#46141=CARTESIAN_POINT('Ctrl Pts',(1.24218986928463,0.426381343603134,5.37));
#46142=CARTESIAN_POINT('Ctrl Pts',(1.27013967931271,0.620156908035278,5.4));
#46143=CARTESIAN_POINT('Ctrl Pts',(1.27013967931271,0.620156908035278,5.37));
#46144=CARTESIAN_POINT('Ctrl Pts',(1.28683517873287,0.586016410589218,5.4));
#46145=CARTESIAN_POINT('Ctrl Pts',(1.28683517873287,0.586016410589218,5.37));
#46146=CARTESIAN_POINT('Ctrl Pts',(1.28683517873287,0.545122796297073,5.4));
#46147=CARTESIAN_POINT('Ctrl Pts',(1.28683517873287,0.545122796297073,5.37));
#46148=CARTESIAN_POINT('',(1.27013967931271,0.620156908035278,5.4));
#46149=CARTESIAN_POINT('Ctrl Pts',(1.27013967931271,0.620156908035278,5.4));
#46150=CARTESIAN_POINT('Ctrl Pts',(1.28683517873287,0.586016410589218,5.4));
#46151=CARTESIAN_POINT('Ctrl Pts',(1.28683517873287,0.545122796297073,5.4));
#46152=CARTESIAN_POINT('',(1.27013967931271,0.620156908035278,5.37));
#46153=CARTESIAN_POINT('',(1.27013967931271,0.620156908035278,5.4));
#46154=CARTESIAN_POINT('Ctrl Pts',(1.27013967931271,0.620156908035278,5.37));
#46155=CARTESIAN_POINT('Ctrl Pts',(1.28683517873287,0.586016410589218,5.37));
#46156=CARTESIAN_POINT('Ctrl Pts',(1.28683517873287,0.545122796297073,5.37));
#46157=CARTESIAN_POINT('Ctrl Pts',(1.2260575145483,0.673243546485901,5.4));
#46158=CARTESIAN_POINT('Ctrl Pts',(1.2260575145483,0.673243546485901,5.37));
#46159=CARTESIAN_POINT('Ctrl Pts',(1.2534446567297,0.654297435283661,5.4));
#46160=CARTESIAN_POINT('Ctrl Pts',(1.2534446567297,0.654297435283661,5.37));
#46161=CARTESIAN_POINT('Ctrl Pts',(1.27013967931271,0.620156908035278,5.4));
#46162=CARTESIAN_POINT('Ctrl Pts',(1.27013967931271,0.620156908035278,5.37));
#46163=CARTESIAN_POINT('',(1.2260575145483,0.673243546485901,5.4));
#46164=CARTESIAN_POINT('Ctrl Pts',(1.2260575145483,0.673243546485901,5.4));
#46165=CARTESIAN_POINT('Ctrl Pts',(1.2534446567297,0.654297435283661,5.4));
#46166=CARTESIAN_POINT('Ctrl Pts',(1.27013967931271,0.620156908035278,5.4));
#46167=CARTESIAN_POINT('',(1.2260575145483,0.673243546485901,5.37));
#46168=CARTESIAN_POINT('',(1.2260575145483,0.673243546485901,5.4));
#46169=CARTESIAN_POINT('Ctrl Pts',(1.2260575145483,0.673243546485901,5.37));
#46170=CARTESIAN_POINT('Ctrl Pts',(1.2534446567297,0.654297435283661,5.37));
#46171=CARTESIAN_POINT('Ctrl Pts',(1.27013967931271,0.620156908035278,5.37));
#46172=CARTESIAN_POINT('Ctrl Pts',(1.15815161168575,0.698942744731903,5.4));
#46173=CARTESIAN_POINT('Ctrl Pts',(1.15815161168575,0.698942744731903,5.37));
#46174=CARTESIAN_POINT('Ctrl Pts',(1.19866989552975,0.692189657688141,5.4));
#46175=CARTESIAN_POINT('Ctrl Pts',(1.19866989552975,0.692189657688141,5.37));
#46176=CARTESIAN_POINT('Ctrl Pts',(1.2260575145483,0.673243546485901,5.4));
#46177=CARTESIAN_POINT('Ctrl Pts',(1.2260575145483,0.673243546485901,5.37));
#46178=CARTESIAN_POINT('',(1.15815161168575,0.698942744731903,5.4));
#46179=CARTESIAN_POINT('Ctrl Pts',(1.15815161168575,0.698942744731903,5.4));
#46180=CARTESIAN_POINT('Ctrl Pts',(1.19866989552975,0.692189657688141,5.4));
#46181=CARTESIAN_POINT('Ctrl Pts',(1.2260575145483,0.673243546485901,5.4));
#46182=CARTESIAN_POINT('',(1.15815161168575,0.698942744731903,5.37));
#46183=CARTESIAN_POINT('',(1.15815161168575,0.698942744731903,5.4));
#46184=CARTESIAN_POINT('Ctrl Pts',(1.15815161168575,0.698942744731903,5.37));
#46185=CARTESIAN_POINT('Ctrl Pts',(1.19866989552975,0.692189657688141,5.37));
#46186=CARTESIAN_POINT('Ctrl Pts',(1.2260575145483,0.673243546485901,5.37));
#46187=CARTESIAN_POINT('Ctrl Pts',(1.07448862493038,0.704195106029511,5.4));
#46188=CARTESIAN_POINT('Ctrl Pts',(1.07448862493038,0.704195106029511,5.37));
#46189=CARTESIAN_POINT('Ctrl Pts',(1.12926338613033,0.704195106029511,5.4));
#46190=CARTESIAN_POINT('Ctrl Pts',(1.12926338613033,0.704195106029511,5.37));
#46191=CARTESIAN_POINT('Ctrl Pts',(1.15815161168575,0.698942744731903,5.4));
#46192=CARTESIAN_POINT('Ctrl Pts',(1.15815161168575,0.698942744731903,5.37));
#46193=CARTESIAN_POINT('',(1.07448862493038,0.704195106029511,5.4));
#46194=CARTESIAN_POINT('Ctrl Pts',(1.07448862493038,0.704195106029511,5.4));
#46195=CARTESIAN_POINT('Ctrl Pts',(1.12926338613033,0.704195106029511,5.4));
#46196=CARTESIAN_POINT('Ctrl Pts',(1.15815161168575,0.698942744731903,5.4));
#46197=CARTESIAN_POINT('',(1.07448862493038,0.704195106029511,5.37));
#46198=CARTESIAN_POINT('',(1.07448862493038,0.704195106029511,5.4));
#46199=CARTESIAN_POINT('Ctrl Pts',(1.07448862493038,0.704195106029511,5.37));
#46200=CARTESIAN_POINT('Ctrl Pts',(1.12926338613033,0.704195106029511,5.37));
#46201=CARTESIAN_POINT('Ctrl Pts',(1.15815161168575,0.698942744731903,5.37));
#46202=CARTESIAN_POINT('Origin',(0.867019161581993,0.704195106029511,5.4));
#46203=CARTESIAN_POINT('',(0.867019161581993,0.704195106029511,5.4));
#46204=CARTESIAN_POINT('',(0.433509580790997,0.704195106029511,5.4));
#46205=CARTESIAN_POINT('',(0.867019161581993,0.704195106029511,5.37));
#46206=CARTESIAN_POINT('',(0.867019161581993,0.704195106029511,5.4));
#46207=CARTESIAN_POINT('',(0.867019161581993,0.704195106029511,5.37));
#46208=CARTESIAN_POINT('Origin',(0.867019161581993,0.154195094108582,5.4));
#46209=CARTESIAN_POINT('',(0.867019161581993,0.154195094108582,5.4));
#46210=CARTESIAN_POINT('',(0.867019161581993,0.0770975470542908,5.4));
#46211=CARTESIAN_POINT('',(0.867019161581993,0.154195094108582,5.37));
#46212=CARTESIAN_POINT('',(0.867019161581993,0.154195094108582,5.4));
#46213=CARTESIAN_POINT('',(0.867019161581993,0.154195094108582,5.37));
#46214=CARTESIAN_POINT('Origin',(0.939802154898643,0.154195094108582,5.4));
#46215=CARTESIAN_POINT('',(0.939802154898643,0.154195094108582,5.4));
#46216=CARTESIAN_POINT('',(0.469901077449322,0.154195094108582,5.4));
#46217=CARTESIAN_POINT('',(0.939802154898643,0.154195094108582,5.37));
#46218=CARTESIAN_POINT('',(0.939802154898643,0.154195094108582,5.4));
#46219=CARTESIAN_POINT('',(0.939802154898643,0.154195094108582,5.37));
#46220=CARTESIAN_POINT('Origin',(0.939802154898643,0.377796748280525,5.4));
#46221=CARTESIAN_POINT('',(0.939802154898643,0.188898374140263,5.4));
#46222=CARTESIAN_POINT('',(0.939802154898643,0.377796748280525,5.37));
#46223=CARTESIAN_POINT('Origin',(1.07692717015743,0.429195100069046,5.37));
#46224=CARTESIAN_POINT('Ctrl Pts',(2.16323326528072,0.451330178976059,5.4));
#46225=CARTESIAN_POINT('Ctrl Pts',(2.16323326528072,0.451330178976059,5.37));
#46226=CARTESIAN_POINT('Ctrl Pts',(2.11746262013912,0.451330178976059,5.4));
#46227=CARTESIAN_POINT('Ctrl Pts',(2.11746262013912,0.451330178976059,5.37));
#46228=CARTESIAN_POINT('Ctrl Pts',(2.08557318150997,0.418502742052078,5.4));
#46229=CARTESIAN_POINT('Ctrl Pts',(2.08557318150997,0.418502742052078,5.37));
#46230=CARTESIAN_POINT('',(2.16323326528072,0.451330178976059,5.4));
#46231=CARTESIAN_POINT('',(2.08557318150997,0.418502742052078,5.4));
#46232=CARTESIAN_POINT('Ctrl Pts',(2.16323326528072,0.451330178976059,5.4));
#46233=CARTESIAN_POINT('Ctrl Pts',(2.11746262013912,0.451330178976059,5.4));
#46234=CARTESIAN_POINT('Ctrl Pts',(2.08557318150997,0.418502742052078,5.4));
#46235=CARTESIAN_POINT('',(2.16323326528072,0.451330178976059,5.37));
#46236=CARTESIAN_POINT('',(2.16323326528072,0.451330178976059,5.4));
#46237=CARTESIAN_POINT('',(2.08557318150997,0.418502742052078,5.37));
#46238=CARTESIAN_POINT('Ctrl Pts',(2.16323326528072,0.451330178976059,5.37));
#46239=CARTESIAN_POINT('Ctrl Pts',(2.11746262013912,0.451330178976059,5.37));
#46240=CARTESIAN_POINT('Ctrl Pts',(2.08557318150997,0.418502742052078,5.37));
#46241=CARTESIAN_POINT('',(2.08557318150997,0.418502742052078,5.4));
#46242=CARTESIAN_POINT('Ctrl Pts',(2.23976801335812,0.418502742052078,5.4));
#46243=CARTESIAN_POINT('Ctrl Pts',(2.23976801335812,0.418502742052078,5.37));
#46244=CARTESIAN_POINT('Ctrl Pts',(2.20937918126583,0.451330178976059,5.4));
#46245=CARTESIAN_POINT('Ctrl Pts',(2.20937918126583,0.451330178976059,5.37));
#46246=CARTESIAN_POINT('Ctrl Pts',(2.16323326528072,0.451330178976059,5.4));
#46247=CARTESIAN_POINT('Ctrl Pts',(2.16323326528072,0.451330178976059,5.37));
#46248=CARTESIAN_POINT('',(2.23976801335812,0.418502742052078,5.4));
#46249=CARTESIAN_POINT('Ctrl Pts',(2.23976801335812,0.418502742052078,5.4));
#46250=CARTESIAN_POINT('Ctrl Pts',(2.20937918126583,0.451330178976059,5.4));
#46251=CARTESIAN_POINT('Ctrl Pts',(2.16323326528072,0.451330178976059,5.4));
#46252=CARTESIAN_POINT('',(2.23976801335812,0.418502742052078,5.37));
#46253=CARTESIAN_POINT('',(2.23976801335812,0.418502742052078,5.4));
#46254=CARTESIAN_POINT('Ctrl Pts',(2.23976801335812,0.418502742052078,5.37));
#46255=CARTESIAN_POINT('Ctrl Pts',(2.20937918126583,0.451330178976059,5.37));
#46256=CARTESIAN_POINT('Ctrl Pts',(2.16323326528072,0.451330178976059,5.37));
#46257=CARTESIAN_POINT('Ctrl Pts',(2.2701568454504,0.328649395704269,5.4));
#46258=CARTESIAN_POINT('Ctrl Pts',(2.2701568454504,0.328649395704269,5.37));
#46259=CARTESIAN_POINT('Ctrl Pts',(2.2701568454504,0.385675320029259,5.4));
#46260=CARTESIAN_POINT('Ctrl Pts',(2.2701568454504,0.385675320029259,5.37));
#46261=CARTESIAN_POINT('Ctrl Pts',(2.23976801335812,0.418502742052078,5.4));
#46262=CARTESIAN_POINT('Ctrl Pts',(2.23976801335812,0.418502742052078,5.37));
#46263=CARTESIAN_POINT('',(2.2701568454504,0.328649395704269,5.4));
#46264=CARTESIAN_POINT('Ctrl Pts',(2.2701568454504,0.328649395704269,5.4));
#46265=CARTESIAN_POINT('Ctrl Pts',(2.2701568454504,0.385675320029259,5.4));
#46266=CARTESIAN_POINT('Ctrl Pts',(2.23976801335812,0.418502742052078,5.4));
#46267=CARTESIAN_POINT('',(2.2701568454504,0.328649395704269,5.37));
#46268=CARTESIAN_POINT('',(2.2701568454504,0.328649395704269,5.4));
#46269=CARTESIAN_POINT('Ctrl Pts',(2.2701568454504,0.328649395704269,5.37));
#46270=CARTESIAN_POINT('Ctrl Pts',(2.2701568454504,0.385675320029259,5.37));
#46271=CARTESIAN_POINT('Ctrl Pts',(2.23976801335812,0.418502742052078,5.37));
#46272=CARTESIAN_POINT('Ctrl Pts',(2.23939274251461,0.234856748580933,5.4));
#46273=CARTESIAN_POINT('Ctrl Pts',(2.23939274251461,0.234856748580933,5.37));
#46274=CARTESIAN_POINT('Ctrl Pts',(2.2701568454504,0.269372457265854,5.4));
#46275=CARTESIAN_POINT('Ctrl Pts',(2.2701568454504,0.269372457265854,5.37));
#46276=CARTESIAN_POINT('Ctrl Pts',(2.2701568454504,0.328649395704269,5.4));
#46277=CARTESIAN_POINT('Ctrl Pts',(2.2701568454504,0.328649395704269,5.37));
#46278=CARTESIAN_POINT('',(2.23939274251461,0.234856748580933,5.4));
#46279=CARTESIAN_POINT('Ctrl Pts',(2.23939274251461,0.234856748580933,5.4));
#46280=CARTESIAN_POINT('Ctrl Pts',(2.2701568454504,0.269372457265854,5.4));
#46281=CARTESIAN_POINT('Ctrl Pts',(2.2701568454504,0.328649395704269,5.4));
#46282=CARTESIAN_POINT('',(2.23939274251461,0.234856748580933,5.37));
#46283=CARTESIAN_POINT('',(2.23939274251461,0.234856748580933,5.4));
#46284=CARTESIAN_POINT('Ctrl Pts',(2.23939274251461,0.234856748580933,5.37));
#46285=CARTESIAN_POINT('Ctrl Pts',(2.2701568454504,0.269372457265854,5.37));
#46286=CARTESIAN_POINT('Ctrl Pts',(2.2701568454504,0.328649395704269,5.37));
#46287=CARTESIAN_POINT('Ctrl Pts',(2.16585968434811,0.200341069698334,5.4));
#46288=CARTESIAN_POINT('Ctrl Pts',(2.16585968434811,0.200341069698334,5.37));
#46289=CARTESIAN_POINT('Ctrl Pts',(2.20862911641598,0.200341069698334,5.4));
#46290=CARTESIAN_POINT('Ctrl Pts',(2.20862911641598,0.200341069698334,5.37));
#46291=CARTESIAN_POINT('Ctrl Pts',(2.23939274251461,0.234856748580933,5.4));
#46292=CARTESIAN_POINT('Ctrl Pts',(2.23939274251461,0.234856748580933,5.37));
#46293=CARTESIAN_POINT('',(2.16585968434811,0.200341069698334,5.4));
#46294=CARTESIAN_POINT('Ctrl Pts',(2.16585968434811,0.200341069698334,5.4));
#46295=CARTESIAN_POINT('Ctrl Pts',(2.20862911641598,0.200341069698334,5.4));
#46296=CARTESIAN_POINT('Ctrl Pts',(2.23939274251461,0.234856748580933,5.4));
#46297=CARTESIAN_POINT('',(2.16585968434811,0.200341069698334,5.37));
#46298=CARTESIAN_POINT('',(2.16585968434811,0.200341069698334,5.4));
#46299=CARTESIAN_POINT('Ctrl Pts',(2.16585968434811,0.200341069698334,5.37));
#46300=CARTESIAN_POINT('Ctrl Pts',(2.20862911641598,0.200341069698334,5.37));
#46301=CARTESIAN_POINT('Ctrl Pts',(2.23939274251461,0.234856748580933,5.37));
#46302=CARTESIAN_POINT('Ctrl Pts',(2.10995911061764,0.217036151885986,5.4));
#46303=CARTESIAN_POINT('Ctrl Pts',(2.10995911061764,0.217036151885986,5.37));
#46304=CARTESIAN_POINT('Ctrl Pts',(2.13659618794918,0.200341069698334,5.4));
#46305=CARTESIAN_POINT('Ctrl Pts',(2.13659618794918,0.200341069698334,5.37));
#46306=CARTESIAN_POINT('Ctrl Pts',(2.16585968434811,0.200341069698334,5.4));
#46307=CARTESIAN_POINT('Ctrl Pts',(2.16585968434811,0.200341069698334,5.37));
#46308=CARTESIAN_POINT('',(2.10995911061764,0.217036151885986,5.4));
#46309=CARTESIAN_POINT('Ctrl Pts',(2.10995911061764,0.217036151885986,5.4));
#46310=CARTESIAN_POINT('Ctrl Pts',(2.13659618794918,0.200341069698334,5.4));
#46311=CARTESIAN_POINT('Ctrl Pts',(2.16585968434811,0.200341069698334,5.4));
#46312=CARTESIAN_POINT('',(2.10995911061764,0.217036151885986,5.37));
#46313=CARTESIAN_POINT('',(2.10995911061764,0.217036151885986,5.4));
#46314=CARTESIAN_POINT('Ctrl Pts',(2.10995911061764,0.217036151885986,5.37));
#46315=CARTESIAN_POINT('Ctrl Pts',(2.13659618794918,0.200341069698334,5.37));
#46316=CARTESIAN_POINT('Ctrl Pts',(2.16585968434811,0.200341069698334,5.37));
#46317=CARTESIAN_POINT('Ctrl Pts',(2.06850288808346,0.265620732307434,5.4));
#46318=CARTESIAN_POINT('Ctrl Pts',(2.06850288808346,0.265620732307434,5.37));
#46319=CARTESIAN_POINT('Ctrl Pts',(2.08332203328609,0.233731234073639,5.4));
#46320=CARTESIAN_POINT('Ctrl Pts',(2.08332203328609,0.233731234073639,5.37));
#46321=CARTESIAN_POINT('Ctrl Pts',(2.10995911061764,0.217036151885986,5.4));
#46322=CARTESIAN_POINT('Ctrl Pts',(2.10995911061764,0.217036151885986,5.37));
#46323=CARTESIAN_POINT('',(2.06850288808346,0.265620732307434,5.4));
#46324=CARTESIAN_POINT('Ctrl Pts',(2.06850288808346,0.265620732307434,5.4));
#46325=CARTESIAN_POINT('Ctrl Pts',(2.08332203328609,0.233731234073639,5.4));
#46326=CARTESIAN_POINT('Ctrl Pts',(2.10995911061764,0.217036151885986,5.4));
#46327=CARTESIAN_POINT('',(2.06850288808346,0.265620732307434,5.37));
#46328=CARTESIAN_POINT('',(2.06850288808346,0.265620732307434,5.4));
#46329=CARTESIAN_POINT('Ctrl Pts',(2.06850288808346,0.265620732307434,5.37));
#46330=CARTESIAN_POINT('Ctrl Pts',(2.08332203328609,0.233731234073639,5.37));
#46331=CARTESIAN_POINT('Ctrl Pts',(2.10995911061764,0.217036151885986,5.37));
#46332=CARTESIAN_POINT('Ctrl Pts',(2.05368326604366,0.332401105761528,5.4));
#46333=CARTESIAN_POINT('Ctrl Pts',(2.05368326604366,0.332401105761528,5.37));
#46334=CARTESIAN_POINT('Ctrl Pts',(2.05368326604366,0.29751024544239,5.4));
#46335=CARTESIAN_POINT('Ctrl Pts',(2.05368326604366,0.29751024544239,5.37));
#46336=CARTESIAN_POINT('Ctrl Pts',(2.06850288808346,0.265620732307434,5.4));
#46337=CARTESIAN_POINT('Ctrl Pts',(2.06850288808346,0.265620732307434,5.37));
#46338=CARTESIAN_POINT('',(2.05368326604366,0.332401105761528,5.4));
#46339=CARTESIAN_POINT('Ctrl Pts',(2.05368326604366,0.332401105761528,5.4));
#46340=CARTESIAN_POINT('Ctrl Pts',(2.05368326604366,0.29751024544239,5.4));
#46341=CARTESIAN_POINT('Ctrl Pts',(2.06850288808346,0.265620732307434,5.4));
#46342=CARTESIAN_POINT('',(2.05368326604366,0.332401105761528,5.37));
#46343=CARTESIAN_POINT('',(2.05368326604366,0.332401105761528,5.4));
#46344=CARTESIAN_POINT('Ctrl Pts',(2.05368326604366,0.332401105761528,5.37));
#46345=CARTESIAN_POINT('Ctrl Pts',(2.05368326604366,0.29751024544239,5.37));
#46346=CARTESIAN_POINT('Ctrl Pts',(2.06850288808346,0.265620732307434,5.37));
#46347=CARTESIAN_POINT('Ctrl Pts',(2.08557318150997,0.418502742052078,5.4));
#46348=CARTESIAN_POINT('Ctrl Pts',(2.08557318150997,0.418502742052078,5.37));
#46349=CARTESIAN_POINT('Ctrl Pts',(2.05368326604366,0.385675320029259,5.4));
#46350=CARTESIAN_POINT('Ctrl Pts',(2.05368326604366,0.385675320029259,5.37));
#46351=CARTESIAN_POINT('Ctrl Pts',(2.05368326604366,0.332401105761528,5.4));
#46352=CARTESIAN_POINT('Ctrl Pts',(2.05368326604366,0.332401105761528,5.37));
#46353=CARTESIAN_POINT('Ctrl Pts',(2.08557318150997,0.418502742052078,5.4));
#46354=CARTESIAN_POINT('Ctrl Pts',(2.05368326604366,0.385675320029259,5.4));
#46355=CARTESIAN_POINT('Ctrl Pts',(2.05368326604366,0.332401105761528,5.4));
#46356=CARTESIAN_POINT('Ctrl Pts',(2.08557318150997,0.418502742052078,5.37));
#46357=CARTESIAN_POINT('Ctrl Pts',(2.05368326604366,0.385675320029259,5.37));
#46358=CARTESIAN_POINT('Ctrl Pts',(2.05368326604366,0.332401105761528,5.37));
#46359=CARTESIAN_POINT('Ctrl Pts',(2.03492496907711,0.643417501449585,5.4));
#46360=CARTESIAN_POINT('Ctrl Pts',(2.03492496907711,0.643417501449585,5.37));
#46361=CARTESIAN_POINT('Ctrl Pts',(2.08632324635983,0.706446135044098,5.4));
#46362=CARTESIAN_POINT('Ctrl Pts',(2.08632324635983,0.706446135044098,5.37));
#46363=CARTESIAN_POINT('Ctrl Pts',(2.17336271703243,0.706446135044098,5.4));
#46364=CARTESIAN_POINT('Ctrl Pts',(2.17336271703243,0.706446135044098,5.37));
#46365=CARTESIAN_POINT('',(2.03492496907711,0.643417501449585,5.4));
#46366=CARTESIAN_POINT('',(2.17336271703243,0.706446135044098,5.4));
#46367=CARTESIAN_POINT('Ctrl Pts',(2.03492496907711,0.643417501449585,5.4));
#46368=CARTESIAN_POINT('Ctrl Pts',(2.08632324635983,0.706446135044098,5.4));
#46369=CARTESIAN_POINT('Ctrl Pts',(2.17336271703243,0.706446135044098,5.4));
#46370=CARTESIAN_POINT('',(2.03492496907711,0.643417501449585,5.37));
#46371=CARTESIAN_POINT('',(2.03492496907711,0.643417501449585,5.4));
#46372=CARTESIAN_POINT('',(2.17336271703243,0.706446135044098,5.37));
#46373=CARTESIAN_POINT('Ctrl Pts',(2.03492496907711,0.643417501449585,5.37));
#46374=CARTESIAN_POINT('Ctrl Pts',(2.08632324635983,0.706446135044098,5.37));
#46375=CARTESIAN_POINT('Ctrl Pts',(2.17336271703243,0.706446135044098,5.37));
#46376=CARTESIAN_POINT('',(2.17336271703243,0.706446135044098,5.4));
#46377=CARTESIAN_POINT('Ctrl Pts',(1.97602318227291,0.411562079191208,5.4));
#46378=CARTESIAN_POINT('Ctrl Pts',(1.97602318227291,0.411562079191208,5.37));
#46379=CARTESIAN_POINT('Ctrl Pts',(1.97602318227291,0.571009570360184,5.4));
#46380=CARTESIAN_POINT('Ctrl Pts',(1.97602318227291,0.571009570360184,5.37));
#46381=CARTESIAN_POINT('Ctrl Pts',(2.03492496907711,0.643417501449585,5.4));
#46382=CARTESIAN_POINT('Ctrl Pts',(2.03492496907711,0.643417501449585,5.37));
#46383=CARTESIAN_POINT('',(1.97602318227291,0.411562079191208,5.4));
#46384=CARTESIAN_POINT('Ctrl Pts',(1.97602318227291,0.411562079191208,5.4));
#46385=CARTESIAN_POINT('Ctrl Pts',(1.97602318227291,0.571009570360184,5.4));
#46386=CARTESIAN_POINT('Ctrl Pts',(2.03492496907711,0.643417501449585,5.4));
#46387=CARTESIAN_POINT('',(1.97602318227291,0.411562079191208,5.37));
#46388=CARTESIAN_POINT('',(1.97602318227291,0.411562079191208,5.4));
#46389=CARTESIAN_POINT('Ctrl Pts',(1.97602318227291,0.411562079191208,5.37));
#46390=CARTESIAN_POINT('Ctrl Pts',(1.97602318227291,0.571009570360184,5.37));
#46391=CARTESIAN_POINT('Ctrl Pts',(2.03492496907711,0.643417501449585,5.37));
#46392=CARTESIAN_POINT('Ctrl Pts',(2.029297336936,0.206906551122665,5.4));
#46393=CARTESIAN_POINT('Ctrl Pts',(2.029297336936,0.206906551122665,5.37));
#46394=CARTESIAN_POINT('Ctrl Pts',(1.97602318227291,0.268997275829315,5.4));
#46395=CARTESIAN_POINT('Ctrl Pts',(1.97602318227291,0.268997275829315,5.37));
#46396=CARTESIAN_POINT('Ctrl Pts',(1.97602318227291,0.411562079191208,5.4));
#46397=CARTESIAN_POINT('Ctrl Pts',(1.97602318227291,0.411562079191208,5.37));
#46398=CARTESIAN_POINT('',(2.029297336936,0.206906551122665,5.4));
#46399=CARTESIAN_POINT('Ctrl Pts',(2.029297336936,0.206906551122665,5.4));
#46400=CARTESIAN_POINT('Ctrl Pts',(1.97602318227291,0.268997275829315,5.4));
#46401=CARTESIAN_POINT('Ctrl Pts',(1.97602318227291,0.411562079191208,5.4));
#46402=CARTESIAN_POINT('',(2.029297336936,0.206906551122665,5.37));
#46403=CARTESIAN_POINT('',(2.029297336936,0.206906551122665,5.4));
#46404=CARTESIAN_POINT('Ctrl Pts',(2.029297336936,0.206906551122665,5.37));
#46405=CARTESIAN_POINT('Ctrl Pts',(1.97602318227291,0.268997275829315,5.37));
#46406=CARTESIAN_POINT('Ctrl Pts',(1.97602318227291,0.411562079191208,5.37));
#46407=CARTESIAN_POINT('Ctrl Pts',(2.16698502004147,0.144815826416016,5.4));
#46408=CARTESIAN_POINT('Ctrl Pts',(2.16698502004147,0.144815826416016,5.37));
#46409=CARTESIAN_POINT('Ctrl Pts',(2.08257149159908,0.144815826416016,5.4));
#46410=CARTESIAN_POINT('Ctrl Pts',(2.08257149159908,0.144815826416016,5.37));
#46411=CARTESIAN_POINT('Ctrl Pts',(2.029297336936,0.206906551122665,5.4));
#46412=CARTESIAN_POINT('Ctrl Pts',(2.029297336936,0.206906551122665,5.37));
#46413=CARTESIAN_POINT('',(2.16698502004147,0.144815826416016,5.4));
#46414=CARTESIAN_POINT('Ctrl Pts',(2.16698502004147,0.144815826416016,5.4));
#46415=CARTESIAN_POINT('Ctrl Pts',(2.08257149159908,0.144815826416016,5.4));
#46416=CARTESIAN_POINT('Ctrl Pts',(2.029297336936,0.206906551122665,5.4));
#46417=CARTESIAN_POINT('',(2.16698502004147,0.144815826416016,5.37));
#46418=CARTESIAN_POINT('',(2.16698502004147,0.144815826416016,5.4));
#46419=CARTESIAN_POINT('Ctrl Pts',(2.16698502004147,0.144815826416016,5.37));
#46420=CARTESIAN_POINT('Ctrl Pts',(2.08257149159908,0.144815826416016,5.37));
#46421=CARTESIAN_POINT('Ctrl Pts',(2.029297336936,0.206906551122665,5.37));
#46422=CARTESIAN_POINT('Ctrl Pts',(2.25552509725094,0.168451571464539,5.4));
#46423=CARTESIAN_POINT('Ctrl Pts',(2.25552509725094,0.168451571464539,5.37));
#46424=CARTESIAN_POINT('Ctrl Pts',(2.21650741994381,0.144815826416016,5.4));
#46425=CARTESIAN_POINT('Ctrl Pts',(2.21650741994381,0.144815826416016,5.37));
#46426=CARTESIAN_POINT('Ctrl Pts',(2.16698502004147,0.144815826416016,5.4));
#46427=CARTESIAN_POINT('Ctrl Pts',(2.16698502004147,0.144815826416016,5.37));
#46428=CARTESIAN_POINT('',(2.25552509725094,0.168451571464539,5.4));
#46429=CARTESIAN_POINT('Ctrl Pts',(2.25552509725094,0.168451571464539,5.4));
#46430=CARTESIAN_POINT('Ctrl Pts',(2.21650741994381,0.144815826416016,5.4));
#46431=CARTESIAN_POINT('Ctrl Pts',(2.16698502004147,0.144815826416016,5.4));
#46432=CARTESIAN_POINT('',(2.25552509725094,0.168451571464539,5.37));
#46433=CARTESIAN_POINT('',(2.25552509725094,0.168451571464539,5.4));
#46434=CARTESIAN_POINT('Ctrl Pts',(2.25552509725094,0.168451571464539,5.37));
#46435=CARTESIAN_POINT('Ctrl Pts',(2.21650741994381,0.144815826416016,5.37));
#46436=CARTESIAN_POINT('Ctrl Pts',(2.16698502004147,0.144815826416016,5.37));
#46437=CARTESIAN_POINT('Ctrl Pts',(2.31686542928219,0.236545050144196,5.4));
#46438=CARTESIAN_POINT('Ctrl Pts',(2.31686542928219,0.236545050144196,5.37));
#46439=CARTESIAN_POINT('Ctrl Pts',(2.29454277455807,0.192087316513062,5.4));
#46440=CARTESIAN_POINT('Ctrl Pts',(2.29454277455807,0.192087316513062,5.37));
#46441=CARTESIAN_POINT('Ctrl Pts',(2.25552509725094,0.168451571464539,5.4));
#46442=CARTESIAN_POINT('Ctrl Pts',(2.25552509725094,0.168451571464539,5.37));
#46443=CARTESIAN_POINT('',(2.31686542928219,0.236545050144196,5.4));
#46444=CARTESIAN_POINT('Ctrl Pts',(2.31686542928219,0.236545050144196,5.4));
#46445=CARTESIAN_POINT('Ctrl Pts',(2.29454277455807,0.192087316513062,5.4));
#46446=CARTESIAN_POINT('Ctrl Pts',(2.25552509725094,0.168451571464539,5.4));
#46447=CARTESIAN_POINT('',(2.31686542928219,0.236545050144196,5.37));
#46448=CARTESIAN_POINT('',(2.31686542928219,0.236545050144196,5.4));
#46449=CARTESIAN_POINT('Ctrl Pts',(2.31686542928219,0.236545050144196,5.37));
#46450=CARTESIAN_POINT('Ctrl Pts',(2.29454277455807,0.192087316513062,5.37));
#46451=CARTESIAN_POINT('Ctrl Pts',(2.25552509725094,0.168451571464539,5.37));
#46452=CARTESIAN_POINT('Ctrl Pts',(2.33918808400631,0.332776272296906,5.4));
#46453=CARTESIAN_POINT('Ctrl Pts',(2.33918808400631,0.332776272296906,5.37));
#46454=CARTESIAN_POINT('Ctrl Pts',(2.33918808400631,0.281002724170685,5.4));
#46455=CARTESIAN_POINT('Ctrl Pts',(2.33918808400631,0.281002724170685,5.37));
#46456=CARTESIAN_POINT('Ctrl Pts',(2.31686542928219,0.236545050144196,5.4));
#46457=CARTESIAN_POINT('Ctrl Pts',(2.31686542928219,0.236545050144196,5.37));
#46458=CARTESIAN_POINT('',(2.33918808400631,0.332776272296906,5.4));
#46459=CARTESIAN_POINT('Ctrl Pts',(2.33918808400631,0.332776272296906,5.4));
#46460=CARTESIAN_POINT('Ctrl Pts',(2.33918808400631,0.281002724170685,5.4));
#46461=CARTESIAN_POINT('Ctrl Pts',(2.31686542928219,0.236545050144196,5.4));
#46462=CARTESIAN_POINT('',(2.33918808400631,0.332776272296906,5.37));
#46463=CARTESIAN_POINT('',(2.33918808400631,0.332776272296906,5.4));
#46464=CARTESIAN_POINT('Ctrl Pts',(2.33918808400631,0.332776272296906,5.37));
#46465=CARTESIAN_POINT('Ctrl Pts',(2.33918808400631,0.281002724170685,5.37));
#46466=CARTESIAN_POINT('Ctrl Pts',(2.31686542928219,0.236545050144196,5.37));
#46467=CARTESIAN_POINT('Ctrl Pts',(2.29172895848751,0.461272174119949,5.4));
#46468=CARTESIAN_POINT('Ctrl Pts',(2.29172895848751,0.461272174119949,5.37));
#46469=CARTESIAN_POINT('Ctrl Pts',(2.33918808400631,0.411562079191208,5.4));
#46470=CARTESIAN_POINT('Ctrl Pts',(2.33918808400631,0.411562079191208,5.37));
#46471=CARTESIAN_POINT('Ctrl Pts',(2.33918808400631,0.332776272296906,5.4));
#46472=CARTESIAN_POINT('Ctrl Pts',(2.33918808400631,0.332776272296906,5.37));
#46473=CARTESIAN_POINT('',(2.29172895848751,0.461272174119949,5.4));
#46474=CARTESIAN_POINT('Ctrl Pts',(2.29172895848751,0.461272174119949,5.4));
#46475=CARTESIAN_POINT('Ctrl Pts',(2.33918808400631,0.411562079191208,5.4));
#46476=CARTESIAN_POINT('Ctrl Pts',(2.33918808400631,0.332776272296906,5.4));
#46477=CARTESIAN_POINT('',(2.29172895848751,0.461272174119949,5.37));
#46478=CARTESIAN_POINT('',(2.29172895848751,0.461272174119949,5.4));
#46479=CARTESIAN_POINT('Ctrl Pts',(2.29172895848751,0.461272174119949,5.37));
#46480=CARTESIAN_POINT('Ctrl Pts',(2.33918808400631,0.411562079191208,5.37));
#46481=CARTESIAN_POINT('Ctrl Pts',(2.33918808400631,0.332776272296906,5.37));
#46482=CARTESIAN_POINT('Ctrl Pts',(2.17673920094967,0.510982298851013,5.4));
#46483=CARTESIAN_POINT('Ctrl Pts',(2.17673920094967,0.510982298851013,5.37));
#46484=CARTESIAN_POINT('Ctrl Pts',(2.24427030980587,0.510982298851013,5.4));
#46485=CARTESIAN_POINT('Ctrl Pts',(2.24427030980587,0.510982298851013,5.37));
#46486=CARTESIAN_POINT('Ctrl Pts',(2.29172895848751,0.461272174119949,5.4));
#46487=CARTESIAN_POINT('Ctrl Pts',(2.29172895848751,0.461272174119949,5.37));
#46488=CARTESIAN_POINT('',(2.17673920094967,0.510982298851013,5.4));
#46489=CARTESIAN_POINT('Ctrl Pts',(2.17673920094967,0.510982298851013,5.4));
#46490=CARTESIAN_POINT('Ctrl Pts',(2.24427030980587,0.510982298851013,5.4));
#46491=CARTESIAN_POINT('Ctrl Pts',(2.29172895848751,0.461272174119949,5.4));
#46492=CARTESIAN_POINT('',(2.17673920094967,0.510982298851013,5.37));
#46493=CARTESIAN_POINT('',(2.17673920094967,0.510982298851013,5.4));
#46494=CARTESIAN_POINT('Ctrl Pts',(2.17673920094967,0.510982298851013,5.37));
#46495=CARTESIAN_POINT('Ctrl Pts',(2.24427030980587,0.510982298851013,5.37));
#46496=CARTESIAN_POINT('Ctrl Pts',(2.29172895848751,0.461272174119949,5.37));
#46497=CARTESIAN_POINT('Ctrl Pts',(2.10283087193966,0.492974096536636,5.4));
#46498=CARTESIAN_POINT('Ctrl Pts',(2.10283087193966,0.492974096536636,5.37));
#46499=CARTESIAN_POINT('Ctrl Pts',(2.13809679448605,0.510982298851013,5.4));
#46500=CARTESIAN_POINT('Ctrl Pts',(2.13809679448605,0.510982298851013,5.37));
#46501=CARTESIAN_POINT('Ctrl Pts',(2.17673920094967,0.510982298851013,5.4));
#46502=CARTESIAN_POINT('Ctrl Pts',(2.17673920094967,0.510982298851013,5.37));
#46503=CARTESIAN_POINT('',(2.10283087193966,0.492974096536636,5.4));
#46504=CARTESIAN_POINT('Ctrl Pts',(2.10283087193966,0.492974096536636,5.4));
#46505=CARTESIAN_POINT('Ctrl Pts',(2.13809679448605,0.510982298851013,5.4));
#46506=CARTESIAN_POINT('Ctrl Pts',(2.17673920094967,0.510982298851013,5.4));
#46507=CARTESIAN_POINT('',(2.10283087193966,0.492974096536636,5.37));
#46508=CARTESIAN_POINT('',(2.10283087193966,0.492974096536636,5.4));
#46509=CARTESIAN_POINT('Ctrl Pts',(2.10283087193966,0.492974096536636,5.37));
#46510=CARTESIAN_POINT('Ctrl Pts',(2.13809679448605,0.510982298851013,5.37));
#46511=CARTESIAN_POINT('Ctrl Pts',(2.17673920094967,0.510982298851013,5.37));
#46512=CARTESIAN_POINT('Ctrl Pts',(2.04317854344845,0.437824034690857,5.4));
#46513=CARTESIAN_POINT('Ctrl Pts',(2.04317854344845,0.437824034690857,5.37));
#46514=CARTESIAN_POINT('Ctrl Pts',(2.06756494939327,0.474965924024582,5.4));
#46515=CARTESIAN_POINT('Ctrl Pts',(2.06756494939327,0.474965924024582,5.37));
#46516=CARTESIAN_POINT('Ctrl Pts',(2.10283087193966,0.492974096536636,5.4));
#46517=CARTESIAN_POINT('Ctrl Pts',(2.10283087193966,0.492974096536636,5.37));
#46518=CARTESIAN_POINT('',(2.04317854344845,0.437824034690857,5.4));
#46519=CARTESIAN_POINT('Ctrl Pts',(2.04317854344845,0.437824034690857,5.4));
#46520=CARTESIAN_POINT('Ctrl Pts',(2.06756494939327,0.474965924024582,5.4));
#46521=CARTESIAN_POINT('Ctrl Pts',(2.10283087193966,0.492974096536636,5.4));
#46522=CARTESIAN_POINT('',(2.04317854344845,0.437824034690857,5.37));
#46523=CARTESIAN_POINT('',(2.04317854344845,0.437824034690857,5.4));
#46524=CARTESIAN_POINT('Ctrl Pts',(2.04317854344845,0.437824034690857,5.37));
#46525=CARTESIAN_POINT('Ctrl Pts',(2.06756494939327,0.474965924024582,5.37));
#46526=CARTESIAN_POINT('Ctrl Pts',(2.10283087193966,0.492974096536636,5.37));
#46527=CARTESIAN_POINT('Ctrl Pts',(2.06231258809566,0.565006846189499,5.4));
#46528=CARTESIAN_POINT('Ctrl Pts',(2.06231258809566,0.565006846189499,5.37));
#46529=CARTESIAN_POINT('Ctrl Pts',(2.04392908513546,0.520361536741257,5.4));
#46530=CARTESIAN_POINT('Ctrl Pts',(2.04392908513546,0.520361536741257,5.37));
#46531=CARTESIAN_POINT('Ctrl Pts',(2.04317854344845,0.437824034690857,5.4));
#46532=CARTESIAN_POINT('Ctrl Pts',(2.04317854344845,0.437824034690857,5.37));
#46533=CARTESIAN_POINT('',(2.06231258809566,0.565006846189499,5.4));
#46534=CARTESIAN_POINT('Ctrl Pts',(2.06231258809566,0.565006846189499,5.4));
#46535=CARTESIAN_POINT('Ctrl Pts',(2.04392908513546,0.520361536741257,5.4));
#46536=CARTESIAN_POINT('Ctrl Pts',(2.04317854344845,0.437824034690857,5.4));
#46537=CARTESIAN_POINT('',(2.06231258809566,0.565006846189499,5.37));
#46538=CARTESIAN_POINT('',(2.06231258809566,0.565006846189499,5.4));
#46539=CARTESIAN_POINT('Ctrl Pts',(2.06231258809566,0.565006846189499,5.37));
#46540=CARTESIAN_POINT('Ctrl Pts',(2.04392908513546,0.520361536741257,5.37));
#46541=CARTESIAN_POINT('Ctrl Pts',(2.04317854344845,0.437824034690857,5.37));
#46542=CARTESIAN_POINT('Ctrl Pts',(2.11258505284786,0.632912719249725,5.4));
#46543=CARTESIAN_POINT('Ctrl Pts',(2.11258505284786,0.632912719249725,5.37));
#46544=CARTESIAN_POINT('Ctrl Pts',(2.08069561421871,0.609652125835419,5.4));
#46545=CARTESIAN_POINT('Ctrl Pts',(2.08069561421871,0.609652125835419,5.37));
#46546=CARTESIAN_POINT('Ctrl Pts',(2.06231258809566,0.565006846189499,5.4));
#46547=CARTESIAN_POINT('Ctrl Pts',(2.06231258809566,0.565006846189499,5.37));
#46548=CARTESIAN_POINT('',(2.11258505284786,0.632912719249725,5.4));
#46549=CARTESIAN_POINT('Ctrl Pts',(2.11258505284786,0.632912719249725,5.4));
#46550=CARTESIAN_POINT('Ctrl Pts',(2.08069561421871,0.609652125835419,5.4));
#46551=CARTESIAN_POINT('Ctrl Pts',(2.06231258809566,0.565006846189499,5.4));
#46552=CARTESIAN_POINT('',(2.11258505284786,0.632912719249725,5.37));
#46553=CARTESIAN_POINT('',(2.11258505284786,0.632912719249725,5.4));
#46554=CARTESIAN_POINT('Ctrl Pts',(2.11258505284786,0.632912719249725,5.37));
#46555=CARTESIAN_POINT('Ctrl Pts',(2.08069561421871,0.609652125835419,5.37));
#46556=CARTESIAN_POINT('Ctrl Pts',(2.06231258809566,0.565006846189499,5.37));
#46557=CARTESIAN_POINT('Ctrl Pts',(2.16923616826534,0.65092089176178,5.4));
#46558=CARTESIAN_POINT('Ctrl Pts',(2.16923616826534,0.65092089176178,5.37));
#46559=CARTESIAN_POINT('Ctrl Pts',(2.13697145879269,0.65092089176178,5.4));
#46560=CARTESIAN_POINT('Ctrl Pts',(2.13697145879269,0.65092089176178,5.37));
#46561=CARTESIAN_POINT('Ctrl Pts',(2.11258505284786,0.632912719249725,5.4));
#46562=CARTESIAN_POINT('Ctrl Pts',(2.11258505284786,0.632912719249725,5.37));
#46563=CARTESIAN_POINT('',(2.16923616826534,0.65092089176178,5.4));
#46564=CARTESIAN_POINT('Ctrl Pts',(2.16923616826534,0.65092089176178,5.4));
#46565=CARTESIAN_POINT('Ctrl Pts',(2.13697145879269,0.65092089176178,5.4));
#46566=CARTESIAN_POINT('Ctrl Pts',(2.11258505284786,0.632912719249725,5.4));
#46567=CARTESIAN_POINT('',(2.16923616826534,0.65092089176178,5.37));
#46568=CARTESIAN_POINT('',(2.16923616826534,0.65092089176178,5.4));
#46569=CARTESIAN_POINT('Ctrl Pts',(2.16923616826534,0.65092089176178,5.37));
#46570=CARTESIAN_POINT('Ctrl Pts',(2.13697145879269,0.65092089176178,5.37));
#46571=CARTESIAN_POINT('Ctrl Pts',(2.11258505284786,0.632912719249725,5.37));
#46572=CARTESIAN_POINT('Ctrl Pts',(2.23676680028439,0.622032755613327,5.4));
#46573=CARTESIAN_POINT('Ctrl Pts',(2.23676680028439,0.622032755613327,5.37));
#46574=CARTESIAN_POINT('Ctrl Pts',(2.20937918126583,0.65092089176178,5.4));
#46575=CARTESIAN_POINT('Ctrl Pts',(2.20937918126583,0.65092089176178,5.37));
#46576=CARTESIAN_POINT('Ctrl Pts',(2.16923616826534,0.65092089176178,5.4));
#46577=CARTESIAN_POINT('Ctrl Pts',(2.16923616826534,0.65092089176178,5.37));
#46578=CARTESIAN_POINT('',(2.23676680028439,0.622032755613327,5.4));
#46579=CARTESIAN_POINT('Ctrl Pts',(2.23676680028439,0.622032755613327,5.4));
#46580=CARTESIAN_POINT('Ctrl Pts',(2.20937918126583,0.65092089176178,5.4));
#46581=CARTESIAN_POINT('Ctrl Pts',(2.16923616826534,0.65092089176178,5.4));
#46582=CARTESIAN_POINT('',(2.23676680028439,0.622032755613327,5.37));
#46583=CARTESIAN_POINT('',(2.23676680028439,0.622032755613327,5.4));
#46584=CARTESIAN_POINT('Ctrl Pts',(2.23676680028439,0.622032755613327,5.37));
#46585=CARTESIAN_POINT('Ctrl Pts',(2.20937918126583,0.65092089176178,5.37));
#46586=CARTESIAN_POINT('Ctrl Pts',(2.16923616826534,0.65092089176178,5.37));
#46587=CARTESIAN_POINT('Ctrl Pts',(2.26227854192257,0.564256513118744,5.4));
#46588=CARTESIAN_POINT('Ctrl Pts',(2.26227854192257,0.564256513118744,5.37));
#46589=CARTESIAN_POINT('Ctrl Pts',(2.25327442586422,0.604024583101273,5.4));
#46590=CARTESIAN_POINT('Ctrl Pts',(2.25327442586422,0.604024583101273,5.37));
#46591=CARTESIAN_POINT('Ctrl Pts',(2.23676680028439,0.622032755613327,5.4));
#46592=CARTESIAN_POINT('Ctrl Pts',(2.23676680028439,0.622032755613327,5.37));
#46593=CARTESIAN_POINT('',(2.26227854192257,0.564256513118744,5.4));
#46594=CARTESIAN_POINT('Ctrl Pts',(2.26227854192257,0.564256513118744,5.4));
#46595=CARTESIAN_POINT('Ctrl Pts',(2.25327442586422,0.604024583101273,5.4));
#46596=CARTESIAN_POINT('Ctrl Pts',(2.23676680028439,0.622032755613327,5.4));
#46597=CARTESIAN_POINT('',(2.26227854192257,0.564256513118744,5.37));
#46598=CARTESIAN_POINT('',(2.26227854192257,0.564256513118744,5.4));
#46599=CARTESIAN_POINT('Ctrl Pts',(2.26227854192257,0.564256513118744,5.37));
#46600=CARTESIAN_POINT('Ctrl Pts',(2.25327442586422,0.604024583101273,5.37));
#46601=CARTESIAN_POINT('Ctrl Pts',(2.23676680028439,0.622032755613327,5.37));
#46602=CARTESIAN_POINT('Origin',(2.32943390309811,0.569508904218674,5.4));
#46603=CARTESIAN_POINT('',(2.32943390309811,0.569508904218674,5.4));
#46604=CARTESIAN_POINT('',(1.14966248238161,0.477235989567443,5.4));
#46605=CARTESIAN_POINT('',(2.32943390309811,0.569508904218674,5.37));
#46606=CARTESIAN_POINT('',(2.32943390309811,0.569508904218674,5.4));
#46607=CARTESIAN_POINT('',(2.32943390309811,0.569508904218674,5.37));
#46608=CARTESIAN_POINT('Ctrl Pts',(2.27972362935543,0.670054578781128,5.4));
#46609=CARTESIAN_POINT('Ctrl Pts',(2.27972362935543,0.670054578781128,5.37));
#46610=CARTESIAN_POINT('Ctrl Pts',(2.32118032872677,0.63366305232048,5.4));
#46611=CARTESIAN_POINT('Ctrl Pts',(2.32118032872677,0.63366305232048,5.37));
#46612=CARTESIAN_POINT('Ctrl Pts',(2.32943390309811,0.569508904218674,5.4));
#46613=CARTESIAN_POINT('Ctrl Pts',(2.32943390309811,0.569508904218674,5.37));
#46614=CARTESIAN_POINT('',(2.27972362935543,0.670054578781128,5.4));
#46615=CARTESIAN_POINT('Ctrl Pts',(2.27972362935543,0.670054578781128,5.4));
#46616=CARTESIAN_POINT('Ctrl Pts',(2.32118032872677,0.63366305232048,5.4));
#46617=CARTESIAN_POINT('Ctrl Pts',(2.32943390309811,0.569508904218674,5.4));
#46618=CARTESIAN_POINT('',(2.27972362935543,0.670054578781128,5.37));
#46619=CARTESIAN_POINT('',(2.27972362935543,0.670054578781128,5.4));
#46620=CARTESIAN_POINT('Ctrl Pts',(2.27972362935543,0.670054578781128,5.37));
#46621=CARTESIAN_POINT('Ctrl Pts',(2.32118032872677,0.63366305232048,5.37));
#46622=CARTESIAN_POINT('Ctrl Pts',(2.32943390309811,0.569508904218674,5.37));
#46623=CARTESIAN_POINT('Ctrl Pts',(2.17336271703243,0.706446135044098,5.4));
#46624=CARTESIAN_POINT('Ctrl Pts',(2.17336271703243,0.706446135044098,5.37));
#46625=CARTESIAN_POINT('Ctrl Pts',(2.23826740682125,0.706446135044098,5.4));
#46626=CARTESIAN_POINT('Ctrl Pts',(2.23826740682125,0.706446135044098,5.37));
#46627=CARTESIAN_POINT('Ctrl Pts',(2.27972362935543,0.670054578781128,5.4));
#46628=CARTESIAN_POINT('Ctrl Pts',(2.27972362935543,0.670054578781128,5.37));
#46629=CARTESIAN_POINT('Ctrl Pts',(2.17336271703243,0.706446135044098,5.4));
#46630=CARTESIAN_POINT('Ctrl Pts',(2.23826740682125,0.706446135044098,5.4));
#46631=CARTESIAN_POINT('Ctrl Pts',(2.27972362935543,0.670054578781128,5.4));
#46632=CARTESIAN_POINT('Ctrl Pts',(2.17336271703243,0.706446135044098,5.37));
#46633=CARTESIAN_POINT('Ctrl Pts',(2.23826740682125,0.706446135044098,5.37));
#46634=CARTESIAN_POINT('Ctrl Pts',(2.27972362935543,0.670054578781128,5.37));
#46635=CARTESIAN_POINT('Origin',(2.15760563313961,0.425630980730057,5.37));
#46636=CARTESIAN_POINT('Ctrl Pts',(-0.344406619668007,-0.352285182476044,
5.4));
#46637=CARTESIAN_POINT('Ctrl Pts',(-0.344406619668007,-0.352285182476044,
5.37));
#46638=CARTESIAN_POINT('Ctrl Pts',(-0.388676658272743,-0.352285182476044,
5.4));
#46639=CARTESIAN_POINT('Ctrl Pts',(-0.388676658272743,-0.352285182476044,
5.37));
#46640=CARTESIAN_POINT('Ctrl Pts',(-0.420941367745399,-0.390740191936493,
5.4));
#46641=CARTESIAN_POINT('Ctrl Pts',(-0.420941367745399,-0.390740191936493,
5.37));
#46642=CARTESIAN_POINT('',(-0.344406619668007,-0.352285182476044,5.4));
#46643=CARTESIAN_POINT('',(-0.420941367745399,-0.390740191936493,5.4));
#46644=CARTESIAN_POINT('Ctrl Pts',(-0.344406619668007,-0.352285182476044,
5.4));
#46645=CARTESIAN_POINT('Ctrl Pts',(-0.388676658272743,-0.352285182476044,
5.4));
#46646=CARTESIAN_POINT('Ctrl Pts',(-0.420941367745399,-0.390740191936493,
5.4));
#46647=CARTESIAN_POINT('',(-0.344406619668007,-0.352285182476044,5.37));
#46648=CARTESIAN_POINT('',(-0.344406619668007,-0.352285182476044,5.4));
#46649=CARTESIAN_POINT('',(-0.420941367745399,-0.390740191936493,5.37));
#46650=CARTESIAN_POINT('Ctrl Pts',(-0.344406619668007,-0.352285182476044,
5.37));
#46651=CARTESIAN_POINT('Ctrl Pts',(-0.388676658272743,-0.352285182476044,
5.37));
#46652=CARTESIAN_POINT('Ctrl Pts',(-0.420941367745399,-0.390740191936493,
5.37));
#46653=CARTESIAN_POINT('',(-0.420941367745399,-0.390740191936493,5.4));
#46654=CARTESIAN_POINT('Ctrl Pts',(-0.269560113549232,-0.389427101612091,
5.4));
#46655=CARTESIAN_POINT('Ctrl Pts',(-0.269560113549232,-0.389427101612091,
5.37));
#46656=CARTESIAN_POINT('Ctrl Pts',(-0.300511613488197,-0.352285182476044,
5.4));
#46657=CARTESIAN_POINT('Ctrl Pts',(-0.300511613488197,-0.352285182476044,
5.37));
#46658=CARTESIAN_POINT('Ctrl Pts',(-0.344406619668007,-0.352285182476044,
5.4));
#46659=CARTESIAN_POINT('Ctrl Pts',(-0.344406619668007,-0.352285182476044,
5.37));
#46660=CARTESIAN_POINT('',(-0.269560113549232,-0.389427101612091,5.4));
#46661=CARTESIAN_POINT('Ctrl Pts',(-0.269560113549232,-0.389427101612091,
5.4));
#46662=CARTESIAN_POINT('Ctrl Pts',(-0.300511613488197,-0.352285182476044,
5.4));
#46663=CARTESIAN_POINT('Ctrl Pts',(-0.344406619668007,-0.352285182476044,
5.4));
#46664=CARTESIAN_POINT('',(-0.269560113549232,-0.389427101612091,5.37));
#46665=CARTESIAN_POINT('',(-0.269560113549232,-0.389427101612091,5.4));
#46666=CARTESIAN_POINT('Ctrl Pts',(-0.269560113549232,-0.389427101612091,
5.37));
#46667=CARTESIAN_POINT('Ctrl Pts',(-0.300511613488197,-0.352285182476044,
5.37));
#46668=CARTESIAN_POINT('Ctrl Pts',(-0.344406619668007,-0.352285182476044,
5.37));
#46669=CARTESIAN_POINT('Ctrl Pts',(-0.238608375191689,-0.504604494571686,
5.4));
#46670=CARTESIAN_POINT('Ctrl Pts',(-0.238608375191689,-0.504604494571686,
5.37));
#46671=CARTESIAN_POINT('Ctrl Pts',(-0.238608375191689,-0.426568961143494,
5.4));
#46672=CARTESIAN_POINT('Ctrl Pts',(-0.238608375191689,-0.426568961143494,
5.37));
#46673=CARTESIAN_POINT('Ctrl Pts',(-0.269560113549232,-0.389427101612091,
5.4));
#46674=CARTESIAN_POINT('Ctrl Pts',(-0.269560113549232,-0.389427101612091,
5.37));
#46675=CARTESIAN_POINT('',(-0.238608375191689,-0.504604494571686,5.4));
#46676=CARTESIAN_POINT('Ctrl Pts',(-0.238608375191689,-0.504604494571686,
5.4));
#46677=CARTESIAN_POINT('Ctrl Pts',(-0.238608375191689,-0.426568961143494,
5.4));
#46678=CARTESIAN_POINT('Ctrl Pts',(-0.269560113549232,-0.389427101612091,
5.4));
#46679=CARTESIAN_POINT('',(-0.238608375191689,-0.504604494571686,5.37));
#46680=CARTESIAN_POINT('',(-0.238608375191689,-0.504604494571686,5.4));
#46681=CARTESIAN_POINT('Ctrl Pts',(-0.238608375191689,-0.504604494571686,
5.37));
#46682=CARTESIAN_POINT('Ctrl Pts',(-0.238608375191689,-0.426568961143494,
5.37));
#46683=CARTESIAN_POINT('Ctrl Pts',(-0.269560113549232,-0.389427101612091,
5.37));
#46684=CARTESIAN_POINT('Ctrl Pts',(-0.270873084664345,-0.619219100475311,
5.4));
#46685=CARTESIAN_POINT('Ctrl Pts',(-0.270873084664345,-0.619219100475311,
5.37));
#46686=CARTESIAN_POINT('Ctrl Pts',(-0.238608375191689,-0.580764091014862,
5.4));
#46687=CARTESIAN_POINT('Ctrl Pts',(-0.238608375191689,-0.580764091014862,
5.37));
#46688=CARTESIAN_POINT('Ctrl Pts',(-0.238608375191689,-0.504604494571686,
5.4));
#46689=CARTESIAN_POINT('Ctrl Pts',(-0.238608375191689,-0.504604494571686,
5.37));
#46690=CARTESIAN_POINT('',(-0.270873084664345,-0.619219100475311,5.4));
#46691=CARTESIAN_POINT('Ctrl Pts',(-0.270873084664345,-0.619219100475311,
5.4));
#46692=CARTESIAN_POINT('Ctrl Pts',(-0.238608375191689,-0.580764091014862,
5.4));
#46693=CARTESIAN_POINT('Ctrl Pts',(-0.238608375191689,-0.504604494571686,
5.4));
#46694=CARTESIAN_POINT('',(-0.270873084664345,-0.619219100475311,5.37));
#46695=CARTESIAN_POINT('',(-0.270873084664345,-0.619219100475311,5.4));
#46696=CARTESIAN_POINT('Ctrl Pts',(-0.270873084664345,-0.619219100475311,
5.37));
#46697=CARTESIAN_POINT('Ctrl Pts',(-0.238608375191689,-0.580764091014862,
5.37));
#46698=CARTESIAN_POINT('Ctrl Pts',(-0.238608375191689,-0.504604494571686,
5.37));
#46699=CARTESIAN_POINT('Ctrl Pts',(-0.347407832741737,-0.657673990726471,
5.4));
#46700=CARTESIAN_POINT('Ctrl Pts',(-0.347407832741737,-0.657673990726471,
5.37));
#46701=CARTESIAN_POINT('Ctrl Pts',(-0.303137794137001,-0.657673990726471,
5.4));
#46702=CARTESIAN_POINT('Ctrl Pts',(-0.303137794137001,-0.657673990726471,
5.37));
#46703=CARTESIAN_POINT('Ctrl Pts',(-0.270873084664345,-0.619219100475311,
5.4));
#46704=CARTESIAN_POINT('Ctrl Pts',(-0.270873084664345,-0.619219100475311,
5.37));
#46705=CARTESIAN_POINT('',(-0.347407832741737,-0.657673990726471,5.4));
#46706=CARTESIAN_POINT('Ctrl Pts',(-0.347407832741737,-0.657673990726471,
5.4));
#46707=CARTESIAN_POINT('Ctrl Pts',(-0.303137794137001,-0.657673990726471,
5.4));
#46708=CARTESIAN_POINT('Ctrl Pts',(-0.270873084664345,-0.619219100475311,
5.4));
#46709=CARTESIAN_POINT('',(-0.347407832741737,-0.657673990726471,5.37));
#46710=CARTESIAN_POINT('',(-0.347407832741737,-0.657673990726471,5.4));
#46711=CARTESIAN_POINT('Ctrl Pts',(-0.347407832741737,-0.657673990726471,
5.37));
#46712=CARTESIAN_POINT('Ctrl Pts',(-0.303137794137001,-0.657673990726471,
5.37));
#46713=CARTESIAN_POINT('Ctrl Pts',(-0.270873084664345,-0.619219100475311,
5.37));
#46714=CARTESIAN_POINT('Ctrl Pts',(-0.433697238564491,-0.605525290966034,
5.4));
#46715=CARTESIAN_POINT('Ctrl Pts',(-0.433697238564491,-0.605525290966034,
5.37));
#46716=CARTESIAN_POINT('Ctrl Pts',(-0.401807561516762,-0.657673990726471,
5.4));
#46717=CARTESIAN_POINT('Ctrl Pts',(-0.401807561516762,-0.657673990726471,
5.37));
#46718=CARTESIAN_POINT('Ctrl Pts',(-0.347407832741737,-0.657673990726471,
5.4));
#46719=CARTESIAN_POINT('Ctrl Pts',(-0.347407832741737,-0.657673990726471,
5.37));
#46720=CARTESIAN_POINT('',(-0.433697238564491,-0.605525290966034,5.4));
#46721=CARTESIAN_POINT('Ctrl Pts',(-0.433697238564491,-0.605525290966034,
5.4));
#46722=CARTESIAN_POINT('Ctrl Pts',(-0.401807561516762,-0.657673990726471,
5.4));
#46723=CARTESIAN_POINT('Ctrl Pts',(-0.347407832741737,-0.657673990726471,
5.4));
#46724=CARTESIAN_POINT('',(-0.433697238564491,-0.605525290966034,5.37));
#46725=CARTESIAN_POINT('',(-0.433697238564491,-0.605525290966034,5.4));
#46726=CARTESIAN_POINT('Ctrl Pts',(-0.433697238564491,-0.605525290966034,
5.37));
#46727=CARTESIAN_POINT('Ctrl Pts',(-0.401807561516762,-0.657673990726471,
5.37));
#46728=CARTESIAN_POINT('Ctrl Pts',(-0.347407832741737,-0.657673990726471,
5.37));
#46729=CARTESIAN_POINT('Ctrl Pts',(-0.453206077218056,-0.501978313922882,
5.4));
#46730=CARTESIAN_POINT('Ctrl Pts',(-0.453206077218056,-0.501978313922882,
5.37));
#46731=CARTESIAN_POINT('Ctrl Pts',(-0.453206077218056,-0.573635852336884,
5.4));
#46732=CARTESIAN_POINT('Ctrl Pts',(-0.453206077218056,-0.573635852336884,
5.37));
#46733=CARTESIAN_POINT('Ctrl Pts',(-0.433697238564491,-0.605525290966034,
5.4));
#46734=CARTESIAN_POINT('Ctrl Pts',(-0.433697238564491,-0.605525290966034,
5.37));
#46735=CARTESIAN_POINT('',(-0.453206077218056,-0.501978313922882,5.4));
#46736=CARTESIAN_POINT('Ctrl Pts',(-0.453206077218056,-0.501978313922882,
5.4));
#46737=CARTESIAN_POINT('Ctrl Pts',(-0.453206077218056,-0.573635852336884,
5.4));
#46738=CARTESIAN_POINT('Ctrl Pts',(-0.433697238564491,-0.605525290966034,
5.4));
#46739=CARTESIAN_POINT('',(-0.453206077218056,-0.501978313922882,5.37));
#46740=CARTESIAN_POINT('',(-0.453206077218056,-0.501978313922882,5.4));
#46741=CARTESIAN_POINT('Ctrl Pts',(-0.453206077218056,-0.501978313922882,
5.37));
#46742=CARTESIAN_POINT('Ctrl Pts',(-0.453206077218056,-0.573635852336884,
5.37));
#46743=CARTESIAN_POINT('Ctrl Pts',(-0.433697238564491,-0.605525290966034,
5.37));
#46744=CARTESIAN_POINT('Ctrl Pts',(-0.420941367745399,-0.390740191936493,
5.4));
#46745=CARTESIAN_POINT('Ctrl Pts',(-0.420941367745399,-0.390740191936493,
5.37));
#46746=CARTESIAN_POINT('Ctrl Pts',(-0.453206077218056,-0.429195141792297,
5.4));
#46747=CARTESIAN_POINT('Ctrl Pts',(-0.453206077218056,-0.429195141792297,
5.37));
#46748=CARTESIAN_POINT('Ctrl Pts',(-0.453206077218056,-0.501978313922882,
5.4));
#46749=CARTESIAN_POINT('Ctrl Pts',(-0.453206077218056,-0.501978313922882,
5.37));
#46750=CARTESIAN_POINT('Ctrl Pts',(-0.420941367745399,-0.390740191936493,
5.4));
#46751=CARTESIAN_POINT('Ctrl Pts',(-0.453206077218056,-0.429195141792297,
5.4));
#46752=CARTESIAN_POINT('Ctrl Pts',(-0.453206077218056,-0.501978313922882,
5.4));
#46753=CARTESIAN_POINT('Ctrl Pts',(-0.420941367745399,-0.390740191936493,
5.37));
#46754=CARTESIAN_POINT('Ctrl Pts',(-0.453206077218056,-0.429195141792297,
5.37));
#46755=CARTESIAN_POINT('Ctrl Pts',(-0.453206077218056,-0.501978313922882,
5.37));
#46756=CARTESIAN_POINT('Ctrl Pts',(-0.220225110650063,-0.657298839092255,
5.4));
#46757=CARTESIAN_POINT('Ctrl Pts',(-0.220225110650063,-0.657298839092255,
5.37));
#46758=CARTESIAN_POINT('Ctrl Pts',(-0.270873084664345,-0.713199293613434,
5.4));
#46759=CARTESIAN_POINT('Ctrl Pts',(-0.270873084664345,-0.713199293613434,
5.37));
#46760=CARTESIAN_POINT('Ctrl Pts',(-0.341780439019203,-0.713199293613434,
5.4));
#46761=CARTESIAN_POINT('Ctrl Pts',(-0.341780439019203,-0.713199293613434,
5.37));
#46762=CARTESIAN_POINT('',(-0.220225110650063,-0.657298839092255,5.4));
#46763=CARTESIAN_POINT('',(-0.341780439019203,-0.713199293613434,5.4));
#46764=CARTESIAN_POINT('Ctrl Pts',(-0.220225110650063,-0.657298839092255,
5.4));
#46765=CARTESIAN_POINT('Ctrl Pts',(-0.270873084664345,-0.713199293613434,
5.4));
#46766=CARTESIAN_POINT('Ctrl Pts',(-0.341780439019203,-0.713199293613434,
5.4));
#46767=CARTESIAN_POINT('',(-0.220225110650063,-0.657298839092255,5.37));
#46768=CARTESIAN_POINT('',(-0.220225110650063,-0.657298839092255,5.4));
#46769=CARTESIAN_POINT('',(-0.341780439019203,-0.713199293613434,5.37));
#46770=CARTESIAN_POINT('Ctrl Pts',(-0.220225110650063,-0.657298839092255,
5.37));
#46771=CARTESIAN_POINT('Ctrl Pts',(-0.270873084664345,-0.713199293613434,
5.37));
#46772=CARTESIAN_POINT('Ctrl Pts',(-0.341780439019203,-0.713199293613434,
5.37));
#46773=CARTESIAN_POINT('',(-0.341780439019203,-0.713199293613434,5.4));
#46774=CARTESIAN_POINT('Ctrl Pts',(-0.16957713663578,-0.498976862430572,
5.4));
#46775=CARTESIAN_POINT('Ctrl Pts',(-0.16957713663578,-0.498976862430572,
5.37));
#46776=CARTESIAN_POINT('Ctrl Pts',(-0.16957713663578,-0.601398384571075,
5.4));
#46777=CARTESIAN_POINT('Ctrl Pts',(-0.16957713663578,-0.601398384571075,
5.37));
#46778=CARTESIAN_POINT('Ctrl Pts',(-0.220225110650063,-0.657298839092255,
5.4));
#46779=CARTESIAN_POINT('Ctrl Pts',(-0.220225110650063,-0.657298839092255,
5.37));
#46780=CARTESIAN_POINT('',(-0.16957713663578,-0.498976862430572,5.4));
#46781=CARTESIAN_POINT('Ctrl Pts',(-0.16957713663578,-0.498976862430572,
5.4));
#46782=CARTESIAN_POINT('Ctrl Pts',(-0.16957713663578,-0.601398384571075,
5.4));
#46783=CARTESIAN_POINT('Ctrl Pts',(-0.220225110650063,-0.657298839092255,
5.4));
#46784=CARTESIAN_POINT('',(-0.16957713663578,-0.498976862430572,5.37));
#46785=CARTESIAN_POINT('',(-0.16957713663578,-0.498976862430572,5.4));
#46786=CARTESIAN_POINT('Ctrl Pts',(-0.16957713663578,-0.498976862430572,
5.37));
#46787=CARTESIAN_POINT('Ctrl Pts',(-0.16957713663578,-0.601398384571075,
5.37));
#46788=CARTESIAN_POINT('Ctrl Pts',(-0.220225110650063,-0.657298839092255,
5.37));
#46789=CARTESIAN_POINT('Ctrl Pts',(-0.18158246576786,-0.417940056324005,
5.4));
#46790=CARTESIAN_POINT('Ctrl Pts',(-0.18158246576786,-0.417940056324005,
5.37));
#46791=CARTESIAN_POINT('Ctrl Pts',(-0.16957713663578,-0.455832278728485,
5.4));
#46792=CARTESIAN_POINT('Ctrl Pts',(-0.16957713663578,-0.455832278728485,
5.37));
#46793=CARTESIAN_POINT('Ctrl Pts',(-0.16957713663578,-0.498976862430572,
5.4));
#46794=CARTESIAN_POINT('Ctrl Pts',(-0.16957713663578,-0.498976862430572,
5.37));
#46795=CARTESIAN_POINT('',(-0.18158246576786,-0.417940056324005,5.4));
#46796=CARTESIAN_POINT('Ctrl Pts',(-0.18158246576786,-0.417940056324005,
5.4));
#46797=CARTESIAN_POINT('Ctrl Pts',(-0.16957713663578,-0.455832278728485,
5.4));
#46798=CARTESIAN_POINT('Ctrl Pts',(-0.16957713663578,-0.498976862430572,
5.4));
#46799=CARTESIAN_POINT('',(-0.18158246576786,-0.417940056324005,5.37));
#46800=CARTESIAN_POINT('',(-0.18158246576786,-0.417940056324005,5.4));
#46801=CARTESIAN_POINT('Ctrl Pts',(-0.18158246576786,-0.417940056324005,
5.37));
#46802=CARTESIAN_POINT('Ctrl Pts',(-0.16957713663578,-0.455832278728485,
5.37));
#46803=CARTESIAN_POINT('Ctrl Pts',(-0.16957713663578,-0.498976862430572,
5.37));
#46804=CARTESIAN_POINT('Ctrl Pts',(-0.214785113930702,-0.353223121166229,
5.4));
#46805=CARTESIAN_POINT('Ctrl Pts',(-0.214785113930702,-0.353223121166229,
5.37));
#46806=CARTESIAN_POINT('Ctrl Pts',(-0.19358803331852,-0.380047833919525,
5.4));
#46807=CARTESIAN_POINT('Ctrl Pts',(-0.19358803331852,-0.380047833919525,
5.37));
#46808=CARTESIAN_POINT('Ctrl Pts',(-0.18158246576786,-0.417940056324005,
5.4));
#46809=CARTESIAN_POINT('Ctrl Pts',(-0.18158246576786,-0.417940056324005,
5.37));
#46810=CARTESIAN_POINT('',(-0.214785113930702,-0.353223121166229,5.4));
#46811=CARTESIAN_POINT('Ctrl Pts',(-0.214785113930702,-0.353223121166229,
5.4));
#46812=CARTESIAN_POINT('Ctrl Pts',(-0.19358803331852,-0.380047833919525,
5.4));
#46813=CARTESIAN_POINT('Ctrl Pts',(-0.18158246576786,-0.417940056324005,
5.4));
#46814=CARTESIAN_POINT('',(-0.214785113930702,-0.353223121166229,5.37));
#46815=CARTESIAN_POINT('',(-0.214785113930702,-0.353223121166229,5.4));
#46816=CARTESIAN_POINT('Ctrl Pts',(-0.214785113930702,-0.353223121166229,
5.37));
#46817=CARTESIAN_POINT('Ctrl Pts',(-0.19358803331852,-0.380047833919525,
5.37));
#46818=CARTESIAN_POINT('Ctrl Pts',(-0.18158246576786,-0.417940056324005,
5.37));
#46819=CARTESIAN_POINT('Ctrl Pts',(-0.2688098102808,-0.311579144001007,
5.4));
#46820=CARTESIAN_POINT('Ctrl Pts',(-0.2688098102808,-0.311579144001007,
5.37));
#46821=CARTESIAN_POINT('Ctrl Pts',(-0.235982194542885,-0.326398408412933,
5.4));
#46822=CARTESIAN_POINT('Ctrl Pts',(-0.235982194542885,-0.326398408412933,
5.37));
#46823=CARTESIAN_POINT('Ctrl Pts',(-0.214785113930702,-0.353223121166229,
5.4));
#46824=CARTESIAN_POINT('Ctrl Pts',(-0.214785113930702,-0.353223121166229,
5.37));
#46825=CARTESIAN_POINT('',(-0.2688098102808,-0.311579144001007,5.4));
#46826=CARTESIAN_POINT('Ctrl Pts',(-0.2688098102808,-0.311579144001007,
5.4));
#46827=CARTESIAN_POINT('Ctrl Pts',(-0.235982194542885,-0.326398408412933,
5.4));
#46828=CARTESIAN_POINT('Ctrl Pts',(-0.214785113930702,-0.353223121166229,
5.4));
#46829=CARTESIAN_POINT('',(-0.2688098102808,-0.311579144001007,5.37));
#46830=CARTESIAN_POINT('',(-0.2688098102808,-0.311579144001007,5.4));
#46831=CARTESIAN_POINT('Ctrl Pts',(-0.2688098102808,-0.311579144001007,
5.37));
#46832=CARTESIAN_POINT('Ctrl Pts',(-0.235982194542885,-0.326398408412933,
5.37));
#46833=CARTESIAN_POINT('Ctrl Pts',(-0.214785113930702,-0.353223121166229,
5.37));
#46834=CARTESIAN_POINT('Ctrl Pts',(-0.338403716683388,-0.296759939193726,
5.4));
#46835=CARTESIAN_POINT('Ctrl Pts',(-0.338403716683388,-0.296759939193726,
5.37));
#46836=CARTESIAN_POINT('Ctrl Pts',(-0.301637187600136,-0.296759939193726,
5.4));
#46837=CARTESIAN_POINT('Ctrl Pts',(-0.301637187600136,-0.296759939193726,
5.37));
#46838=CARTESIAN_POINT('Ctrl Pts',(-0.2688098102808,-0.311579144001007,
5.4));
#46839=CARTESIAN_POINT('Ctrl Pts',(-0.2688098102808,-0.311579144001007,
5.37));
#46840=CARTESIAN_POINT('',(-0.338403716683388,-0.296759939193726,5.4));
#46841=CARTESIAN_POINT('Ctrl Pts',(-0.338403716683388,-0.296759939193726,
5.4));
#46842=CARTESIAN_POINT('Ctrl Pts',(-0.301637187600136,-0.296759939193726,
5.4));
#46843=CARTESIAN_POINT('Ctrl Pts',(-0.2688098102808,-0.311579144001007,
5.4));
#46844=CARTESIAN_POINT('',(-0.338403716683388,-0.296759939193726,5.37));
#46845=CARTESIAN_POINT('',(-0.338403716683388,-0.296759939193726,5.4));
#46846=CARTESIAN_POINT('Ctrl Pts',(-0.338403716683388,-0.296759939193726,
5.37));
#46847=CARTESIAN_POINT('Ctrl Pts',(-0.301637187600136,-0.296759939193726,
5.37));
#46848=CARTESIAN_POINT('Ctrl Pts',(-0.2688098102808,-0.311579144001007,
5.37));
#46849=CARTESIAN_POINT('Ctrl Pts',(-0.447578445076942,-0.350409305095673,
5.4));
#46850=CARTESIAN_POINT('Ctrl Pts',(-0.447578445076942,-0.350409305095673,
5.37));
#46851=CARTESIAN_POINT('Ctrl Pts',(-0.404809013009071,-0.296759939193726,
5.4));
#46852=CARTESIAN_POINT('Ctrl Pts',(-0.404809013009071,-0.296759939193726,
5.37));
#46853=CARTESIAN_POINT('Ctrl Pts',(-0.338403716683388,-0.296759939193726,
5.4));
#46854=CARTESIAN_POINT('Ctrl Pts',(-0.338403716683388,-0.296759939193726,
5.37));
#46855=CARTESIAN_POINT('',(-0.447578445076942,-0.350409305095673,5.4));
#46856=CARTESIAN_POINT('Ctrl Pts',(-0.447578445076942,-0.350409305095673,
5.4));
#46857=CARTESIAN_POINT('Ctrl Pts',(-0.404809013009071,-0.296759939193726,
5.4));
#46858=CARTESIAN_POINT('Ctrl Pts',(-0.338403716683388,-0.296759939193726,
5.4));
#46859=CARTESIAN_POINT('',(-0.447578445076942,-0.350409305095673,5.37));
#46860=CARTESIAN_POINT('',(-0.447578445076942,-0.350409305095673,5.4));
#46861=CARTESIAN_POINT('Ctrl Pts',(-0.447578445076942,-0.350409305095673,
5.37));
#46862=CARTESIAN_POINT('Ctrl Pts',(-0.404809013009071,-0.296759939193726,
5.37));
#46863=CARTESIAN_POINT('Ctrl Pts',(-0.338403716683388,-0.296759939193726,
5.37));
#46864=CARTESIAN_POINT('Origin',(-0.447578445076942,-0.154195165634155,
5.4));
#46865=CARTESIAN_POINT('',(-0.447578445076942,-0.154195165634155,5.4));
#46866=CARTESIAN_POINT('',(-0.447578445076942,-0.0770975828170776,5.4));
#46867=CARTESIAN_POINT('',(-0.447578445076942,-0.154195165634155,5.37));
#46868=CARTESIAN_POINT('',(-0.447578445076942,-0.154195165634155,5.4));
#46869=CARTESIAN_POINT('',(-0.447578445076942,-0.154195165634155,5.37));
#46870=CARTESIAN_POINT('Origin',(-0.515109077095985,-0.154195165634155,
5.4));
#46871=CARTESIAN_POINT('',(-0.515109077095985,-0.154195165634155,5.4));
#46872=CARTESIAN_POINT('',(-0.257554538547993,-0.154195165634155,5.4));
#46873=CARTESIAN_POINT('',(-0.515109077095985,-0.154195165634155,5.37));
#46874=CARTESIAN_POINT('',(-0.515109077095985,-0.154195165634155,5.4));
#46875=CARTESIAN_POINT('',(-0.515109077095985,-0.154195165634155,5.37));
#46876=CARTESIAN_POINT('Origin',(-0.515109077095985,-0.704195177555084,
5.4));
#46877=CARTESIAN_POINT('',(-0.515109077095985,-0.704195177555084,5.4));
#46878=CARTESIAN_POINT('',(-0.515109077095985,-0.352097588777542,5.4));
#46879=CARTESIAN_POINT('',(-0.515109077095985,-0.704195177555084,5.37));
#46880=CARTESIAN_POINT('',(-0.515109077095985,-0.704195177555084,5.4));
#46881=CARTESIAN_POINT('',(-0.515109077095985,-0.704195177555084,5.37));
#46882=CARTESIAN_POINT('Origin',(-0.452455773949623,-0.704195177555084,
5.4));
#46883=CARTESIAN_POINT('',(-0.452455773949623,-0.704195177555084,5.4));
#46884=CARTESIAN_POINT('',(-0.226227886974812,-0.704195177555084,5.4));
#46885=CARTESIAN_POINT('',(-0.452455773949623,-0.704195177555084,5.37));
#46886=CARTESIAN_POINT('',(-0.452455773949623,-0.704195177555084,5.4));
#46887=CARTESIAN_POINT('',(-0.452455773949623,-0.704195177555084,5.37));
#46888=CARTESIAN_POINT('Origin',(-0.452455773949623,-0.654297506809235,
5.4));
#46889=CARTESIAN_POINT('',(-0.452455773949623,-0.654297506809235,5.4));
#46890=CARTESIAN_POINT('',(-0.452455773949623,-0.327148753404617,5.4));
#46891=CARTESIAN_POINT('',(-0.452455773949623,-0.654297506809235,5.37));
#46892=CARTESIAN_POINT('',(-0.452455773949623,-0.654297506809235,5.4));
#46893=CARTESIAN_POINT('',(-0.452455773949623,-0.654297506809235,5.37));
#46894=CARTESIAN_POINT('Ctrl Pts',(-0.341780439019203,-0.713199293613434,
5.4));
#46895=CARTESIAN_POINT('Ctrl Pts',(-0.341780439019203,-0.713199293613434,
5.37));
#46896=CARTESIAN_POINT('Ctrl Pts',(-0.412312522530556,-0.713199293613434,
5.4));
#46897=CARTESIAN_POINT('Ctrl Pts',(-0.412312522530556,-0.713199293613434,
5.37));
#46898=CARTESIAN_POINT('Ctrl Pts',(-0.452455773949623,-0.654297506809235,
5.4));
#46899=CARTESIAN_POINT('Ctrl Pts',(-0.452455773949623,-0.654297506809235,
5.37));
#46900=CARTESIAN_POINT('Ctrl Pts',(-0.341780439019203,-0.713199293613434,
5.4));
#46901=CARTESIAN_POINT('Ctrl Pts',(-0.412312522530556,-0.713199293613434,
5.4));
#46902=CARTESIAN_POINT('Ctrl Pts',(-0.452455773949623,-0.654297506809235,
5.4));
#46903=CARTESIAN_POINT('Ctrl Pts',(-0.341780439019203,-0.713199293613434,
5.37));
#46904=CARTESIAN_POINT('Ctrl Pts',(-0.412312522530556,-0.713199293613434,
5.37));
#46905=CARTESIAN_POINT('Ctrl Pts',(-0.452455773949623,-0.654297506809235,
5.37));
#46906=CARTESIAN_POINT('Origin',(-0.342343106865883,-0.433697229623795,
5.37));
#46907=CARTESIAN_POINT('Ctrl Pts',(0.417940124869347,-0.416814541816711,
5.4));
#46908=CARTESIAN_POINT('Ctrl Pts',(0.417940124869347,-0.416814541816711,
5.37));
#46909=CARTESIAN_POINT('Ctrl Pts',(0.40668486058712,-0.452830946445465,
5.4));
#46910=CARTESIAN_POINT('Ctrl Pts',(0.40668486058712,-0.452830946445465,
5.37));
#46911=CARTESIAN_POINT('Ctrl Pts',(0.40668486058712,-0.495600378513336,
5.4));
#46912=CARTESIAN_POINT('Ctrl Pts',(0.40668486058712,-0.495600378513336,
5.37));
#46913=CARTESIAN_POINT('',(0.417940124869347,-0.416814541816711,5.4));
#46914=CARTESIAN_POINT('',(0.40668486058712,-0.495600378513336,5.4));
#46915=CARTESIAN_POINT('Ctrl Pts',(0.417940124869347,-0.416814541816711,
5.4));
#46916=CARTESIAN_POINT('Ctrl Pts',(0.40668486058712,-0.452830946445465,
5.4));
#46917=CARTESIAN_POINT('Ctrl Pts',(0.40668486058712,-0.495600378513336,
5.4));
#46918=CARTESIAN_POINT('',(0.417940124869347,-0.416814541816711,5.37));
#46919=CARTESIAN_POINT('',(0.417940124869347,-0.416814541816711,5.4));
#46920=CARTESIAN_POINT('',(0.40668486058712,-0.495600378513336,5.37));
#46921=CARTESIAN_POINT('Ctrl Pts',(0.417940124869347,-0.416814541816711,
5.37));
#46922=CARTESIAN_POINT('Ctrl Pts',(0.40668486058712,-0.452830946445465,
5.37));
#46923=CARTESIAN_POINT('Ctrl Pts',(0.40668486058712,-0.495600378513336,
5.37));
#46924=CARTESIAN_POINT('',(0.40668486058712,-0.495600378513336,5.4));
#46925=CARTESIAN_POINT('Ctrl Pts',(0.443076357245445,-0.379860198497772,
5.4));
#46926=CARTESIAN_POINT('Ctrl Pts',(0.443076357245445,-0.379860198497772,
5.37));
#46927=CARTESIAN_POINT('Ctrl Pts',(0.425443395972252,-0.393178796768188,
5.4));
#46928=CARTESIAN_POINT('Ctrl Pts',(0.425443395972252,-0.393178796768188,
5.37));
#46929=CARTESIAN_POINT('Ctrl Pts',(0.417940124869347,-0.416814541816711,
5.4));
#46930=CARTESIAN_POINT('Ctrl Pts',(0.417940124869347,-0.416814541816711,
5.37));
#46931=CARTESIAN_POINT('',(0.443076357245445,-0.379860198497772,5.4));
#46932=CARTESIAN_POINT('Ctrl Pts',(0.443076357245445,-0.379860198497772,
5.4));
#46933=CARTESIAN_POINT('Ctrl Pts',(0.425443395972252,-0.393178796768188,
5.4));
#46934=CARTESIAN_POINT('Ctrl Pts',(0.417940124869347,-0.416814541816711,
5.4));
#46935=CARTESIAN_POINT('',(0.443076357245445,-0.379860198497772,5.37));
#46936=CARTESIAN_POINT('',(0.443076357245445,-0.379860198497772,5.4));
#46937=CARTESIAN_POINT('Ctrl Pts',(0.443076357245445,-0.379860198497772,
5.37));
#46938=CARTESIAN_POINT('Ctrl Pts',(0.425443395972252,-0.393178796768188,
5.37));
#46939=CARTESIAN_POINT('Ctrl Pts',(0.417940124869347,-0.416814541816711,
5.37));
#46940=CARTESIAN_POINT('Ctrl Pts',(0.482844337821007,-0.366541659832001,
5.4));
#46941=CARTESIAN_POINT('Ctrl Pts',(0.482844337821007,-0.366541659832001,
5.37));
#46942=CARTESIAN_POINT('Ctrl Pts',(0.460709556937218,-0.366541659832001,
5.4));
#46943=CARTESIAN_POINT('Ctrl Pts',(0.460709556937218,-0.366541659832001,
5.37));
#46944=CARTESIAN_POINT('Ctrl Pts',(0.443076357245445,-0.379860198497772,
5.4));
#46945=CARTESIAN_POINT('Ctrl Pts',(0.443076357245445,-0.379860198497772,
5.37));
#46946=CARTESIAN_POINT('',(0.482844337821007,-0.366541659832001,5.4));
#46947=CARTESIAN_POINT('Ctrl Pts',(0.482844337821007,-0.366541659832001,
5.4));
#46948=CARTESIAN_POINT('Ctrl Pts',(0.460709556937218,-0.366541659832001,
5.4));
#46949=CARTESIAN_POINT('Ctrl Pts',(0.443076357245445,-0.379860198497772,
5.4));
#46950=CARTESIAN_POINT('',(0.482844337821007,-0.366541659832001,5.37));
#46951=CARTESIAN_POINT('',(0.482844337821007,-0.366541659832001,5.4));
#46952=CARTESIAN_POINT('Ctrl Pts',(0.482844337821007,-0.366541659832001,
5.37));
#46953=CARTESIAN_POINT('Ctrl Pts',(0.460709556937218,-0.366541659832001,
5.37));
#46954=CARTESIAN_POINT('Ctrl Pts',(0.443076357245445,-0.379860198497772,
5.37));
#46955=CARTESIAN_POINT('Ctrl Pts',(0.53236697614193,-0.381173288822174,
5.4));
#46956=CARTESIAN_POINT('Ctrl Pts',(0.53236697614193,-0.381173288822174,
5.37));
#46957=CARTESIAN_POINT('Ctrl Pts',(0.507605776190758,-0.366541659832001,
5.4));
#46958=CARTESIAN_POINT('Ctrl Pts',(0.507605776190758,-0.366541659832001,
5.37));
#46959=CARTESIAN_POINT('Ctrl Pts',(0.482844337821007,-0.366541659832001,
5.4));
#46960=CARTESIAN_POINT('Ctrl Pts',(0.482844337821007,-0.366541659832001,
5.37));
#46961=CARTESIAN_POINT('',(0.53236697614193,-0.381173288822174,5.4));
#46962=CARTESIAN_POINT('Ctrl Pts',(0.53236697614193,-0.381173288822174,
5.4));
#46963=CARTESIAN_POINT('Ctrl Pts',(0.507605776190758,-0.366541659832001,
5.4));
#46964=CARTESIAN_POINT('Ctrl Pts',(0.482844337821007,-0.366541659832001,
5.4));
#46965=CARTESIAN_POINT('',(0.53236697614193,-0.381173288822174,5.37));
#46966=CARTESIAN_POINT('',(0.53236697614193,-0.381173288822174,5.4));
#46967=CARTESIAN_POINT('Ctrl Pts',(0.53236697614193,-0.381173288822174,
5.37));
#46968=CARTESIAN_POINT('Ctrl Pts',(0.507605776190758,-0.366541659832001,
5.37));
#46969=CARTESIAN_POINT('Ctrl Pts',(0.482844337821007,-0.366541659832001,
5.37));
#46970=CARTESIAN_POINT('Origin',(0.555627569556236,-0.318519866466522,5.4));
#46971=CARTESIAN_POINT('',(0.555627569556236,-0.318519866466522,5.4));
#46972=CARTESIAN_POINT('',(0.573938477534482,-0.269198637603509,5.4));
#46973=CARTESIAN_POINT('',(0.555627569556236,-0.318519866466522,5.37));
#46974=CARTESIAN_POINT('',(0.555627569556236,-0.318519866466522,5.4));
#46975=CARTESIAN_POINT('',(0.555627569556236,-0.318519866466522,5.37));
#46976=CARTESIAN_POINT('Ctrl Pts',(0.486221060156822,-0.29675999879837,
5.4));
#46977=CARTESIAN_POINT('Ctrl Pts',(0.486221060156822,-0.29675999879837,
5.37));
#46978=CARTESIAN_POINT('Ctrl Pts',(0.52036140859127,-0.29675999879837,5.4));
#46979=CARTESIAN_POINT('Ctrl Pts',(0.52036140859127,-0.29675999879837,5.37));
#46980=CARTESIAN_POINT('Ctrl Pts',(0.555627569556236,-0.318519866466522,
5.4));
#46981=CARTESIAN_POINT('Ctrl Pts',(0.555627569556236,-0.318519866466522,
5.37));
#46982=CARTESIAN_POINT('',(0.486221060156822,-0.29675999879837,5.4));
#46983=CARTESIAN_POINT('Ctrl Pts',(0.486221060156822,-0.29675999879837,
5.4));
#46984=CARTESIAN_POINT('Ctrl Pts',(0.52036140859127,-0.29675999879837,5.4));
#46985=CARTESIAN_POINT('Ctrl Pts',(0.555627569556236,-0.318519866466522,
5.4));
#46986=CARTESIAN_POINT('',(0.486221060156822,-0.29675999879837,5.37));
#46987=CARTESIAN_POINT('',(0.486221060156822,-0.29675999879837,5.4));
#46988=CARTESIAN_POINT('Ctrl Pts',(0.486221060156822,-0.29675999879837,
5.37));
#46989=CARTESIAN_POINT('Ctrl Pts',(0.52036140859127,-0.29675999879837,5.37));
#46990=CARTESIAN_POINT('Ctrl Pts',(0.555627569556236,-0.318519866466522,
5.37));
#46991=CARTESIAN_POINT('Ctrl Pts',(0.442888721823692,-0.310266053676605,
5.4));
#46992=CARTESIAN_POINT('Ctrl Pts',(0.442888721823692,-0.310266053676605,
5.37));
#46993=CARTESIAN_POINT('Ctrl Pts',(0.462585434317589,-0.29675999879837,
5.4));
#46994=CARTESIAN_POINT('Ctrl Pts',(0.462585434317589,-0.29675999879837,
5.37));
#46995=CARTESIAN_POINT('Ctrl Pts',(0.486221060156822,-0.29675999879837,
5.4));
#46996=CARTESIAN_POINT('Ctrl Pts',(0.486221060156822,-0.29675999879837,
5.37));
#46997=CARTESIAN_POINT('',(0.442888721823692,-0.310266053676605,5.4));
#46998=CARTESIAN_POINT('Ctrl Pts',(0.442888721823692,-0.310266053676605,
5.4));
#46999=CARTESIAN_POINT('Ctrl Pts',(0.462585434317589,-0.29675999879837,
5.4));
#47000=CARTESIAN_POINT('Ctrl Pts',(0.486221060156822,-0.29675999879837,
5.4));
#47001=CARTESIAN_POINT('',(0.442888721823692,-0.310266053676605,5.37));
#47002=CARTESIAN_POINT('',(0.442888721823692,-0.310266053676605,5.4));
#47003=CARTESIAN_POINT('Ctrl Pts',(0.442888721823692,-0.310266053676605,
5.37));
#47004=CARTESIAN_POINT('Ctrl Pts',(0.462585434317589,-0.29675999879837,
5.37));
#47005=CARTESIAN_POINT('Ctrl Pts',(0.486221060156822,-0.29675999879837,
5.37));
#47006=CARTESIAN_POINT('Ctrl Pts',(0.399931892752647,-0.366166508197784,
5.4));
#47007=CARTESIAN_POINT('Ctrl Pts',(0.399931892752647,-0.366166508197784,
5.37));
#47008=CARTESIAN_POINT('Ctrl Pts',(0.423192486166954,-0.32377222776413,
5.4));
#47009=CARTESIAN_POINT('Ctrl Pts',(0.423192486166954,-0.32377222776413,
5.37));
#47010=CARTESIAN_POINT('Ctrl Pts',(0.442888721823692,-0.310266053676605,
5.4));
#47011=CARTESIAN_POINT('Ctrl Pts',(0.442888721823692,-0.310266053676605,
5.37));
#47012=CARTESIAN_POINT('',(0.399931892752647,-0.366166508197784,5.4));
#47013=CARTESIAN_POINT('Ctrl Pts',(0.399931892752647,-0.366166508197784,
5.4));
#47014=CARTESIAN_POINT('Ctrl Pts',(0.423192486166954,-0.32377222776413,
5.4));
#47015=CARTESIAN_POINT('Ctrl Pts',(0.442888721823692,-0.310266053676605,
5.4));
#47016=CARTESIAN_POINT('',(0.399931892752647,-0.366166508197784,5.37));
#47017=CARTESIAN_POINT('',(0.399931892752647,-0.366166508197784,5.4));
#47018=CARTESIAN_POINT('Ctrl Pts',(0.399931892752647,-0.366166508197784,
5.37));
#47019=CARTESIAN_POINT('Ctrl Pts',(0.423192486166954,-0.32377222776413,
5.37));
#47020=CARTESIAN_POINT('Ctrl Pts',(0.442888721823692,-0.310266053676605,
5.37));
#47021=CARTESIAN_POINT('Origin',(0.399931892752647,-0.305764055252075,5.4));
#47022=CARTESIAN_POINT('',(0.399931892752647,-0.305764055252075,5.4));
#47023=CARTESIAN_POINT('',(0.399931892752647,-0.152882027626038,5.4));
#47024=CARTESIAN_POINT('',(0.399931892752647,-0.305764055252075,5.37));
#47025=CARTESIAN_POINT('',(0.399931892752647,-0.305764055252075,5.4));
#47026=CARTESIAN_POINT('',(0.399931892752647,-0.305764055252075,5.37));
#47027=CARTESIAN_POINT('Origin',(0.339154228568077,-0.305764055252075,5.4));
#47028=CARTESIAN_POINT('',(0.339154228568077,-0.305764055252075,5.4));
#47029=CARTESIAN_POINT('',(0.169577114284039,-0.305764055252075,5.4));
#47030=CARTESIAN_POINT('',(0.339154228568077,-0.305764055252075,5.37));
#47031=CARTESIAN_POINT('',(0.339154228568077,-0.305764055252075,5.4));
#47032=CARTESIAN_POINT('',(0.339154228568077,-0.305764055252075,5.37));
#47033=CARTESIAN_POINT('Origin',(0.339154228568077,-0.704195177555084,5.4));
#47034=CARTESIAN_POINT('',(0.339154228568077,-0.704195177555084,5.4));
#47035=CARTESIAN_POINT('',(0.339154228568077,-0.352097588777542,5.4));
#47036=CARTESIAN_POINT('',(0.339154228568077,-0.704195177555084,5.37));
#47037=CARTESIAN_POINT('',(0.339154228568077,-0.704195177555084,5.4));
#47038=CARTESIAN_POINT('',(0.339154228568077,-0.704195177555084,5.37));
#47039=CARTESIAN_POINT('Origin',(0.40668486058712,-0.704195177555084,5.4));
#47040=CARTESIAN_POINT('',(0.40668486058712,-0.704195177555084,5.4));
#47041=CARTESIAN_POINT('',(0.20334243029356,-0.704195177555084,5.4));
#47042=CARTESIAN_POINT('',(0.40668486058712,-0.704195177555084,5.37));
#47043=CARTESIAN_POINT('',(0.40668486058712,-0.704195177555084,5.4));
#47044=CARTESIAN_POINT('',(0.40668486058712,-0.704195177555084,5.37));
#47045=CARTESIAN_POINT('Origin',(0.40668486058712,-0.495600378513336,5.4));
#47046=CARTESIAN_POINT('',(0.40668486058712,-0.247800189256668,5.4));
#47047=CARTESIAN_POINT('',(0.40668486058712,-0.495600378513336,5.37));
#47048=CARTESIAN_POINT('Origin',(0.447390899062157,-0.500477588176727,5.37));
#47049=CARTESIAN_POINT('Origin',(0.,0.,5.4));
#47050=CARTESIAN_POINT('Origin',(0.,0.,5.4));
#47051=CARTESIAN_POINT('Origin',(0.,0.,5.4));
#47052=CARTESIAN_POINT('Origin',(0.,0.,5.4));
#47053=CARTESIAN_POINT('Origin',(0.,0.,5.4));
#47054=CARTESIAN_POINT('Origin',(0.,0.,5.4));
#47055=CARTESIAN_POINT('Origin',(0.,4.8,3.135));
#47056=CARTESIAN_POINT('',(-0.3,4.8,2.4));
#47057=CARTESIAN_POINT('Origin',(0.,4.8,2.4));
#47058=CARTESIAN_POINT('',(-0.3,4.8,3.5));
#47059=CARTESIAN_POINT('',(-0.3,4.8,3.135));
#47060=CARTESIAN_POINT('',(-1.32689352189158E-17,4.5,3.4));
#47061=CARTESIAN_POINT('Ctrl Pts',(3.46944695195361E-17,4.5,3.4));
#47062=CARTESIAN_POINT('Ctrl Pts',(-0.0387350904599242,4.5,3.4));
#47063=CARTESIAN_POINT('Ctrl Pts',(-0.079391136615057,4.50794962800524,
3.40489262537173));
#47064=CARTESIAN_POINT('Ctrl Pts',(-0.153059740759081,4.53890790426334,
3.42249923688317));
#47065=CARTESIAN_POINT('Ctrl Pts',(-0.186131887156364,4.56186781844444,
3.43504912069967));
#47066=CARTESIAN_POINT('Ctrl Pts',(-0.238301026739628,4.6140369580277,3.4594914730493));
#47067=CARTESIAN_POINT('Ctrl Pts',(-0.261143371678758,4.64706258429155,
3.47321311494003));
#47068=CARTESIAN_POINT('Ctrl Pts',(-0.291998110979302,4.7204841942567,3.49369955460524));
#47069=CARTESIAN_POINT('Ctrl Pts',(-0.3,4.76101336352273,3.5));
#47070=CARTESIAN_POINT('Ctrl Pts',(-0.3,4.8,3.5));
#47071=CARTESIAN_POINT('',(0.3,4.8,3.5));
#47072=CARTESIAN_POINT('Ctrl Pts',(0.3,4.8,3.5));
#47073=CARTESIAN_POINT('Ctrl Pts',(0.3,4.76101336352273,3.5));
#47074=CARTESIAN_POINT('Ctrl Pts',(0.291998110979302,4.7204841942567,3.49369955460524));
#47075=CARTESIAN_POINT('Ctrl Pts',(0.261143371678758,4.64706258429155,3.47321311494003));
#47076=CARTESIAN_POINT('Ctrl Pts',(0.238301026739628,4.6140369580277,3.4594914730493));
#47077=CARTESIAN_POINT('Ctrl Pts',(0.186131887156364,4.56186781844444,3.43504912069967));
#47078=CARTESIAN_POINT('Ctrl Pts',(0.153059740759081,4.53890790426334,3.42249923688317));
#47079=CARTESIAN_POINT('Ctrl Pts',(0.0793911366150571,4.50794962800524,
3.40489262537173));
#47080=CARTESIAN_POINT('Ctrl Pts',(0.0387350904599242,4.5,3.4));
#47081=CARTESIAN_POINT('Ctrl Pts',(-6.24500451351651E-17,4.5,3.4));
#47082=CARTESIAN_POINT('',(-3.75550638825911E-17,5.1,3.4));
#47083=CARTESIAN_POINT('Ctrl Pts',(-4.16333634234434E-17,5.1,3.4));
#47084=CARTESIAN_POINT('Ctrl Pts',(0.0387350904599243,5.1,3.4));
#47085=CARTESIAN_POINT('Ctrl Pts',(0.079391136615057,5.09205037199476,3.40489262537173));
#47086=CARTESIAN_POINT('Ctrl Pts',(0.15305974075908,5.06109209573666,3.42249923688317));
#47087=CARTESIAN_POINT('Ctrl Pts',(0.186131887156364,5.03813218155556,3.43504912069967));
#47088=CARTESIAN_POINT('Ctrl Pts',(0.238301026739628,4.9859630419723,3.4594914730493));
#47089=CARTESIAN_POINT('Ctrl Pts',(0.261143371678758,4.95293741570845,3.47321311494003));
#47090=CARTESIAN_POINT('Ctrl Pts',(0.291998110979302,4.8795158057433,3.49369955460524));
#47091=CARTESIAN_POINT('Ctrl Pts',(0.3,4.83898663647727,3.5));
#47092=CARTESIAN_POINT('Ctrl Pts',(0.3,4.8,3.5));
#47093=CARTESIAN_POINT('Ctrl Pts',(-0.3,4.8,3.5));
#47094=CARTESIAN_POINT('Ctrl Pts',(-0.3,4.83898663647727,3.5));
#47095=CARTESIAN_POINT('Ctrl Pts',(-0.291998110979302,4.8795158057433,3.49369955460524));
#47096=CARTESIAN_POINT('Ctrl Pts',(-0.261143371678758,4.95293741570845,
3.47321311494003));
#47097=CARTESIAN_POINT('Ctrl Pts',(-0.238301026739628,4.9859630419723,3.4594914730493));
#47098=CARTESIAN_POINT('Ctrl Pts',(-0.186131887156364,5.03813218155556,
3.43504912069967));
#47099=CARTESIAN_POINT('Ctrl Pts',(-0.153059740759081,5.06109209573666,
3.42249923688317));
#47100=CARTESIAN_POINT('Ctrl Pts',(-0.0793911366150575,5.09205037199476,
3.40489262537173));
#47101=CARTESIAN_POINT('Ctrl Pts',(-0.0387350904599243,5.1,3.4));
#47102=CARTESIAN_POINT('Ctrl Pts',(-1.38777878078145E-17,5.1,3.4));
#47103=CARTESIAN_POINT('Origin',(0.,6.76,3.9));
#47104=CARTESIAN_POINT('',(-1.12434822629719E-16,6.8,2.9819));
#47105=CARTESIAN_POINT('Origin',(0.,6.8,3.9));
#47106=CARTESIAN_POINT('',(1.0263764823654E-16,6.72,3.0619));
#47107=CARTESIAN_POINT('',(-1.07536235433129E-16,6.76,3.0219));
#47108=CARTESIAN_POINT('Origin',(0.,6.72,3.9));
#47109=CARTESIAN_POINT('Origin',(0.,6.115,3.9));
#47110=CARTESIAN_POINT('',(-1.0263764823654E-16,5.4,3.0619));
#47111=CARTESIAN_POINT('Origin',(0.,5.4,3.9));
#47112=CARTESIAN_POINT('',(-1.0263764823654E-16,6.115,3.0619));
#47113=CARTESIAN_POINT('Origin',(0.,6.8,3.9));
#47114=CARTESIAN_POINT('',(-1.66132477258362,6.8,4.7));
#47115=CARTESIAN_POINT('',(-1.66132477258362,6.8,2.6));
#47116=CARTESIAN_POINT('',(-1.66132477258362,6.8,3.925));
#47117=CARTESIAN_POINT('',(1.66132477258362,6.8,4.7));
#47118=CARTESIAN_POINT('Ctrl Pts',(1.66132477258362,6.8,4.7));
#47119=CARTESIAN_POINT('Ctrl Pts',(1.66132477258362,6.8,4.72938558803469));
#47120=CARTESIAN_POINT('Ctrl Pts',(1.65134477996489,6.8,4.76320656017475));
#47121=CARTESIAN_POINT('Ctrl Pts',(1.61541194091876,6.8,4.82883847656767));
#47122=CARTESIAN_POINT('Ctrl Pts',(1.57674832389957,6.8,4.86728708168208));
#47123=CARTESIAN_POINT('Ctrl Pts',(1.47030882164508,6.8,4.94844516253902));
#47124=CARTESIAN_POINT('Ctrl Pts',(1.37375034243015,6.8,4.99240423873322));
#47125=CARTESIAN_POINT('Ctrl Pts',(1.19382805886623,6.8,5.05708112048866));
#47126=CARTESIAN_POINT('Ctrl Pts',(1.09032757512215,6.8,5.08373727101866));
#47127=CARTESIAN_POINT('Ctrl Pts',(0.876179229724424,6.8,5.12689010427577));
#47128=CARTESIAN_POINT('Ctrl Pts',(0.765498572136393,6.8,5.14322387535846));
#47129=CARTESIAN_POINT('Ctrl Pts',(0.431232289541573,6.8,5.18054651477358));
#47130=CARTESIAN_POINT('Ctrl Pts',(0.20556454289784,6.8,5.18989794855664));
#47131=CARTESIAN_POINT('Ctrl Pts',(-0.20556454289784,6.8,5.18989794855664));
#47132=CARTESIAN_POINT('Ctrl Pts',(-0.431232289541573,6.8,5.18054651477358));
#47133=CARTESIAN_POINT('Ctrl Pts',(-0.765498572136393,6.8,5.14322387535846));
#47134=CARTESIAN_POINT('Ctrl Pts',(-0.876179229724424,6.8,5.12689010427577));
#47135=CARTESIAN_POINT('Ctrl Pts',(-1.09032757512215,6.8,5.08373727101866));
#47136=CARTESIAN_POINT('Ctrl Pts',(-1.19382805886623,6.8,5.05708112048866));
#47137=CARTESIAN_POINT('Ctrl Pts',(-1.37375034243015,6.8,4.99240423873322));
#47138=CARTESIAN_POINT('Ctrl Pts',(-1.47030882164508,6.8,4.94844516253902));
#47139=CARTESIAN_POINT('Ctrl Pts',(-1.57674832389957,6.8,4.86728708168208));
#47140=CARTESIAN_POINT('Ctrl Pts',(-1.61541194091876,6.8,4.82883847656767));
#47141=CARTESIAN_POINT('Ctrl Pts',(-1.65134477996489,6.8,4.76320656017475));
#47142=CARTESIAN_POINT('Ctrl Pts',(-1.66132477258362,6.8,4.7293855880347));
#47143=CARTESIAN_POINT('Ctrl Pts',(-1.66132477258362,6.8,4.7));
#47144=CARTESIAN_POINT('',(1.66132477258362,6.8,2.6));
#47145=CARTESIAN_POINT('',(1.66132477258362,6.8,3.925));
#47146=CARTESIAN_POINT('',(-1.7,6.8,2.6));
#47147=CARTESIAN_POINT('Origin',(0.,4.24978484524311,3.9));
#47148=CARTESIAN_POINT('',(0.,4.09956969048622,3.9));
#47149=CARTESIAN_POINT('',(-6.12323399573677E-17,4.4,3.4));
#47150=CARTESIAN_POINT('',(-3.06161699786839E-17,4.24978484524311,3.65));
#47151=CARTESIAN_POINT('Origin',(0.,4.4,3.9));
#47152=CARTESIAN_POINT('Origin',(0.,4.9,3.9));
#47153=CARTESIAN_POINT('',(-6.12323399573677E-17,4.9,3.4));
#47154=CARTESIAN_POINT('',(-6.12323399573677E-17,5.4,3.4));
#47155=CARTESIAN_POINT('',(-6.12323399573677E-17,4.9,3.4));
#47156=CARTESIAN_POINT('Origin',(0.,5.4,3.9));
#47157=CARTESIAN_POINT('Origin',(0.,5.4,4.7381));
#47158=CARTESIAN_POINT('Origin',(1.7,6.8,2.6));
#47159=CARTESIAN_POINT('Origin',(0.,0.,2.6));
#47160=CARTESIAN_POINT('Origin',(0.,0.,3.925));
#47161=CARTESIAN_POINT('',(-7.,-8.57252759403147E-16,4.7));
#47162=CARTESIAN_POINT('Origin',(0.,0.,4.7));
#47163=CARTESIAN_POINT('',(-7.,-8.57252759403147E-16,2.45));
#47164=CARTESIAN_POINT('',(-7.,-8.57252759403147E-16,3.925));
#47165=CARTESIAN_POINT('Origin',(0.,0.,2.45));
#47166=CARTESIAN_POINT('Origin',(0.,0.,4.7));
#47167=CARTESIAN_POINT('Origin',(0.,0.,4.7));
#47168=CARTESIAN_POINT('',(-6.3,-7.71527483462833E-16,5.4));
#47169=CARTESIAN_POINT('Origin',(0.,0.,5.4));
#47170=CARTESIAN_POINT('Origin',(-6.3,-7.71527483462833E-16,4.7));
#47171=CARTESIAN_POINT('Origin',(6.,0.,2.425));
#47172=CARTESIAN_POINT('',(5.545,5.57214293612045E-17,2.4));
#47173=CARTESIAN_POINT('Origin',(6.,0.,2.4));
#47174=CARTESIAN_POINT('',(5.595,-4.95981953654677E-17,2.45));
#47175=CARTESIAN_POINT('',(5.57,5.26598123633361E-17,2.425));
#47176=CARTESIAN_POINT('Origin',(6.,0.,2.45));
#47177=CARTESIAN_POINT('Origin',(6.95,0.,2.4));
#47178=CARTESIAN_POINT('',(-6.95,-8.5112952540741E-16,2.4));
#47179=CARTESIAN_POINT('Origin',(0.,0.,2.4));
#47180=CARTESIAN_POINT('',(-3.455,5.19615242270663,2.4));
#47181=CARTESIAN_POINT('Origin',(-3.,5.19615242270663,2.4));
#47182=CARTESIAN_POINT('',(-3.455,-5.19615242270663,2.4));
#47183=CARTESIAN_POINT('Origin',(-3.,-5.19615242270663,2.4));
#47184=CARTESIAN_POINT('',(2.66,-3.25756048573196E-16,2.4));
#47185=CARTESIAN_POINT('Origin',(0.,0.,2.4));
#47186=CARTESIAN_POINT('',(2.545,-5.19615242270663,2.4));
#47187=CARTESIAN_POINT('Origin',(3.,-5.19615242270663,2.4));
#47188=CARTESIAN_POINT('',(-6.455,7.90509508849616E-16,2.4));
#47189=CARTESIAN_POINT('Origin',(-6.,7.34788079488412E-16,2.4));
#47190=CARTESIAN_POINT('',(2.545,5.19615242270663,2.4));
#47191=CARTESIAN_POINT('Origin',(3.,5.19615242270663,2.4));
#47192=CARTESIAN_POINT('Origin',(6.,0.,3.385));
#47193=CARTESIAN_POINT('',(5.595,-4.95981953654677E-17,4.4));
#47194=CARTESIAN_POINT('',(5.595,-4.95981953654677E-17,3.385));
#47195=CARTESIAN_POINT('Origin',(6.,0.,4.4));
#47196=CARTESIAN_POINT('Origin',(3.,5.19615242270663,2.425));
#47197=CARTESIAN_POINT('',(2.595,5.19615242270663,2.45));
#47198=CARTESIAN_POINT('',(2.57,5.19615242270663,2.425));
#47199=CARTESIAN_POINT('Origin',(3.,5.19615242270663,2.45));
#47200=CARTESIAN_POINT('Origin',(3.,5.19615242270663,3.385));
#47201=CARTESIAN_POINT('',(2.595,5.19615242270663,4.4));
#47202=CARTESIAN_POINT('',(2.595,5.19615242270663,3.385));
#47203=CARTESIAN_POINT('Origin',(3.,5.19615242270663,4.4));
#47204=CARTESIAN_POINT('Origin',(-3.,5.19615242270663,2.425));
#47205=CARTESIAN_POINT('',(-3.405,5.19615242270663,2.45));
#47206=CARTESIAN_POINT('',(-3.43,5.19615242270663,2.425));
#47207=CARTESIAN_POINT('Origin',(-3.,5.19615242270663,2.45));
#47208=CARTESIAN_POINT('Origin',(-3.,5.19615242270663,3.385));
#47209=CARTESIAN_POINT('',(-3.405,5.19615242270663,4.4));
#47210=CARTESIAN_POINT('',(-3.405,5.19615242270663,3.385));
#47211=CARTESIAN_POINT('Origin',(-3.,5.19615242270663,4.4));
#47212=CARTESIAN_POINT('Origin',(-6.,7.34788079488412E-16,2.425));
#47213=CARTESIAN_POINT('',(-6.405,6.85189884122944E-16,2.45));
#47214=CARTESIAN_POINT('',(-6.43,7.87447891851748E-16,2.425));
#47215=CARTESIAN_POINT('Origin',(-6.,7.34788079488412E-16,2.45));
#47216=CARTESIAN_POINT('Origin',(-6.,7.34788079488412E-16,3.385));
#47217=CARTESIAN_POINT('',(-6.405,6.85189884122944E-16,4.4));
#47218=CARTESIAN_POINT('',(-6.405,6.85189884122944E-16,3.385));
#47219=CARTESIAN_POINT('Origin',(-6.,7.34788079488412E-16,4.4));
#47220=CARTESIAN_POINT('Origin',(-3.,-5.19615242270663,2.425));
#47221=CARTESIAN_POINT('',(-3.405,-5.19615242270663,2.45));
#47222=CARTESIAN_POINT('',(-3.43,-5.19615242270663,2.425));
#47223=CARTESIAN_POINT('Origin',(-3.,-5.19615242270663,2.45));
#47224=CARTESIAN_POINT('Origin',(-3.,-5.19615242270663,3.385));
#47225=CARTESIAN_POINT('',(-3.405,-5.19615242270663,4.4));
#47226=CARTESIAN_POINT('',(-3.405,-5.19615242270663,3.385));
#47227=CARTESIAN_POINT('Origin',(-3.,-5.19615242270663,4.4));
#47228=CARTESIAN_POINT('Origin',(3.,-5.19615242270663,2.425));
#47229=CARTESIAN_POINT('',(2.595,-5.19615242270663,2.45));
#47230=CARTESIAN_POINT('',(2.57,-5.19615242270663,2.425));
#47231=CARTESIAN_POINT('Origin',(3.,-5.19615242270663,2.45));
#47232=CARTESIAN_POINT('Origin',(3.,-5.19615242270663,3.385));
#47233=CARTESIAN_POINT('',(2.595,-5.19615242270663,4.4));
#47234=CARTESIAN_POINT('',(2.595,-5.19615242270663,3.385));
#47235=CARTESIAN_POINT('Origin',(3.,-5.19615242270663,4.4));
#47236=CARTESIAN_POINT('Origin',(3.,-5.19615242270663,4.4));
#47237=CARTESIAN_POINT('',(3.,-5.19615242270663,4.64334855070616));
#47238=CARTESIAN_POINT('',(2.595,-5.19615242270663,4.4));
#47239=CARTESIAN_POINT('Origin',(-3.,-5.19615242270663,4.4));
#47240=CARTESIAN_POINT('',(-3.,-5.19615242270663,4.64334855070616));
#47241=CARTESIAN_POINT('',(-3.405,-5.19615242270663,4.4));
#47242=CARTESIAN_POINT('Origin',(-6.,7.34788079488412E-16,4.4));
#47243=CARTESIAN_POINT('',(-6.,7.34788079488412E-16,4.64334855070616));
#47244=CARTESIAN_POINT('',(-6.405,6.85189884122944E-16,4.4));
#47245=CARTESIAN_POINT('Origin',(-3.,5.19615242270663,4.4));
#47246=CARTESIAN_POINT('',(-3.,5.19615242270663,4.64334855070616));
#47247=CARTESIAN_POINT('',(-3.405,5.19615242270663,4.4));
#47248=CARTESIAN_POINT('Origin',(3.,5.19615242270663,4.4));
#47249=CARTESIAN_POINT('',(3.,5.19615242270663,4.64334855070616));
#47250=CARTESIAN_POINT('',(2.595,5.19615242270663,4.4));
#47251=CARTESIAN_POINT('Origin',(6.,0.,4.4));
#47252=CARTESIAN_POINT('',(6.,0.,4.64334855070616));
#47253=CARTESIAN_POINT('',(5.595,-4.95981953654677E-17,4.4));
#47254=CARTESIAN_POINT('Origin',(0.,0.,2.43));
#47255=CARTESIAN_POINT('',(2.6,3.18408167778312E-16,2.46));
#47256=CARTESIAN_POINT('',(2.63,-3.22082108175754E-16,2.43));
#47257=CARTESIAN_POINT('',(-2.6,-3.18408167778312E-16,2.46));
#47258=CARTESIAN_POINT('Origin',(0.,0.,2.46));
#47259=CARTESIAN_POINT('Origin',(0.,0.,2.46));
#47260=CARTESIAN_POINT('Origin',(0.,0.,3.1));
#47261=CARTESIAN_POINT('',(-2.6,-3.18408167778312E-16,3.8));
#47262=CARTESIAN_POINT('Origin',(0.,0.,3.8));
#47263=CARTESIAN_POINT('',(-2.6,-3.18408167778312E-16,3.1));
#47264=CARTESIAN_POINT('Origin',(0.,0.,5.4));
#47265=CARTESIAN_POINT('Origin',(0.,0.,2.425));
#47266=CARTESIAN_POINT('',(-6.975,-8.54191142405279E-16,2.425));
#47267=CARTESIAN_POINT('Origin',(2.4,0.,4.6));
#47268=CARTESIAN_POINT('',(-2.4,-2.93915231795365E-16,4.6));
#47269=CARTESIAN_POINT('Origin',(0.,0.,4.6));
#47270=CARTESIAN_POINT('Origin',(0.,0.,4.2));
#47271=CARTESIAN_POINT('',(-2.4,-2.93915231795365E-16,3.8));
#47272=CARTESIAN_POINT('',(-2.4,-2.93915231795365E-16,4.2));
#47273=CARTESIAN_POINT('Origin',(0.,0.,3.8));
#47274=CARTESIAN_POINT('Origin',(2.6,0.,3.8));
#59174=UNCERTAINTY_MEASURE_WITH_UNIT(LENGTH_MEASURE(0.001),#59205,
'DISTANCE_ACCURACY_VALUE',
'Maximum model space distance between geometric entities at asserted c
onnectivities');
#59182=UNCERTAINTY_MEASURE_WITH_UNIT(LENGTH_MEASURE(0.001),#59205,
'DISTANCE_ACCURACY_VALUE',
'Maximum model space distance between geometric entities at asserted c
onnectivities');
#59196=(
GEOMETRIC_REPRESENTATION_CONTEXT(3)
GLOBAL_UNCERTAINTY_ASSIGNED_CONTEXT((#59174))
GLOBAL_UNIT_ASSIGNED_CONTEXT((#59205,#59207,#59208))
REPRESENTATION_CONTEXT('','3D')
);
#59204=(
GEOMETRIC_REPRESENTATION_CONTEXT(3)
GLOBAL_UNCERTAINTY_ASSIGNED_CONTEXT((#59182))
GLOBAL_UNIT_ASSIGNED_CONTEXT((#59205,#59207,#59208))
REPRESENTATION_CONTEXT('','3D')
);
#59205=(
LENGTH_UNIT()
NAMED_UNIT(*)
SI_UNIT(.CENTI.,.METRE.)
);
#59207=(
NAMED_UNIT(*)
PLANE_ANGLE_UNIT()
SI_UNIT($,.RADIAN.)
);
#59208=(
NAMED_UNIT(*)
SI_UNIT($,.STERADIAN.)
SOLID_ANGLE_UNIT()
);
#59222=SHAPE_DEFINITION_REPRESENTATION(#59243,#59309);
#59243=PRODUCT_DEFINITION_SHAPE('',$,#59331);
#59309=SHAPE_REPRESENTATION('',(#23996),#59196);
#59317=PRODUCT_DEFINITION_CONTEXT('part definition',#59382,'design');
#59331=PRODUCT_DEFINITION('2026-10-23-00-48-24-882',
'03_Rear_End_Cover_D140_Bearing_Housing',#59352,#59317);
#59352=PRODUCT_DEFINITION_FORMATION('',$,#59397);
#59382=APPLICATION_CONTEXT(
'Core Data for Automotive Mechanical Design Process');
#59383=PRODUCT_CONTEXT('part definition',#59382,'mechanical');
#59397=PRODUCT('2026-10-23-00-48-24-882',
'03_Rear_End_Cover_D140_Bearing_Housing',$,(#59383));
#59580=COLOUR_RGB('Grey',0.48,0.52,0.57);
#59581=FILL_AREA_STYLE_COLOUR('',#59580);
#59582=FILL_AREA_STYLE('',(#59581));
#59583=SURFACE_STYLE_FILL_AREA(#59582);
#59584=SURFACE_SIDE_STYLE('',(#59583));
#59585=SURFACE_STYLE_USAGE(.BOTH.,#59584);
#59586=PRESENTATION_STYLE_ASSIGNMENT((#59585));
ENDSEC;
END-ISO-10303-21;
